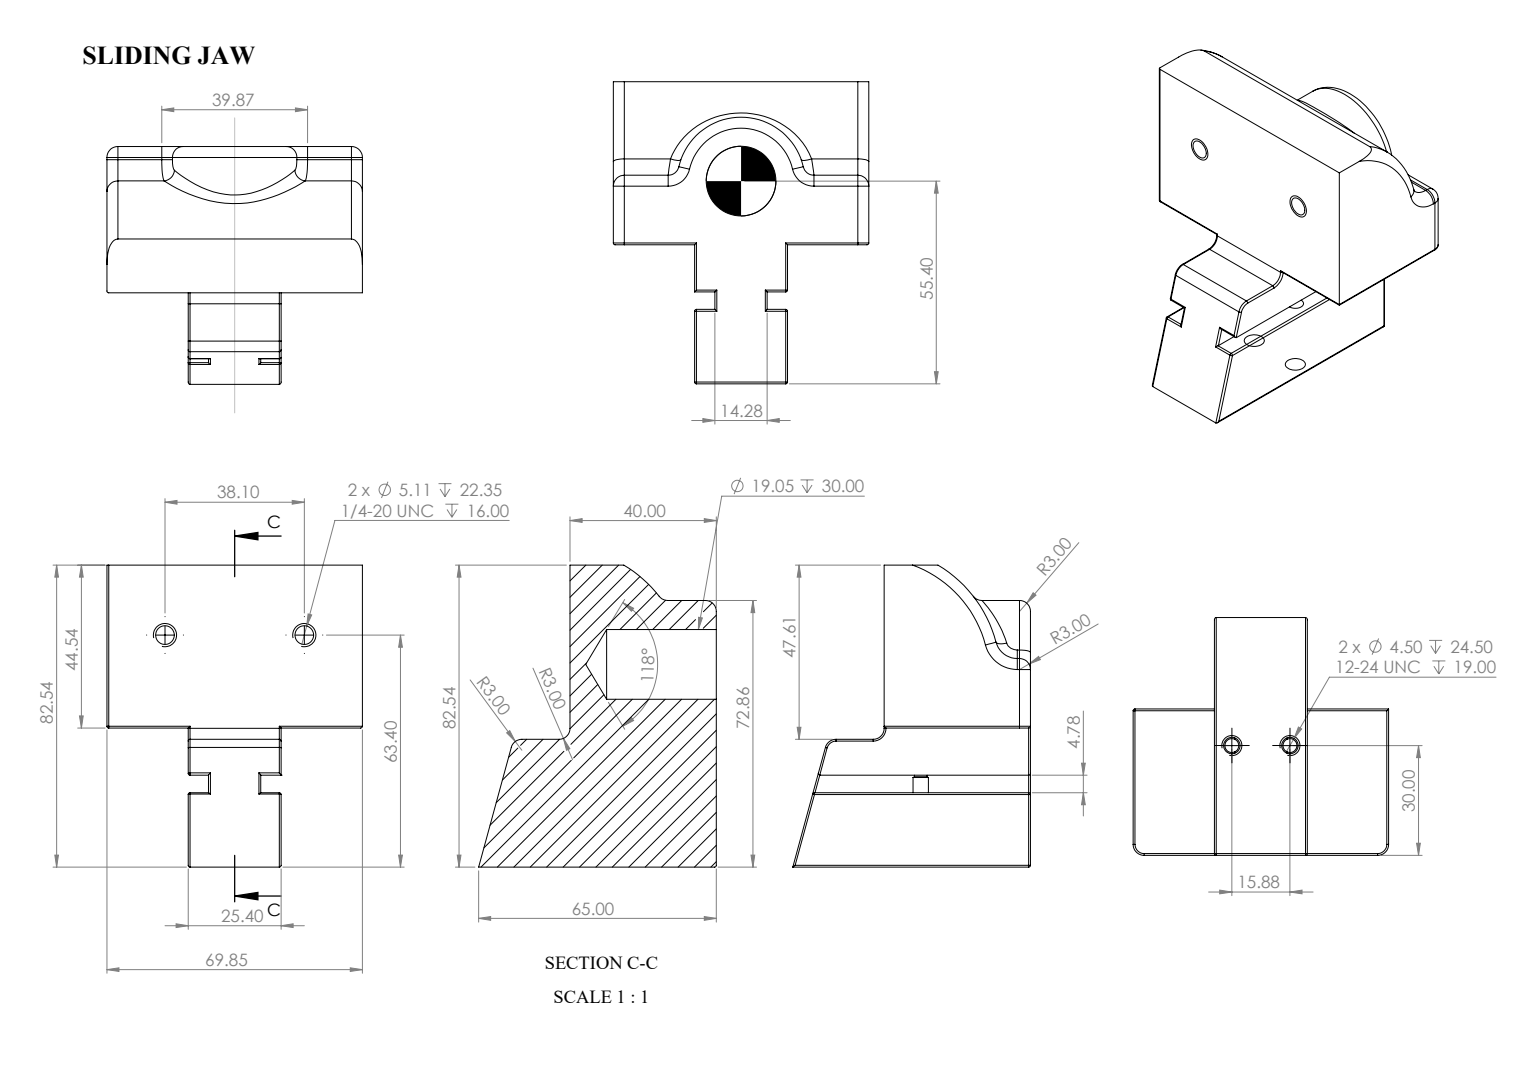
ISO-10303-21;
HEADER;
FILE_DESCRIPTION (('STEP AP214'),
    '1' );
FILE_NAME ('1.1 Sliding Jaw.step',
    '2026-10-06T08:51:13',
    ( '' ),
    ( '' ),
    'SwSTEP 2.0',
    'SolidWorks 2021',
    '' );
FILE_SCHEMA (( 'AUTOMOTIVE_DESIGN' ));
ENDSEC;

DATA;
#14=COLOUR_RGB ( '', 0.08235294, 0.09019608, 0.10196078) ;
#59=CARTESIAN_POINT ( 'NONE',  ( -12.69999999999999929, -60.26999999999998892, -39.50000000000000000 ) ) ;
#66=FILL_AREA_STYLE ('',( #56690 ) ) ;
#140=ORIENTED_EDGE ( 'NONE', *, *, #3276, .F. ) ;
#150=DIRECTION ( 'NONE',  ( 0.000000000000000000, -0.9647414015272155474, 0.2631995976047525887 ) ) ;
#175=ORIENTED_EDGE ( 'NONE', *, *, #80806, .F. ) ;
#177=EDGE_CURVE ( 'NONE', #92630, #88659, #70457, .T. ) ;
#207=ORIENTED_EDGE ( 'NONE', *, *, #61881, .T. ) ;
#237=VERTEX_POINT ( 'NONE', #52898 ) ;
#261=PRESENTATION_STYLE_ASSIGNMENT (( #47937 ) ) ;
#311=ORIENTED_EDGE ( 'NONE', *, *, #103224, .T. ) ;
#327=DIRECTION ( 'NONE',  ( -1.000000000000000000, -2.891205793294679312E-16, 0.000000000000000000 ) ) ;
#402=CARTESIAN_POINT ( 'NONE',  ( -16.92402963342697220, -0.5732982342275830812, -34.79992920313960525 ) ) ;
#422=FILL_AREA_STYLE ('',( #141288 ) ) ;
#437=EDGE_CURVE ( 'NONE', #128814, #125503, #6074, .T. ) ;
#500=EDGE_CURVE ( 'NONE', #83224, #56577, #120555, .T. ) ;
#523=CARTESIAN_POINT ( 'NONE',  ( 0.000000000000000000, -40.42999999999999261, -39.50000000000000000 ) ) ;
#561=SURFACE_STYLE_FILL_AREA ( #32509 ) ;
#640=CARTESIAN_POINT ( 'NONE',  ( 19.04500000000000881, 3.130000000000007887, -22.35000000000000142 ) ) ;
#662=ORIENTED_EDGE ( 'NONE', *, *, #138768, .T. ) ;
#675=DIRECTION ( 'NONE',  ( 1.000000000000000000, -1.248002500702738701E-15, 3.404785525682858480E-16 ) ) ;
#735=ORIENTED_EDGE ( 'NONE', *, *, #48279, .T. ) ;
#744=ORIENTED_EDGE ( 'NONE', *, *, #46623, .T. ) ;
#797=DIRECTION ( 'NONE',  ( 0.000000000000000000, 0.000000000000000000, -1.000000000000000000 ) ) ;
#818=PRESENTATION_STYLE_ASSIGNMENT (( #100864 ) ) ;
#821=ORIENTED_EDGE ( 'NONE', *, *, #120338, .F. ) ;
#853=CARTESIAN_POINT ( 'NONE',  ( 18.91358171146897860, 2.162374846302510090, -30.33482670853117114 ) ) ;
#858=STYLED_ITEM ( 'NONE', ( #106410 ), #103236 ) ;
#859=( NAMED_UNIT ( * ) SI_UNIT ( $, .STERADIAN. ) SOLID_ANGLE_UNIT ( ) );
#864=CARTESIAN_POINT ( 'NONE',  ( -19.05499999999999972, 3.130000000000007887, -23.88381690219165776 ) ) ;
#865=DIRECTION ( 'NONE',  ( 0.000000000000000000, 1.000000000000000000, 0.000000000000000000 ) ) ;
#878=VERTEX_POINT ( 'NONE', #7356 ) ;
#915=ORIENTED_EDGE ( 'NONE', *, *, #126095, .T. ) ;
#982=CARTESIAN_POINT ( 'NONE',  ( -19.05499999999999261, 3.130000000000007887, -22.35000000000000142 ) ) ;
#1021=LINE ( 'NONE', #64172, #109457 ) ;
#1027=CARTESIAN_POINT ( 'NONE',  ( 34.92500000000001847, -3.269999999999991580, -36.39086428169088094 ) ) ;
#1062=CIRCLE ( 'NONE', #24171, 9.524999999999991473 ) ;
#1094=ORIENTED_EDGE ( 'NONE', *, *, #50202, .T. ) ;
#1098=EDGE_CURVE ( 'NONE', #125503, #115328, #46246, .T. ) ;
#1116=SURFACE_STYLE_FILL_AREA ( #111312 ) ;
#1187=DIRECTION ( 'NONE',  ( 0.000000000000000000, 0.000000000000000000, -1.000000000000000000 ) ) ;
#1205=UNCERTAINTY_MEASURE_WITH_UNIT (LENGTH_MEASURE( 1.000000000000000082E-05 ), #112057, 'distance_accuracy_value', 'NONE');
#1216=CARTESIAN_POINT ( 'NONE',  ( 19.61406247417281890, -0.8217383486644460611, -31.54407713966740090 ) ) ;
#1223=EDGE_CURVE ( 'NONE', #56577, #75784, #81427, .T. ) ;
#1228=UNCERTAINTY_MEASURE_WITH_UNIT (LENGTH_MEASURE( 1.000000000000000082E-05 ), #8180, 'distance_accuracy_value', 'NONE');
#1271=ORIENTED_EDGE ( 'NONE', *, *, #28429, .T. ) ;
#1342=FACE_OUTER_BOUND ( 'NONE', #53273, .T. ) ;
#1423=CARTESIAN_POINT ( 'NONE',  ( 19.93618820137057668, -0.2700000000508058218, -40.00000000000000000 ) ) ;
#1560=FILL_AREA_STYLE_COLOUR ( '', #46155 ) ;
#1583=DIRECTION ( 'NONE',  ( 1.000000000000000000, 0.000000000000000000, 0.000000000000000000 ) ) ;
#1608=VECTOR ( 'NONE', #22294, 1000.000000000000000 ) ;
#1684=ORIENTED_EDGE ( 'NONE', *, *, #62219, .F. ) ;
#1758=CARTESIAN_POINT ( 'NONE',  ( 7.940000000000001279, -35.14999999999999858, -10.00000000000000178 ) ) ;
#1775=CARTESIAN_POINT ( 'NONE',  ( 12.19999999999999574, -25.83999999999997499, -40.00000000000000711 ) ) ;
#1800=VERTEX_POINT ( 'NONE', #105620 ) ;
#1802=CARTESIAN_POINT ( 'NONE',  ( -17.54957349249705345, -3.270000000000005347, -36.39086428169088094 ) ) ;
#1884=CARTESIAN_POINT ( 'NONE',  ( -32.59703385998916758, 22.27000000000000668, -14.57157165008255006 ) ) ;
#1899=DIRECTION ( 'NONE',  ( -1.000000000000000000, -0.000000000000000000, -0.000000000000000000 ) ) ;
#1905=( NAMED_UNIT ( * ) SI_UNIT ( $, .STERADIAN. ) SOLID_ANGLE_UNIT ( ) );
#1907=COLOUR_RGB ( '', 0.31764706, 0.68627451, 0.89019608) ;
#1970=EDGE_CURVE ( 'NONE', #119435, #81122, #129068, .T. ) ;
#1980=ORIENTED_EDGE ( 'NONE', *, *, #31379, .F. ) ;
#2139=CIRCLE ( 'NONE', #83211, 9.000000000000001776 ) ;
#2174=LINE ( 'NONE', #122554, #93845 ) ;
#2207=( NAMED_UNIT ( * ) SI_UNIT ( $, .STERADIAN. ) SOLID_ANGLE_UNIT ( ) );
#2256=CARTESIAN_POINT ( 'NONE',  ( -6.640000000000001457, -40.42999999999999261, -40.00000000000000000 ) ) ;
#2267=CARTESIAN_POINT ( 'NONE',  ( 12.56294698093633500, 9.782926692783094680, -27.04452493197952734 ) ) ;
#2273=ORIENTED_EDGE ( 'NONE', *, *, #3238, .F. ) ;
#2279=DIRECTION ( 'NONE',  ( -1.000000000000000000, 0.000000000000000000, 0.000000000000000000 ) ) ;
#2290=VECTOR ( 'NONE', #11080, 1000.000000000000000 ) ;
#2342=EDGE_LOOP ( 'NONE', ( #132806, #114622, #99029, #81008 ) ) ;
#2362=CARTESIAN_POINT ( 'NONE',  ( 33.16642969376915318, 22.27000000000001023, -14.18759795118478806 ) ) ;
#2383=ADVANCED_FACE ( 'NONE', ( #22714 ), #26494, .F. ) ;
#2395=( NAMED_UNIT ( * ) SI_UNIT ( $, .STERADIAN. ) SOLID_ANGLE_UNIT ( ) );
#2401=VERTEX_POINT ( 'NONE', #112622 ) ;
#2418=CARTESIAN_POINT ( 'NONE',  ( -7.940000000000001279, -35.14999999999999147, -11.89864999999999640 ) ) ;
#2443=LINE ( 'NONE', #24925, #33137 ) ;
#2479=ORIENTED_EDGE ( 'NONE', *, *, #17002, .F. ) ;
#2537=CARTESIAN_POINT ( 'NONE',  ( -17.15351703751440482, -1.296283446796709926, -31.89465879581624819 ) ) ;
#2598=ORIENTED_EDGE ( 'NONE', *, *, #29243, .F. ) ;
#2608=AXIS2_PLACEMENT_3D ( 'NONE', #21342, #132276, #123538 ) ;
#2651=( NAMED_UNIT ( * ) PLANE_ANGLE_UNIT ( ) SI_UNIT ( $, .RADIAN. ) );
#2664=UNCERTAINTY_MEASURE_WITH_UNIT (LENGTH_MEASURE( 1.000000000000000082E-05 ), #86950, 'distance_accuracy_value', 'NONE');
#2723=MECHANICAL_DESIGN_GEOMETRIC_PRESENTATION_REPRESENTATION('',(#65265),#107034);
#2737=ORIENTED_EDGE ( 'NONE', *, *, #52281, .F. ) ;
#2907=VERTEX_POINT ( 'NONE', #4607 ) ;
#2931=VECTOR ( 'NONE', #119304, 1000.000000000000000 ) ;
#3000=CARTESIAN_POINT ( 'NONE',  ( 12.19999999999999574, -34.51840020119763608, 17.97447928118983640 ) ) ;
#3003=CARTESIAN_POINT ( 'NONE',  ( -34.92499999999999005, -3.270000000000013340, -37.00000000000000000 ) ) ;
#3025=LINE ( 'NONE', #37086, #65102 ) ;
#3124=FILL_AREA_STYLE_COLOUR ( '', #104610 ) ;
#3150=CARTESIAN_POINT ( 'NONE',  ( 14.92996780037367799, 4.193323835446171266, -32.27671736793806900 ) ) ;
#3170=LINE ( 'NONE', #103201, #143489 ) ;
#3238=EDGE_CURVE ( 'NONE', #120537, #2401, #79273, .T. ) ;
#3248=DIRECTION ( 'NONE',  ( -1.000000000000000000, 1.451651444332056451E-15, 0.000000000000000000 ) ) ;
#3263=CARTESIAN_POINT ( 'NONE',  ( -16.45742106731621845, 0.9613713492673543470, -33.49048331797055766 ) ) ;
#3264=ORIENTED_EDGE ( 'NONE', *, *, #77395, .F. ) ;
#3276=EDGE_CURVE ( 'NONE', #6439, #25909, #5535, .T. ) ;
#3312=CARTESIAN_POINT ( 'NONE',  ( -7.940000000000001279, -33.26999999999999602, -8.101350000000008933 ) ) ;
#3341=EDGE_CURVE ( 'NONE', #71785, #109962, #90838, .T. ) ;
#3362=DIRECTION ( 'NONE',  ( 1.400468248933915008E-15, 0.9647414015272156584, -0.2631995976047526442 ) ) ;
#3417=ADVANCED_FACE ( 'NONE', ( #84929 ), #71949, .T. ) ;
#3421=DIRECTION ( 'NONE',  ( 0.000000000000000000, -0.2631995976047557528, -0.9647414015272147703 ) ) ;
#3497=ORIENTED_EDGE ( 'NONE', *, *, #39825, .F. ) ;
#3510=CARTESIAN_POINT ( 'NONE',  ( 12.69999999999999574, -34.65000000000001279, 17.49210858042622618 ) ) ;
#3521=DIRECTION ( 'NONE',  ( -1.000000000000000000, 0.000000000000000000, 0.000000000000000000 ) ) ;
#3531=VERTEX_POINT ( 'NONE', #10209 ) ;
#3602=FILL_AREA_STYLE_COLOUR ( '', #53782 ) ;
#3652=DIRECTION ( 'NONE',  ( -1.000000000000000000, 0.000000000000000000, 0.000000000000000000 ) ) ;
#3698=DIRECTION ( 'NONE',  ( -2.891205793294675861E-16, 1.000000000000000000, 0.000000000000000000 ) ) ;
#3718=CARTESIAN_POINT ( 'NONE',  ( 7.939999999999994174, -60.26999999999998892, -12.24790000000000134 ) ) ;
#3723=DIRECTION ( 'NONE',  ( 1.000000000000000000, 0.000000000000000000, 0.000000000000000000 ) ) ;
#3756=CARTESIAN_POINT ( 'NONE',  ( 12.69999999999999574, -25.83999999999998565, 13.17925390838733968 ) ) ;
#3757=CARTESIAN_POINT ( 'NONE',  ( -7.140000000000001457, 0.000000000000000000, -40.00000000000000000 ) ) ;
#3786=PRESENTATION_STYLE_ASSIGNMENT (( #58989 ) ) ;
#3795=CIRCLE ( 'NONE', #82606, 2.247899999999998677 ) ;
#3799=FACE_OUTER_BOUND ( 'NONE', #140007, .T. ) ;
#3816=VECTOR ( 'NONE', #59667, 1000.000000000000000 ) ;
#3839=DIRECTION ( 'NONE',  ( 1.000000000000000000, 0.000000000000000000, 0.000000000000000000 ) ) ;
#3861=VECTOR ( 'NONE', #102788, 1000.000000000000000 ) ;
#3883=SURFACE_SIDE_STYLE ('',( #14805 ) ) ;
#3941=SURFACE_SIDE_STYLE ('',( #68571 ) ) ;
#3983=CARTESIAN_POINT ( 'NONE',  ( -19.28515664589288647, 1.196650378695323758, -30.59010235425024860 ) ) ;
#3999=DIRECTION ( 'NONE',  ( 0.000000000000000000, 0.000000000000000000, -1.000000000000000000 ) ) ;
#4035=CARTESIAN_POINT ( 'NONE',  ( 16.85424587240084904, -0.3099398835762542936, -34.40694344753310929 ) ) ;
#4092=DIRECTION ( 'NONE',  ( -0.000000000000000000, -1.000000000000000000, -0.000000000000000000 ) ) ;
#4129=DIRECTION ( 'NONE',  ( -1.000000000000000000, 0.000000000000000000, 0.000000000000000000 ) ) ;
#4192=VERTEX_POINT ( 'NONE', #140280 ) ;
#4219=LINE ( 'NONE', #47843, #99999 ) ;
#4226=ORIENTED_EDGE ( 'NONE', *, *, #50412, .F. ) ;
#4280=EDGE_CURVE ( 'NONE', #87140, #131250, #73496, .T. ) ;
#4283=ORIENTED_EDGE ( 'NONE', *, *, #28653, .T. ) ;
#4300=ORIENTED_EDGE ( 'NONE', *, *, #110869, .F. ) ;
#4317=( NAMED_UNIT ( * ) SI_UNIT ( $, .STERADIAN. ) SOLID_ANGLE_UNIT ( ) );
#4374=CARTESIAN_POINT ( 'NONE',  ( -18.46799460936313864, 3.072550929180732471, -30.05020605058495065 ) ) ;
#4385=DIRECTION ( 'NONE',  ( 0.000000000000000000, 0.9647414015272156584, -0.2631995976047526442 ) ) ;
#4393=DIRECTION ( 'NONE',  ( 1.000000000000000000, 0.000000000000000000, 0.000000000000000000 ) ) ;
#4472=CIRCLE ( 'NONE', #64785, 2.247899999999995568 ) ;
#4482=ORIENTED_EDGE ( 'NONE', *, *, #105415, .F. ) ;
#4493=ORIENTED_EDGE ( 'NONE', *, *, #112721, .T. ) ;
#4502=ORIENTED_EDGE ( 'NONE', *, *, #56252, .F. ) ;
#4530=DIRECTION ( 'NONE',  ( 0.000000000000000000, 1.000000000000000000, 0.000000000000000000 ) ) ;
#4537=VECTOR ( 'NONE', #106112, 999.9999999999998863 ) ;
#4540=AXIS2_PLACEMENT_3D ( 'NONE', #69357, #125137, #25826 ) ;
#4607=CARTESIAN_POINT ( 'NONE',  ( -7.140000000000001457, -39.92999999999999261, 18.93259187797432475 ) ) ;
#4616=DIRECTION ( 'NONE',  ( 0.9743982503113673976, -0.2248289345038710085, 0.000000000000000000 ) ) ;
#4668=STYLED_ITEM ( 'NONE', ( #17992 ), #48749 ) ;
#4697=CARTESIAN_POINT ( 'NONE',  ( -13.89419556063288397, 5.740820235442677166, -29.07950590408880132 ) ) ;
#4708=CARTESIAN_POINT ( 'NONE',  ( -7.940000000000001279, -35.14999999999999147, -10.00000000000000178 ) ) ;
#4731=CARTESIAN_POINT ( 'NONE',  ( -34.36724870009786059, 22.27000000000001023, -12.13301201282878772 ) ) ;
#4745=CIRCLE ( 'NONE', #11710, 3.499999999999999556 ) ;
#4769=AXIS2_PLACEMENT_3D ( 'NONE', #25165, #24459, #89036 ) ;
#4819=CARTESIAN_POINT ( 'NONE',  ( -19.93618820137057668, -0.2700000000508183118, -40.00000000000000000 ) ) ;
#4829=DIRECTION ( 'NONE',  ( -1.000000000000000000, 0.000000000000000000, 0.000000000000000000 ) ) ;
#4913=DIRECTION ( 'NONE',  ( 1.000000000000000000, 0.000000000000000000, 0.000000000000000000 ) ) ;
#4964=CONICAL_SURFACE ( 'NONE', #32766, 1.898649999999993065, 1.029744258676648316 ) ;
#4984=STYLED_ITEM ( 'NONE', ( #104537 ), #141940 ) ;
#5055=CONICAL_SURFACE ( 'NONE', #67642, 2.247899999999995568, 1.029744258676650315 ) ;
#5131=CARTESIAN_POINT ( 'NONE',  ( 34.92500000000001847, 2.730000000000007976, -36.39086428169088094 ) ) ;
#5154=AXIS2_PLACEMENT_3D ( 'NONE', #122356, #67304, #78180 ) ;
#5164=CARTESIAN_POINT ( 'NONE',  ( 0.000000000000000000, -34.64999999999999147, -39.50000000000000000 ) ) ;
#5190=( NAMED_UNIT ( * ) SI_UNIT ( $, .STERADIAN. ) SOLID_ANGLE_UNIT ( ) );
#5201=FACE_OUTER_BOUND ( 'NONE', #50065, .T. ) ;
#5225=COLOUR_RGB ( '', 0.08235294, 0.09019608, 0.10196078) ;
#5267=ORIENTED_EDGE ( 'NONE', *, *, #73471, .T. ) ;
#5302=CARTESIAN_POINT ( 'NONE',  ( 34.92500000000002558, -21.76999999999999247, -37.00000000000000000 ) ) ;
#5314=B_SPLINE_CURVE_WITH_KNOTS ( 'NONE', 3,
 ( #95896, #85018, #8149, #54562, #98739, #142285, #52387, #141559, #41508, #76305 ),
 .UNSPECIFIED., .F., .F.,
 ( 4, 2, 2, 2, 4 ),
 ( 2.602085213965210642E-18, 0.001968391616361199817, 0.003936783232722403103, 0.005905174849083606389, 0.007873566465444809676 ),
 .UNSPECIFIED. ) ;
#5336=EDGE_CURVE ( 'NONE', #103352, #23962, #99221, .T. ) ;
#5383=ORIENTED_EDGE ( 'NONE', *, *, #86397, .F. ) ;
#5444=CARTESIAN_POINT ( 'NONE',  ( -11.11660040884707357, 10.72905655457496543, -26.47562522530603957 ) ) ;
#5446=DIRECTION ( 'NONE',  ( 0.000000000000000000, -1.387778780781446464E-15, 1.000000000000000000 ) ) ;
#5489=UNCERTAINTY_MEASURE_WITH_UNIT (LENGTH_MEASURE( 1.000000000000000082E-05 ), #69508, 'distance_accuracy_value', 'NONE');
#5512=ORIENTED_EDGE ( 'NONE', *, *, #26066, .T. ) ;
#5535=CIRCLE ( 'NONE', #102847, 0.5000000000000004441 ) ;
#5582=DIRECTION ( 'NONE',  ( -0.000000000000000000, -1.000000000000000000, -0.000000000000000000 ) ) ;
#5680=UNCERTAINTY_MEASURE_WITH_UNIT (LENGTH_MEASURE( 1.000000000000000082E-05 ), #58105, 'distance_accuracy_value', 'NONE');
#5683=CARTESIAN_POINT ( 'NONE',  ( 16.49230000000001439, 3.130000000000008331, -22.35000000000000142 ) ) ;
#5689=SURFACE_SIDE_STYLE ('',( #62255 ) ) ;
#5700=SURFACE_STYLE_FILL_AREA ( #105035 ) ;
#5749=SHAPE_REPRESENTATION_RELATIONSHIP ( 'NONE' , 'NONE' ,  #88538, #11968 ) ;
#5841=CARTESIAN_POINT ( 'NONE',  ( -10.91502770842411785, 10.86848332146160168, -26.39372705248169027 ) ) ;
#5955=( LENGTH_UNIT ( ) NAMED_UNIT ( * ) SI_UNIT ( .MILLI., .METRE. ) );
#6049=CARTESIAN_POINT ( 'NONE',  ( 7.139999999999991687, -35.69931938766895740, -8.025146269613541605 ) ) ;
#6069=CARTESIAN_POINT ( 'NONE',  ( -16.64463492972600633, 0.4092709014657676114, -33.72289106502642397 ) ) ;
#6074=LINE ( 'NONE', #28606, #4537 ) ;
#6099=EDGE_CURVE ( 'NONE', #40406, #27902, #137847, .T. ) ;
#6100=DIRECTION ( 'NONE',  ( 0.000000000000000000, -0.9647414015272149923, 0.2631995976047557528 ) ) ;
#6106=ORIENTED_EDGE ( 'NONE', *, *, #44004, .T. ) ;
#6127=EDGE_CURVE ( 'NONE', #17782, #4192, #2174, .T. ) ;
#6141=AXIS2_PLACEMENT_3D ( 'NONE', #137176, #68375, #93668 ) ;
#6143=CARTESIAN_POINT ( 'NONE',  ( -15.35539145651694781, 3.520240452094296923, -29.92141252516384142 ) ) ;
#6261=EDGE_CURVE ( 'NONE', #88226, #134318, #142405, .T. ) ;
#6264=VECTOR ( 'NONE', #121697, 1000.000000000000000 ) ;
#6325=FACE_OUTER_BOUND ( 'NONE', #85481, .T. ) ;
#6350=PRESENTATION_STYLE_ASSIGNMENT (( #7812 ) ) ;
#6364=LINE ( 'NONE', #48499, #141521 ) ;
#6384=SURFACE_STYLE_USAGE ( .BOTH. , #49966 ) ;
#6439=VERTEX_POINT ( 'NONE', #70256 ) ;
#6463=SURFACE_STYLE_FILL_AREA ( #65214 ) ;
#6482=SURFACE_STYLE_USAGE ( .BOTH. , #83396 ) ;
#6515=DIRECTION ( 'NONE',  ( 0.000000000000000000, -0.9647414015272155474, 0.2631995976047525887 ) ) ;
#6522=CARTESIAN_POINT ( 'NONE',  ( -7.940000000000001279, -35.14999999999999147, -10.00000000000000178 ) ) ;
#6536=VECTOR ( 'NONE', #97245, 1000.000000000000000 ) ;
#6617=FACE_OUTER_BOUND ( 'NONE', #82475, .T. ) ;
#6654=CARTESIAN_POINT ( 'NONE',  ( 31.92500000000002203, -22.26999999999999247, -39.50000000000000000 ) ) ;
#6664=ORIENTED_EDGE ( 'NONE', *, *, #95843, .T. ) ;
#6669=( GEOMETRIC_REPRESENTATION_CONTEXT ( 3 ) GLOBAL_UNCERTAINTY_ASSIGNED_CONTEXT ( ( #1228 ) ) GLOBAL_UNIT_ASSIGNED_CONTEXT ( ( #8180, #51740, #52420 ) ) REPRESENTATION_CONTEXT ( 'NONE', 'WORKASPACE' ) );
#6729=ORIENTED_EDGE ( 'NONE', *, *, #89457, .T. ) ;
#6789=ORIENTED_EDGE ( 'NONE', *, *, #51613, .T. ) ;
#6790=SURFACE_STYLE_USAGE ( .BOTH. , #41604 ) ;
#6801=SURFACE_SIDE_STYLE ('',( #72151 ) ) ;
#6828=CARTESIAN_POINT ( 'NONE',  ( 12.69999999999999574, -60.26999999999998892, -39.50000000000000000 ) ) ;
#6838=AXIS2_PLACEMENT_3D ( 'NONE', #22591, #66861, #111031 ) ;
#6852=MECHANICAL_DESIGN_GEOMETRIC_PRESENTATION_REPRESENTATION('',(#134096),#141099);
#6856=CARTESIAN_POINT ( 'NONE',  ( -16.03282571951856283, 6.618735317068870749, -28.66949109531741158 ) ) ;
#6861=CIRCLE ( 'NONE', #87938, 3.000000000000000000 ) ;
#6908=CARTESIAN_POINT ( 'NONE',  ( 17.54601624070869548, -3.246904730846185583, -35.78195362552649783 ) ) ;
#6912=ORIENTED_EDGE ( 'NONE', *, *, #121789, .T. ) ;
#6929=CARTESIAN_POINT ( 'NONE',  ( 21.59770000000000323, 3.130000000000007887, -22.35000000000000142 ) ) ;
#6940=LINE ( 'NONE', #30161, #2931 ) ;
#6948=DIRECTION ( 'NONE',  ( 0.000000000000000000, -0.000000000000000000, 1.000000000000000000 ) ) ;
#6966=EDGE_CURVE ( 'NONE', #126576, #120537, #90574, .T. ) ;
#7035=ORIENTED_EDGE ( 'NONE', *, *, #22890, .F. ) ;
#7066=CARTESIAN_POINT ( 'NONE',  ( -12.49289321881345494, -22.06289321881344634, -1.793453714559299607E-17 ) ) ;
#7073=FACE_OUTER_BOUND ( 'NONE', #99253, .T. ) ;
#7087=FACE_OUTER_BOUND ( 'NONE', #54296, .T. ) ;
#7131=ORIENTED_EDGE ( 'NONE', *, *, #67255, .T. ) ;
#7146=ORIENTED_EDGE ( 'NONE', *, *, #68056, .T. ) ;
#7236=CARTESIAN_POINT ( 'NONE',  ( 7.122370700763592133, -39.92999999999999972, 19.06900128115122328 ) ) ;
#7283=DIRECTION ( 'NONE',  ( 0.000000000000000000, -1.000000000000000000, 0.000000000000000000 ) ) ;
#7302=CONICAL_SURFACE ( 'NONE', #11972, 2.247899999999995568, 1.029744258676650315 ) ;
#7336=SURFACE_SIDE_STYLE ('',( #118970 ) ) ;
#7356=CARTESIAN_POINT ( 'NONE',  ( -7.940000000000007496, -60.26999999999998892, -12.24790000000000312 ) ) ;
#7376=CARTESIAN_POINT ( 'NONE',  ( 34.42500000000002558, -22.26999999999999247, -0.5000000000000000000 ) ) ;
#7388=ADVANCED_FACE ( 'NONE', ( #117207 ), #50553, .F. ) ;
#7451=LINE ( 'NONE', #142981, #124684 ) ;
#7456=LINE ( 'NONE', #129981, #14319 ) ;
#7478=( GEOMETRIC_REPRESENTATION_CONTEXT ( 3 ) GLOBAL_UNCERTAINTY_ASSIGNED_CONTEXT ( ( #130361 ) ) GLOBAL_UNIT_ASSIGNED_CONTEXT ( ( #90232, #54777, #33049 ) ) REPRESENTATION_CONTEXT ( 'NONE', 'WORKASPACE' ) );
#7546=ORIENTED_EDGE ( 'NONE', *, *, #63364, .F. ) ;
#7572=ADVANCED_FACE ( 'NONE', ( #130989 ), #33131, .T. ) ;
#7590=ORIENTED_EDGE ( 'NONE', *, *, #57217, .T. ) ;
#7594=CARTESIAN_POINT ( 'NONE',  ( 13.55929415207057076, 9.045080515339410709, -27.46719384617228243 ) ) ;
#7609=PRODUCT ( '1.1 Sliding Jaw', '1.1 Sliding Jaw', '', ( #61303 ) ) ;
#7648=ORIENTED_EDGE ( 'NONE', *, *, #120810, .T. ) ;
#7667=DIRECTION ( 'NONE',  ( -3.166071393695993333E-32, 1.016133275908817741E-16, -1.000000000000000000 ) ) ;
#7698=DIRECTION ( 'NONE',  ( 1.000000000000000000, 0.000000000000000000, 0.000000000000000000 ) ) ;
#7812=SURFACE_STYLE_USAGE ( .BOTH. , #139074 ) ;
#7843=EDGE_CURVE ( 'NONE', #64319, #22146, #125819, .T. ) ;
#7888=ORIENTED_EDGE ( 'NONE', *, *, #106156, .T. ) ;
#7896=( LENGTH_UNIT ( ) NAMED_UNIT ( * ) SI_UNIT ( .MILLI., .METRE. ) );
#7902=ORIENTED_EDGE ( 'NONE', *, *, #35649, .T. ) ;
#7905=( NAMED_UNIT ( * ) PLANE_ANGLE_UNIT ( ) SI_UNIT ( $, .RADIAN. ) );
#7919=CARTESIAN_POINT ( 'NONE',  ( 7.939999999999994174, -60.26999999999998892, -12.24789999999999957 ) ) ;
#7921=CARTESIAN_POINT ( 'NONE',  ( 19.61884355727922014, -0.8539424794488987835, -31.56759919030367101 ) ) ;
#7925=VERTEX_POINT ( 'NONE', #85860 ) ;
#7936=CARTESIAN_POINT ( 'NONE',  ( -9.524999999999995026, -4.870000000000014317, -40.00000000000000000 ) ) ;
#7941=STYLED_ITEM ( 'NONE', ( #13280 ), #2383 ) ;
#7960=FACE_OUTER_BOUND ( 'NONE', #132463, .T. ) ;
#7987=ORIENTED_EDGE ( 'NONE', *, *, #1098, .F. ) ;
#8028=CARTESIAN_POINT ( 'NONE',  ( -3.753437965960260136, 12.18814048229829261, -27.09591142044626011 ) ) ;
#8029=CARTESIAN_POINT ( 'NONE',  ( -6.684521246590537480, -34.56135169103111338, 17.98619725537731995 ) ) ;
#8045=( GEOMETRIC_REPRESENTATION_CONTEXT ( 3 ) GLOBAL_UNCERTAINTY_ASSIGNED_CONTEXT ( ( #105876 ) ) GLOBAL_UNIT_ASSIGNED_CONTEXT ( ( #104927, #115764, #17884 ) ) REPRESENTATION_CONTEXT ( 'NONE', 'WORKASPACE' ) );
#8051=( LENGTH_UNIT ( ) NAMED_UNIT ( * ) SI_UNIT ( .MILLI., .METRE. ) );
#8102=ORIENTED_EDGE ( 'NONE', *, *, #500, .T. ) ;
#8149=CARTESIAN_POINT ( 'NONE',  ( -19.49368896717581023, -0.02969617003380616710, -31.02254237922252500 ) ) ;
#8158=FACE_OUTER_BOUND ( 'NONE', #136308, .T. ) ;
#8162=DIRECTION ( 'NONE',  ( -0.000000000000000000, -1.000000000000000000, -0.000000000000000000 ) ) ;
#8163=CARTESIAN_POINT ( 'NONE',  ( 12.69999999999999574, -35.15000000000000568, -40.00000000000000000 ) ) ;
#8164=DIRECTION ( 'NONE',  ( -1.000000000000000000, -0.000000000000000000, -0.000000000000000000 ) ) ;
#8180=( LENGTH_UNIT ( ) NAMED_UNIT ( * ) SI_UNIT ( .MILLI., .METRE. ) );
#8257=EDGE_CURVE ( 'NONE', #63984, #124237, #110663, .T. ) ;
#8291=CARTESIAN_POINT ( 'NONE',  ( -4.595688708094440855, 11.98067335678676670, -27.27784815589622980 ) ) ;
#8402=AXIS2_PLACEMENT_3D ( 'NONE', #98352, #87474, #129520 ) ;
#8417=AXIS2_PLACEMENT_3D ( 'NONE', #44307, #141459, #63907 ) ;
#8418=EDGE_CURVE ( 'NONE', #79752, #126576, #128219, .T. ) ;
#8466=ORIENTED_EDGE ( 'NONE', *, *, #112375, .F. ) ;
#8520=DIRECTION ( 'NONE',  ( 0.000000000000000000, 0.000000000000000000, -1.000000000000000000 ) ) ;
#8534=( NAMED_UNIT ( * ) SI_UNIT ( $, .STERADIAN. ) SOLID_ANGLE_UNIT ( ) );
#8547=CARTESIAN_POINT ( 'NONE',  ( -55.65468426143998215, -25.33999999999998565, 0.000000000000000000 ) ) ;
#8557=AXIS2_PLACEMENT_3D ( 'NONE', #104149, #4092, #49116 ) ;
#8646=FACE_OUTER_BOUND ( 'NONE', #139703, .T. ) ;
#8791=SURFACE_SIDE_STYLE ('',( #63277 ) ) ;
#8833=STYLED_ITEM ( 'NONE', ( #98753 ), #57613 ) ;
#8846=DIRECTION ( 'NONE',  ( 0.000000000000000000, 1.000000000000000000, 0.000000000000000000 ) ) ;
#8891=ORIENTED_EDGE ( 'NONE', *, *, #49728, .F. ) ;
#8925=CARTESIAN_POINT ( 'NONE',  ( 0.000000000000000000, 0.000000000000000000, 0.000000000000000000 ) ) ;
#8938=EDGE_CURVE ( 'NONE', #4192, #28467, #21801, .T. ) ;
#8949=FILL_AREA_STYLE ('',( #17712 ) ) ;
#8984=CARTESIAN_POINT ( 'NONE',  ( 0.4527155423044956772, 12.59110042198609136, -25.26827755431022027 ) ) ;
#8998=ORIENTED_EDGE ( 'NONE', *, *, #117477, .T. ) ;
#9007=( LENGTH_UNIT ( ) NAMED_UNIT ( * ) SI_UNIT ( .MILLI., .METRE. ) );
#9044=AXIS2_PLACEMENT_3D ( 'NONE', #41542, #107522, #16954 ) ;
#9045=CIRCLE ( 'NONE', #129535, 2.999999999999999112 ) ;
#9071=CARTESIAN_POINT ( 'NONE',  ( -12.70000000000000462, -25.83999999999997499, -40.00000000000000711 ) ) ;
#9084=EDGE_CURVE ( 'NONE', #111777, #118671, #55247, .T. ) ;
#9102=ORIENTED_EDGE ( 'NONE', *, *, #57276, .T. ) ;
#9177=ORIENTED_EDGE ( 'NONE', *, *, #105365, .T. ) ;
#9194=EDGE_LOOP ( 'NONE', ( #48404, #130165, #120221, #122182, #13890, #72824 ) ) ;
#9225=ORIENTED_EDGE ( 'NONE', *, *, #104797, .F. ) ;
#9269=ORIENTED_EDGE ( 'NONE', *, *, #79857, .T. ) ;
#9298=ORIENTED_EDGE ( 'NONE', *, *, #77651, .T. ) ;
#9300=EDGE_CURVE ( 'NONE', #53394, #80081, #84507, .T. ) ;
#9303=MECHANICAL_DESIGN_GEOMETRIC_PRESENTATION_REPRESENTATION('',(#111157),#23539);
#9347=AXIS2_PLACEMENT_3D ( 'NONE', #68266, #35630, #11658 ) ;
#9369=( LENGTH_UNIT ( ) NAMED_UNIT ( * ) SI_UNIT ( .MILLI., .METRE. ) );
#9370=CARTESIAN_POINT ( 'NONE',  ( 7.134088674951085451, -39.93000000000000682, 19.02448003456068548 ) ) ;
#9397=DIRECTION ( 'NONE',  ( -0.000000000000000000, -0.9647414015272155474, 0.2631995976047525887 ) ) ;
#9398=ORIENTED_EDGE ( 'NONE', *, *, #6099, .F. ) ;
#9431=DIRECTION ( 'NONE',  ( 0.000000000000000000, 0.000000000000000000, 1.000000000000000000 ) ) ;
#9435=MECHANICAL_DESIGN_GEOMETRIC_PRESENTATION_REPRESENTATION('',(#53452),#44272);
#9445=CARTESIAN_POINT ( 'NONE',  ( -0.9818841892814907935, 12.58817548488941540, -26.73591915876452774 ) ) ;
#9494=CIRCLE ( 'NONE', #28058, 34.92999999999999261 ) ;
#9531=CYLINDRICAL_SURFACE ( 'NONE', #29626, 2.999999999999999112 ) ;
#9539=ORIENTED_EDGE ( 'NONE', *, *, #71326, .F. ) ;
#9561=COLOUR_RGB ( '', 0.09019608, 0.27058824, 0.51372549) ;
#9568=DIRECTION ( 'NONE',  ( -1.000000000000000000, 0.000000000000000000, 0.000000000000000000 ) ) ;
#9615=DIRECTION ( 'NONE',  ( -0.000000000000000000, 0.2631995976047526442, 0.9647414015272156584 ) ) ;
#9621=ORIENTED_EDGE ( 'NONE', *, *, #117477, .F. ) ;
#9648=AXIS2_PLACEMENT_3D ( 'NONE', #51640, #95834, #29152 ) ;
#9690=ORIENTED_EDGE ( 'NONE', *, *, #61925, .F. ) ;
#9707=VERTEX_POINT ( 'NONE', #68481 ) ;
#9727=LINE ( 'NONE', #54000, #61169 ) ;
#9741=CARTESIAN_POINT ( 'NONE',  ( -3.453448961350486623, 12.25336827149928176, -25.50699926098112513 ) ) ;
#9743=EDGE_CURVE ( 'NONE', #46696, #40966, #127095, .T. ) ;
#9786=EDGE_CURVE ( 'NONE', #106369, #103352, #59738, .T. ) ;
#9798=DIRECTION ( 'NONE',  ( 1.000000000000000000, 0.000000000000000000, 0.000000000000000000 ) ) ;
#9804=SURFACE_SIDE_STYLE ('',( #107686 ) ) ;
#9854=ORIENTED_EDGE ( 'NONE', *, *, #138768, .F. ) ;
#9868=VERTEX_POINT ( 'NONE', #118356 ) ;
#9871=CARTESIAN_POINT ( 'NONE',  ( 12.19999999999999574, -34.65000000000001279, -40.00000000000000000 ) ) ;
#9896=CIRCLE ( 'NONE', #19226, 0.5000000000000004441 ) ;
#9924=AXIS2_PLACEMENT_3D ( 'NONE', #60888, #40528, #118029 ) ;
#9949=ORIENTED_EDGE ( 'NONE', *, *, #108303, .F. ) ;
#9955=UNCERTAINTY_MEASURE_WITH_UNIT (LENGTH_MEASURE( 1.000000000000000082E-05 ), #59728, 'distance_accuracy_value', 'NONE');
#9983=UNCERTAINTY_MEASURE_WITH_UNIT (LENGTH_MEASURE( 1.000000000000000082E-05 ), #133825, 'distance_accuracy_value', 'NONE');
#10009=DIRECTION ( 'NONE',  ( -1.000000000000000000, -0.000000000000000000, -0.000000000000000000 ) ) ;
#10016=EDGE_CURVE ( 'NONE', #63984, #142234, #118080, .T. ) ;
#10072=CARTESIAN_POINT ( 'NONE',  ( 19.28515664589288647, 1.196650378695337302, -30.59010235425025215 ) ) ;
#10086=MECHANICAL_DESIGN_GEOMETRIC_PRESENTATION_REPRESENTATION('',(#858),#19400);
#10111=EDGE_CURVE ( 'NONE', #113508, #16702, #65744, .T. ) ;
#10121=VECTOR ( 'NONE', #35480, 1000.000000000000000 ) ;
#10179=CARTESIAN_POINT ( 'NONE',  ( 12.19999999999999574, -39.93000000000000682, -40.00000000000000000 ) ) ;
#10184=CARTESIAN_POINT ( 'NONE',  ( 13.41054942568818298, 6.345126847568487882, -31.22086726222595132 ) ) ;
#10197=CARTESIAN_POINT ( 'NONE',  ( -12.20000000000000284, -34.64999999999999147, -39.50000000000000000 ) ) ;
#10204=EDGE_CURVE ( 'NONE', #71183, #43110, #56533, .T. ) ;
#10209=CARTESIAN_POINT ( 'NONE',  ( -6.771599798802371950, -34.64999999999999147, 17.99210858042621908 ) ) ;
#10212=AXIS2_PLACEMENT_3D ( 'NONE', #20470, #108897, #64007 ) ;
#10229=MECHANICAL_DESIGN_GEOMETRIC_PRESENTATION_REPRESENTATION('',(#7941),#17187);
#10291=ADVANCED_FACE ( 'NONE', ( #8158 ), #42270, .T. ) ;
#10295=ORIENTED_EDGE ( 'NONE', *, *, #73754, .T. ) ;
#10322=STYLED_ITEM ( 'NONE', ( #138283 ), #7388 ) ;
#10326=( NAMED_UNIT ( * ) PLANE_ANGLE_UNIT ( ) SI_UNIT ( $, .RADIAN. ) );
#10339=SURFACE_SIDE_STYLE ('',( #111065 ) ) ;
#10340=DIRECTION ( 'NONE',  ( 0.000000000000000000, -1.000000000000000000, 0.000000000000000000 ) ) ;
#10368=CARTESIAN_POINT ( 'NONE',  ( 0.000000000000000000, -40.42999999999999261, 19.06900128115122328 ) ) ;
#10429=EDGE_CURVE ( 'NONE', #79752, #25013, #40149, .T. ) ;
#10450=CARTESIAN_POINT ( 'NONE',  ( 9.461405300130673268, 9.830979504677589631, -29.00227189367402048 ) ) ;
#10515=CARTESIAN_POINT ( 'NONE',  ( -12.20000000000000462, -21.76999999999999247, -40.00000000000000000 ) ) ;
#10516=FILL_AREA_STYLE_COLOUR ( '', #118530 ) ;
#10563=FACE_OUTER_BOUND ( 'NONE', #68307, .T. ) ;
#10598=CARTESIAN_POINT ( 'NONE',  ( -12.20000000000000284, -27.68200100598810209, 15.59110741220538188 ) ) ;
#10647=EDGE_LOOP ( 'NONE', ( #83159, #44774 ) ) ;
#10668=LINE ( 'NONE', #133223, #92463 ) ;
#10679=CARTESIAN_POINT ( 'NONE',  ( 7.940000000000001279, -33.26999999999999602, -10.00000000000000178 ) ) ;
#10712=AXIS2_PLACEMENT_3D ( 'NONE', #73543, #98146, #95272 ) ;
#10749=ORIENTED_EDGE ( 'NONE', *, *, #100523, .F. ) ;
#10753=ADVANCED_FACE ( 'NONE', ( #79021 ), #35522, .T. ) ;
#10763=EDGE_LOOP ( 'NONE', ( #9854, #5512, #58166, #127087, #132725, #106930, #115007, #23359, #46568 ) ) ;
#10768=CARTESIAN_POINT ( 'NONE',  ( 19.75393710176154016, -1.810825152012566219, -32.45514583868006753 ) ) ;
#10780=STYLED_ITEM ( 'NONE', ( #105440 ), #92115 ) ;
#10795=LINE ( 'NONE', #131177, #35628 ) ;
#10818=DIRECTION ( 'NONE',  ( -2.969899378462214681E-16, 0.9667936545734399090, 0.2555582702174445942 ) ) ;
#10820=ORIENTED_EDGE ( 'NONE', *, *, #94769, .F. ) ;
#10893=FACE_OUTER_BOUND ( 'NONE', #96011, .T. ) ;
#10902=( NAMED_UNIT ( * ) SI_UNIT ( $, .STERADIAN. ) SOLID_ANGLE_UNIT ( ) );
#10909=CARTESIAN_POINT ( 'NONE',  ( -17.01299345042646749, -0.9444868035190713274, -36.39086428169088094 ) ) ;
#10966=DIRECTION ( 'NONE',  ( -0.000000000000000000, -1.000000000000000000, -0.000000000000000000 ) ) ;
#11007=CARTESIAN_POINT ( 'NONE',  ( 17.42079396106911560, 4.797059468579773167, -29.42940194308667401 ) ) ;
#11033=DIRECTION ( 'NONE',  ( -1.000000000000000000, 0.000000000000000000, 0.000000000000000000 ) ) ;
#11075=LINE ( 'NONE', #31445, #33712 ) ;
#11080=DIRECTION ( 'NONE',  ( -1.000000000000000000, 0.000000000000000000, -0.000000000000000000 ) ) ;
#11084=MECHANICAL_DESIGN_GEOMETRIC_PRESENTATION_REPRESENTATION('',(#57508),#76009);
#11099=AXIS2_PLACEMENT_3D ( 'NONE', #101049, #56180, #55430 ) ;
#11128=ORIENTED_EDGE ( 'NONE', *, *, #79071, .F. ) ;
#11141=CARTESIAN_POINT ( 'NONE',  ( 16.93425912790457843, 5.488690751113135313, -29.15508941616193539 ) ) ;
#11152=VECTOR ( 'NONE', #46773, 1000.000000000000000 ) ;
#11155=FACE_OUTER_BOUND ( 'NONE', #117967, .T. ) ;
#11161=CARTESIAN_POINT ( 'NONE',  ( -34.92499999999997584, 0.000000000000000000, -0.5000000000000004441 ) ) ;
#11162=CARTESIAN_POINT ( 'NONE',  ( -31.92499999999997584, -21.76999999999999247, -39.50000000000000000 ) ) ;
#11181=UNCERTAINTY_MEASURE_WITH_UNIT (LENGTH_MEASURE( 1.000000000000000082E-05 ), #23420, 'distance_accuracy_value', 'NONE');
#11228=LINE ( 'NONE', #20704, #79271 ) ;
#11310=AXIS2_PLACEMENT_3D ( 'NONE', #123413, #58173, #89325 ) ;
#11343=DIRECTION ( 'NONE',  ( -1.000000000000000000, -3.115803279706882722E-16, 0.000000000000000000 ) ) ;
#11378=DIRECTION ( 'NONE',  ( 1.000000000000000000, 0.000000000000000000, 0.000000000000000000 ) ) ;
#11410=FILL_AREA_STYLE ('',( #110726 ) ) ;
#11421=ORIENTED_EDGE ( 'NONE', *, *, #45142, .F. ) ;
#11461=CARTESIAN_POINT ( 'NONE',  ( 12.69999999999999574, -22.26999999999999247, -0.2071067811865477670 ) ) ;
#11533=CARTESIAN_POINT ( 'NONE',  ( 16.93289034258302550, -0.6086847910684115570, -34.86941310074139011 ) ) ;
#11547=ORIENTED_EDGE ( 'NONE', *, *, #55115, .T. ) ;
#11613=VECTOR ( 'NONE', #675, 1000.000000000000000 ) ;
#11637=ORIENTED_EDGE ( 'NONE', *, *, #128832, .T. ) ;
#11658=DIRECTION ( 'NONE',  ( 1.000000000000000000, 0.000000000000000000, 0.000000000000000000 ) ) ;
#11669=FILL_AREA_STYLE ('',( #110992 ) ) ;
#11687=CARTESIAN_POINT ( 'NONE',  ( -7.122370700763609008, -39.92999999999999261, 19.06900128115122328 ) ) ;
#11707=AXIS2_PLACEMENT_3D ( 'NONE', #14368, #4129, #61482 ) ;
#11710=AXIS2_PLACEMENT_3D ( 'NONE', #13953, #100982, #133631 ) ;
#11716=AXIS2_PLACEMENT_3D ( 'NONE', #3510, #15107, #14422 ) ;
#11722=FACE_OUTER_BOUND ( 'NONE', #52523, .T. ) ;
#11745=EDGE_LOOP ( 'NONE', ( #142019, #9102, #29773, #311 ) ) ;
#11821=CARTESIAN_POINT ( 'NONE',  ( 33.51679449616821671, 22.27000000000000668, -13.80793696990846620 ) ) ;
#11827=VECTOR ( 'NONE', #140660, 1000.000000000000000 ) ;
#11829=AXIS2_PLACEMENT_3D ( 'NONE', #134413, #24910, #93031 ) ;
#11855=AXIS2_PLACEMENT_3D ( 'NONE', #87493, #53428, #119373 ) ;
#11875=CARTESIAN_POINT ( 'NONE',  ( 14.45122993026753377, 4.938655920609167360, -31.93222277579656776 ) ) ;
#11898=CIRCLE ( 'NONE', #60598, 1.898649999999994842 ) ;
#11968=ADVANCED_BREP_SHAPE_REPRESENTATION ( '', ( #142469, #127880 ), #35272 ) ;
#11972=AXIS2_PLACEMENT_3D ( 'NONE', #110290, #10966, #55233 ) ;
#11983=CARTESIAN_POINT ( 'NONE',  ( 0.000000000000000000, -4.870000000000014317, -10.00000000000000178 ) ) ;
#11998=LINE ( 'NONE', #112753, #116317 ) ;
#12014=PRODUCT_DEFINITION ( 'UNKNOWN', '', #132846, #61802 ) ;
#12021=DIRECTION ( 'NONE',  ( 2.496005001405478586E-15, 1.000000000000000000, -0.000000000000000000 ) ) ;
#12028=CARTESIAN_POINT ( 'NONE',  ( -12.70000000000000995, 12.19802518668052471, 4.711086268963014412 ) ) ;
#12055=FACE_OUTER_BOUND ( 'NONE', #113673, .T. ) ;
#12064=CONICAL_SURFACE ( 'NONE', #93112, 9.524999999999991473, 1.029744258676653645 ) ;
#12099=DIRECTION ( 'NONE',  ( 0.000000000000000000, -0.000000000000000000, -1.000000000000000000 ) ) ;
#12107=CARTESIAN_POINT ( 'NONE',  ( 17.52071992270299106, -3.088060075592792497, -34.88610987998131208 ) ) ;
#12161=CARTESIAN_POINT ( 'NONE',  ( -7.940000000000001279, -33.26999999999999602, -8.101350000000008933 ) ) ;
#12164=VERTEX_POINT ( 'NONE', #105726 ) ;
#12180=EDGE_CURVE ( 'NONE', #22506, #129819, #48065, .T. ) ;
#12236=DIRECTION ( 'NONE',  ( -0.000000000000000000, -0.000000000000000000, 1.000000000000000000 ) ) ;
#12247=EDGE_LOOP ( 'NONE', ( #93015, #66710, #102469, #60919 ) ) ;
#12529=ORIENTED_EDGE ( 'NONE', *, *, #57276, .F. ) ;
#12579=SURFACE_STYLE_FILL_AREA ( #99574 ) ;
#12603=CARTESIAN_POINT ( 'NONE',  ( 15.53628966088338004, 3.145490004818007446, -30.03788422909113720 ) ) ;
#12615=FACE_OUTER_BOUND ( 'NONE', #113746, .T. ) ;
#12638=( NAMED_UNIT ( * ) SI_UNIT ( $, .STERADIAN. ) SOLID_ANGLE_UNIT ( ) );
#12664=UNCERTAINTY_MEASURE_WITH_UNIT (LENGTH_MEASURE( 1.000000000000000082E-05 ), #120019, 'distance_accuracy_value', 'NONE');
#12695=ORIENTED_EDGE ( 'NONE', *, *, #120626, .T. ) ;
#12716=SURFACE_STYLE_USAGE ( .BOTH. , #25015 ) ;
#12726=CARTESIAN_POINT ( 'NONE',  ( 7.939999999999994174, -39.93000000000000682, -12.24789999999999957 ) ) ;
#12803=UNCERTAINTY_MEASURE_WITH_UNIT (LENGTH_MEASURE( 1.000000000000000082E-05 ), #9369, 'distance_accuracy_value', 'NONE');
#12855=( NAMED_UNIT ( * ) PLANE_ANGLE_UNIT ( ) SI_UNIT ( $, .RADIAN. ) );
#12877=CARTESIAN_POINT ( 'NONE',  ( -12.20000000000000284, -25.47159979880235881, 14.98806839329795260 ) ) ;
#12908=STYLED_ITEM ( 'NONE', ( #125167 ), #133441 ) ;
#12930=PRESENTATION_STYLE_ASSIGNMENT (( #71629 ) ) ;
#12978=FILL_AREA_STYLE ('',( #99264 ) ) ;
#13012=DIRECTION ( 'NONE',  ( 0.000000000000000000, 0.000000000000000000, 1.000000000000000000 ) ) ;
#13018=ORIENTED_EDGE ( 'NONE', *, *, #45142, .T. ) ;
#13112=ORIENTED_EDGE ( 'NONE', *, *, #9743, .T. ) ;
#13157=CARTESIAN_POINT ( 'NONE',  ( 15.56310719811854959, 7.173451295978907183, -28.42221963501224025 ) ) ;
#13211=AXIS2_PLACEMENT_3D ( 'NONE', #10368, #54623, #108959 ) ;
#13239=FACE_OUTER_BOUND ( 'NONE', #33860, .T. ) ;
#13262=ORIENTED_EDGE ( 'NONE', *, *, #79213, .T. ) ;
#13280=PRESENTATION_STYLE_ASSIGNMENT (( #69873 ) ) ;
#13301=CARTESIAN_POINT ( 'NONE',  ( 16.67979525387081807, 0.3337821591035673441, -30.81818940114110816 ) ) ;
#13335=EDGE_CURVE ( 'NONE', #140981, #41660, #114507, .T. ) ;
#13365=SURFACE_STYLE_FILL_AREA ( #88108 ) ;
#13368=CARTESIAN_POINT ( 'NONE',  ( 12.19999999999999574, -25.33999999999998565, 2.999999999999999112 ) ) ;
#13414=( NAMED_UNIT ( * ) SI_UNIT ( $, .STERADIAN. ) SOLID_ANGLE_UNIT ( ) );
#13442=EDGE_CURVE ( 'NONE', #121504, #878, #31797, .T. ) ;
#13467=CARTESIAN_POINT ( 'NONE',  ( 34.92500000000001847, 1.088194295437629318E-14, 0.000000000000000000 ) ) ;
#13519=CARTESIAN_POINT ( 'NONE',  ( 19.71979893569068309, -1.560063818677258851, -32.18359520017570219 ) ) ;
#13538=VERTEX_POINT ( 'NONE', #27319 ) ;
#13615=ADVANCED_FACE ( 'NONE', ( #59982 ), #22447, .F. ) ;
#13672=ORIENTED_EDGE ( 'NONE', *, *, #56935, .T. ) ;
#13698=COLOUR_RGB ( '', 0.40784314, 0.44705882, 0.49803922) ;
#13741=CIRCLE ( 'NONE', #39010, 2.247899999999996901 ) ;
#13752=PLANE ( 'NONE',  #66531 ) ;
#13758=ORIENTED_EDGE ( 'NONE', *, *, #17622, .T. ) ;
#13759=LINE ( 'NONE', #74975, #105388 ) ;
#13807=FACE_OUTER_BOUND ( 'NONE', #54293, .T. ) ;
#13819=ORIENTED_EDGE ( 'NONE', *, *, #40600, .T. ) ;
#13826=DIRECTION ( 'NONE',  ( -1.000000000000000000, 0.000000000000000000, 0.000000000000000000 ) ) ;
#13890=ORIENTED_EDGE ( 'NONE', *, *, #9300, .F. ) ;
#13917=CARTESIAN_POINT ( 'NONE',  ( -34.92499999999997584, 22.27000000000000668, -7.752744394707050901 ) ) ;
#13953=CARTESIAN_POINT ( 'NONE',  ( -12.70000000000000462, -22.33999999999998565, 3.000000000000000000 ) ) ;
#13961=CARTESIAN_POINT ( 'NONE',  ( 34.62665285692208528, 22.27000000000001023, -11.14529726906961749 ) ) ;
#13978=VERTEX_POINT ( 'NONE', #33787 ) ;
#13983=VERTEX_POINT ( 'NONE', #67864 ) ;
#13988=CIRCLE ( 'NONE', #76549, 3.000000000000002665 ) ;
#13992=CIRCLE ( 'NONE', #92758, 2.999999999999999112 ) ;
#13996=FILL_AREA_STYLE_COLOUR ( '', #26405 ) ;
#14034=SURFACE_STYLE_FILL_AREA ( #80066 ) ;
#14087=EDGE_CURVE ( 'NONE', #22506, #2401, #13992, .T. ) ;
#14161=EDGE_CURVE ( 'NONE', #131125, #82818, #18642, .T. ) ;
#14205=COLOUR_RGB ( '', 0.08235294, 0.09019608, 0.10196078) ;
#14238=CIRCLE ( 'NONE', #125406, 0.5000000000000000000 ) ;
#14253=CARTESIAN_POINT ( 'NONE',  ( 0.000000000000000000, -4.870000000000014317, -40.00000000000000000 ) ) ;
#14259=CARTESIAN_POINT ( 'NONE',  ( 16.99081895618983751, -0.8493047346644202467, -35.56339853354601388 ) ) ;
#14272=CARTESIAN_POINT ( 'NONE',  ( -21.60769999999998703, 3.130000000000008331, -22.35000000000000142 ) ) ;
#14299=ORIENTED_EDGE ( 'NONE', *, *, #60631, .T. ) ;
#14319=VECTOR ( 'NONE', #8164, 1000.000000000000000 ) ;
#14342=B_SPLINE_CURVE_WITH_KNOTS ( 'NONE', 3,
 ( #126962, #116090, #106621, #73335, #26945, #83495, #115342, #137152, #29790, #118219, #28393, #72653, #18925, #16033, #17494, #61748, #105910, #103768, #139320, #8028, #85597, #75468, #9445, #63191, #41390, #52965, #65327, #53724, #108756, #97927, #142854, #88491, #21059, #86349, #131993, #96452, #97163, #130569, #10184, #42139, #109509, #54448, #32685, #107362, #132731, #141427 ),
 .UNSPECIFIED., .F., .F.,
 ( 4, 2, 2, 2, 2, 2, 2, 2, 2, 2, 2, 2, 2, 2, 2, 2, 2, 2, 2, 2, 2, 2, 4 ),
 ( 0.000000000000000000, 0.002810485862540013525, 0.005620971725080024448, 0.007026214656350030993, 0.008431457587620039273, 0.01124194345016004543, 0.01264718638143005197, 0.01405242931270006025, 0.01686291517524007855, 0.01826815810651008856, 0.01967340103778009511, 0.02248388690032011861, 0.02388912983159013209, 0.02529437276286013864, 0.02810485862540016214, 0.02951010155667016868, 0.03091534448794018217, 0.03372583035048019873, 0.03653631621302021876, 0.03934680207556023879, 0.04075204500683024533, 0.04215728793810025188, 0.04496777380064026497 ),
 .UNSPECIFIED. ) ;
#14352=EDGE_CURVE ( 'NONE', #109349, #87614, #4745, .T. ) ;
#14368=CARTESIAN_POINT ( 'NONE',  ( 0.000000000000000000, -34.64999999999999147, 17.49210858042621908 ) ) ;
#14404=DIRECTION ( 'NONE',  ( -0.000000000000000000, -1.000000000000000000, -0.000000000000000000 ) ) ;
#14422=DIRECTION ( 'NONE',  ( 0.000000000000000000, 2.775557561562888827E-14, 1.000000000000000000 ) ) ;
#14440=DIRECTION ( 'NONE',  ( 0.000000000000000000, 0.000000000000000000, 1.000000000000000000 ) ) ;
#14562=( GEOMETRIC_REPRESENTATION_CONTEXT ( 3 ) GLOBAL_UNCERTAINTY_ASSIGNED_CONTEXT ( ( #22798 ) ) GLOBAL_UNIT_ASSIGNED_CONTEXT ( ( #9007, #132309, #88791 ) ) REPRESENTATION_CONTEXT ( 'NONE', 'WORKASPACE' ) );
#14614=CARTESIAN_POINT ( 'NONE',  ( -12.59816835436673621, 9.780221332989524896, -27.05079659061421182 ) ) ;
#14615=DIRECTION ( 'NONE',  ( -1.000000000000000000, 0.000000000000000000, 0.000000000000000000 ) ) ;
#14631=EDGE_LOOP ( 'NONE', ( #64050, #7888, #132003 ) ) ;
#14667=EDGE_LOOP ( 'NONE', ( #35487, #36498, #72551, #15198 ) ) ;
#14681=DIRECTION ( 'NONE',  ( 0.000000000000000000, 0.000000000000000000, -1.000000000000000000 ) ) ;
#14683=( NAMED_UNIT ( * ) PLANE_ANGLE_UNIT ( ) SI_UNIT ( $, .RADIAN. ) );
#14686=EDGE_LOOP ( 'NONE', ( #29095, #91055, #37837 ) ) ;
#14704=CARTESIAN_POINT ( 'NONE',  ( 34.55179764501523465, 22.26999999999999957, -11.48108961241408998 ) ) ;
#14708=FILL_AREA_STYLE ('',( #27006 ) ) ;
#14724=STYLED_ITEM ( 'NONE', ( #128682 ), #19464 ) ;
#14732=DIRECTION ( 'NONE',  ( 0.000000000000000000, 0.2631995976047524777, 0.9647414015272156584 ) ) ;
#14801=CARTESIAN_POINT ( 'NONE',  ( 12.19999999999999574, -39.93000000000001393, 19.45086547876359617 ) ) ;
#14805=SURFACE_STYLE_FILL_AREA ( #56921 ) ;
#14881=AXIS2_PLACEMENT_3D ( 'NONE', #37965, #69905, #48121 ) ;
#14893=( LENGTH_UNIT ( ) NAMED_UNIT ( * ) SI_UNIT ( .MILLI., .METRE. ) );
#14912=VERTEX_POINT ( 'NONE', #105603 ) ;
#14936=AXIS2_PLACEMENT_3D ( 'NONE', #5164, #92922, #49461 ) ;
#14958=CARTESIAN_POINT ( 'NONE',  ( 19.39435622689822480, 0.5802795747914162305, -30.75303128506508088 ) ) ;
#14989=ORIENTED_EDGE ( 'NONE', *, *, #124322, .F. ) ;
#15078=AXIS2_PLACEMENT_3D ( 'NONE', #57349, #34152, #111704 ) ;
#15079=FACE_OUTER_BOUND ( 'NONE', #133185, .T. ) ;
#15107=DIRECTION ( 'NONE',  ( 1.000000000000000000, -0.000000000000000000, -0.000000000000000000 ) ) ;
#15135=VECTOR ( 'NONE', #66225, 1000.000000000000114 ) ;
#15183=DIRECTION ( 'NONE',  ( 1.000000000000000000, 0.000000000000000000, 0.000000000000000000 ) ) ;
#15191=VERTEX_POINT ( 'NONE', #12726 ) ;
#15198=ORIENTED_EDGE ( 'NONE', *, *, #36598, .T. ) ;
#15227=AXIS2_PLACEMENT_3D ( 'NONE', #138905, #136023, #61378 ) ;
#15232=MECHANICAL_DESIGN_GEOMETRIC_PRESENTATION_REPRESENTATION('',(#98562),#57005);
#15333=CIRCLE ( 'NONE', #31624, 0.5000000000000004441 ) ;
#15381=SURFACE_STYLE_USAGE ( .BOTH. , #103141 ) ;
#15423=CIRCLE ( 'NONE', #131271, 0.5000000000000004441 ) ;
#15466=EDGE_LOOP ( 'NONE', ( #133658, #119771, #135127, #95629 ) ) ;
#15476=EDGE_LOOP ( 'NONE', ( #131384, #2479, #124770, #134830 ) ) ;
#15491=UNCERTAINTY_MEASURE_WITH_UNIT (LENGTH_MEASURE( 1.000000000000000082E-05 ), #83953, 'distance_accuracy_value', 'NONE');
#15508=LINE ( 'NONE', #82263, #97596 ) ;
#15586=CARTESIAN_POINT ( 'NONE',  ( -12.52134243846371398, 7.306103351283218750, -30.66480774954007416 ) ) ;
#15600=CARTESIAN_POINT ( 'NONE',  ( -7.940000000000001279, -60.26999999999998892, -10.00000000000000178 ) ) ;
#15625=UNCERTAINTY_MEASURE_WITH_UNIT (LENGTH_MEASURE( 1.000000000000000082E-05 ), #51391, 'distance_accuracy_value', 'NONE');
#15639=CARTESIAN_POINT ( 'NONE',  ( 17.01022479757872219, -0.9324317514308457788, -36.05569165383651153 ) ) ;
#15660=LINE ( 'NONE', #38196, #94651 ) ;
#15692=ADVANCED_FACE ( 'NONE', ( #103145 ), #116256, .T. ) ;
#15730=AXIS2_PLACEMENT_3D ( 'NONE', #84840, #29719, #95707 ) ;
#15748=FILL_AREA_STYLE ('',( #70925 ) ) ;
#15831=EDGE_CURVE ( 'NONE', #40891, #44308, #53670, .T. ) ;
#15851=AXIS2_PLACEMENT_3D ( 'NONE', #99831, #131041, #42631 ) ;
#15870=PRESENTATION_STYLE_ASSIGNMENT (( #48556 ) ) ;
#15958=MECHANICAL_DESIGN_GEOMETRIC_PRESENTATION_REPRESENTATION('',(#25208),#136349);
#16008=DIRECTION ( 'NONE',  ( -0.8571673007021110013, 1.049727191138617093E-16, 0.5150380749100563760 ) ) ;
#16020=ORIENTED_EDGE ( 'NONE', *, *, #20401, .F. ) ;
#16033=CARTESIAN_POINT ( 'NONE',  ( -8.782784137141019798, 10.22668762134568077, -28.70197684735530075 ) ) ;
#16071=AXIS2_PLACEMENT_3D ( 'NONE', #523, #11378, #33221 ) ;
#16091=( LENGTH_UNIT ( ) NAMED_UNIT ( * ) SI_UNIT ( .MILLI., .METRE. ) );
#16116=CYLINDRICAL_SURFACE ( 'NONE', #97673, 6.000000000000000000 ) ;
#16124=FILL_AREA_STYLE ('',( #95137 ) ) ;
#16169=MECHANICAL_DESIGN_GEOMETRIC_PRESENTATION_REPRESENTATION('',(#134295),#27793);
#16183=ADVANCED_FACE ( 'NONE', ( #129712 ), #84794, .T. ) ;
#16228=ORIENTED_EDGE ( 'NONE', *, *, #6261, .T. ) ;
#16240=CARTESIAN_POINT ( 'NONE',  ( 6.639999999999993463, -34.64999999999999858, -40.00000000000000000 ) ) ;
#16256=AXIS2_PLACEMENT_3D ( 'NONE', #137371, #82984, #61281 ) ;
#16265=AXIS2_PLACEMENT_3D ( 'NONE', #69082, #115374, #136448 ) ;
#16314=EDGE_LOOP ( 'NONE', ( #24492, #9539, #52690, #71646 ) ) ;
#16318=CARTESIAN_POINT ( 'NONE',  ( -10.92112245905905610, 8.781005371807186322, -29.73817149962091477 ) ) ;
#16322=DIRECTION ( 'NONE',  ( 1.000000000000000000, 3.115803279706882722E-16, -0.000000000000000000 ) ) ;
#16328=ORIENTED_EDGE ( 'NONE', *, *, #113493, .T. ) ;
#16373=CARTESIAN_POINT ( 'NONE',  ( 17.54957349249705700, -3.269999999999996909, -36.39086428169088094 ) ) ;
#16412=DIRECTION ( 'NONE',  ( 0.000000000000000000, 0.000000000000000000, 1.000000000000000000 ) ) ;
#16478=TOROIDAL_SURFACE ( 'NONE', #11829, 6.000000000000000000, 3.000000000000000000 ) ;
#16484=ORIENTED_EDGE ( 'NONE', *, *, #140396, .T. ) ;
#16501=( NAMED_UNIT ( * ) SI_UNIT ( $, .STERADIAN. ) SOLID_ANGLE_UNIT ( ) );
#16507=DIRECTION ( 'NONE',  ( 1.000000000000000000, 0.000000000000000000, 0.000000000000000000 ) ) ;
#16531=CARTESIAN_POINT ( 'NONE',  ( -31.92499999999997584, -6.270000000000012896, -36.39086428169088094 ) ) ;
#16548=ORIENTED_EDGE ( 'NONE', *, *, #27767, .F. ) ;
#16594=MECHANICAL_DESIGN_GEOMETRIC_PRESENTATION_REPRESENTATION('',(#55964),#74479);
#16608=DIRECTION ( 'NONE',  ( -3.115803279706882722E-16, 1.000000000000000000, -0.000000000000000000 ) ) ;
#16616=ORIENTED_EDGE ( 'NONE', *, *, #128025, .T. ) ;
#16702=VERTEX_POINT ( 'NONE', #66988 ) ;
#16728=FILL_AREA_STYLE_COLOUR ( '', #111173 ) ;
#16748=CARTESIAN_POINT ( 'NONE',  ( -13.39050432165378446, 9.181379155046611729, -27.39219850300061765 ) ) ;
#16793=CARTESIAN_POINT ( 'NONE',  ( 12.19999999999999574, -25.33999999999998920, 13.17925390838734323 ) ) ;
#16821=( GEOMETRIC_REPRESENTATION_CONTEXT ( 3 ) GLOBAL_UNCERTAINTY_ASSIGNED_CONTEXT ( ( #73823 ) ) GLOBAL_UNIT_ASSIGNED_CONTEXT ( ( #40008, #50148, #52269 ) ) REPRESENTATION_CONTEXT ( 'NONE', 'WORKASPACE' ) );
#16869=ORIENTED_EDGE ( 'NONE', *, *, #20291, .F. ) ;
#16954=DIRECTION ( 'NONE',  ( 0.000000000000000000, -0.000000000000000000, -1.000000000000000000 ) ) ;
#16955=CARTESIAN_POINT ( 'NONE',  ( 7.139999999999985469, -39.93000000000000682, -7.899272885403731514 ) ) ;
#16994=LINE ( 'NONE', #39476, #83395 ) ;
#17002=EDGE_CURVE ( 'NONE', #124237, #98685, #98704, .T. ) ;
#17004=ORIENTED_EDGE ( 'NONE', *, *, #177, .F. ) ;
#17050=DIRECTION ( 'NONE',  ( 0.000000000000000000, 0.000000000000000000, -1.000000000000000000 ) ) ;
#17071=CARTESIAN_POINT ( 'NONE',  ( -16.11017474120846060, 1.958518950653415303, -30.40717620614491068 ) ) ;
#17111=CYLINDRICAL_SURFACE ( 'NONE', #15227, 1.898649999999994842 ) ;
#17183=DIRECTION ( 'NONE',  ( -0.000000000000000000, 0.000000000000000000, 1.000000000000000000 ) ) ;
#17187=( GEOMETRIC_REPRESENTATION_CONTEXT ( 3 ) GLOBAL_UNCERTAINTY_ASSIGNED_CONTEXT ( ( #108726 ) ) GLOBAL_UNIT_ASSIGNED_CONTEXT ( ( #90147, #122777, #2395 ) ) REPRESENTATION_CONTEXT ( 'NONE', 'WORKASPACE' ) );
#17193=CARTESIAN_POINT ( 'NONE',  ( 12.19999999999999574, -59.76999999999998892, -39.50000000000000000 ) ) ;
#17225=CARTESIAN_POINT ( 'NONE',  ( 12.19999999999999574, -40.43000000000000682, -40.00000000000000000 ) ) ;
#17255=EDGE_CURVE ( 'NONE', #91102, #73050, #93556, .T. ) ;
#17277=CARTESIAN_POINT ( 'NONE',  ( 7.939999999999994174, -60.26999999999998892, -10.00000000000000178 ) ) ;
#17316=CARTESIAN_POINT ( 'NONE',  ( -12.20000000000000284, -35.14999999999999147, -39.50000000000000000 ) ) ;
#17392=ORIENTED_EDGE ( 'NONE', *, *, #26645, .F. ) ;
#17397=CARTESIAN_POINT ( 'NONE',  ( 6.639999999999984581, -40.42999999999999972, -40.00000000000000000 ) ) ;
#17405=CARTESIAN_POINT ( 'NONE',  ( -34.42499999999997584, -22.26999999999999247, -40.00000000000000000 ) ) ;
#17444=AXIS2_PLACEMENT_3D ( 'NONE', #123235, #112341, #134835 ) ;
#17470=LINE ( 'NONE', #105885, #118398 ) ;
#17494=CARTESIAN_POINT ( 'NONE',  ( -8.396172048266301147, 10.44511258719185953, -28.53519072974560800 ) ) ;
#17507=EDGE_LOOP ( 'NONE', ( #29832, #13112, #140233, #40422 ) ) ;
#17518=DIRECTION ( 'NONE',  ( 0.000000000000000000, 1.000000000000000000, 0.000000000000000000 ) ) ;
#17539=CARTESIAN_POINT ( 'NONE',  ( -19.28515664589289003, 1.196650378695325090, -30.59010235425025215 ) ) ;
#17547=( NAMED_UNIT ( * ) PLANE_ANGLE_UNIT ( ) SI_UNIT ( $, .RADIAN. ) );
#17556=COLOUR_RGB ( '', 0.72549020, 0.75294118, 0.79215686) ;
#17617=LINE ( 'NONE', #127102, #83003 ) ;
#17622=EDGE_CURVE ( 'NONE', #81439, #80081, #143465, .T. ) ;
#17650=CIRCLE ( 'NONE', #110264, 9.524999999999998579 ) ;
#17677=CARTESIAN_POINT ( 'NONE',  ( -16.45742106731621845, 0.9613713492673547911, -33.49048331797055766 ) ) ;
#17712=FILL_AREA_STYLE_COLOUR ( '', #23152 ) ;
#17748=CARTESIAN_POINT ( 'NONE',  ( -18.92851995498817530, 2.123550300856637207, -30.34508942967045186 ) ) ;
#17755=LINE ( 'NONE', #103342, #77629 ) ;
#17782=VERTEX_POINT ( 'NONE', #103484 ) ;
#17785=EDGE_LOOP ( 'NONE', ( #32631, #62652, #73622, #36329 ) ) ;
#17884=( NAMED_UNIT ( * ) SI_UNIT ( $, .STERADIAN. ) SOLID_ANGLE_UNIT ( ) );
#17992=PRESENTATION_STYLE_ASSIGNMENT (( #41944 ) ) ;
#18059=ORIENTED_EDGE ( 'NONE', *, *, #47667, .F. ) ;
#18081=ADVANCED_FACE ( 'NONE', ( #112093 ), #48797, .T. ) ;
#18110=SURFACE_SIDE_STYLE ('',( #59043 ) ) ;
#18199=FILL_AREA_STYLE ('',( #29116 ) ) ;
#18206=CYLINDRICAL_SURFACE ( 'NONE', #8417, 2.552699999999994418 ) ;
#18226=EDGE_CURVE ( 'NONE', #118457, #38058, #113651, .T. ) ;
#18268=DIRECTION ( 'NONE',  ( 2.496005001405478586E-15, 1.000000000000000000, -0.000000000000000000 ) ) ;
#18320=CARTESIAN_POINT ( 'NONE',  ( 12.19999999999999574, -40.43000000000000682, -39.50000000000000000 ) ) ;
#18335=AXIS2_PLACEMENT_3D ( 'NONE', #65721, #86724, #43221 ) ;
#18426=EDGE_CURVE ( 'NONE', #38919, #104775, #65400, .T. ) ;
#18453=CARTESIAN_POINT ( 'NONE',  ( 12.77438429321126812, 9.652835684742514744, -27.12452711299875574 ) ) ;
#18479=DIRECTION ( 'NONE',  ( -1.000000000000000000, 2.496005001405478586E-15, -6.809571051365719919E-16 ) ) ;
#18480=CARTESIAN_POINT ( 'NONE',  ( -7.122370700763609008, -39.92999999999999261, 19.06900128115122328 ) ) ;
#18550=DIRECTION ( 'NONE',  ( 0.000000000000000000, -1.000000000000000000, 0.000000000000000000 ) ) ;
#18555=FACE_OUTER_BOUND ( 'NONE', #135254, .T. ) ;
#18564=ORIENTED_EDGE ( 'NONE', *, *, #128832, .F. ) ;
#18600=ORIENTED_EDGE ( 'NONE', *, *, #97500, .F. ) ;
#18608=ORIENTED_EDGE ( 'NONE', *, *, #17002, .T. ) ;
#18642=CIRCLE ( 'NONE', #16256, 2.552699999999997971 ) ;
#18695=DIRECTION ( 'NONE',  ( 3.115803279706882722E-16, -1.000000000000000000, 0.000000000000000000 ) ) ;
#18698=ORIENTED_EDGE ( 'NONE', *, *, #80182, .F. ) ;
#18717=EDGE_CURVE ( 'NONE', #122313, #61905, #62362, .T. ) ;
#18720=EDGE_CURVE ( 'NONE', #86478, #6439, #130764, .T. ) ;
#18750=LINE ( 'NONE', #62297, #138026 ) ;
#18789=CARTESIAN_POINT ( 'NONE',  ( -8.773457579940252170E-14, -35.14999999999997726, -40.00000000000000000 ) ) ;
#18790=CARTESIAN_POINT ( 'NONE',  ( 12.69999999999999574, -40.43000000000000682, -40.00000000000000000 ) ) ;
#18805=CARTESIAN_POINT ( 'NONE',  ( 19.83042955554208220, -2.395858916147067585, -33.25513085038058136 ) ) ;
#18816=CARTESIAN_POINT ( 'NONE',  ( -31.92499999999997584, -21.76999999999999247, -40.00000000000000000 ) ) ;
#18833=VERTEX_POINT ( 'NONE', #33329 ) ;
#18888=ORIENTED_EDGE ( 'NONE', *, *, #29080, .F. ) ;
#18891=( NAMED_UNIT ( * ) PLANE_ANGLE_UNIT ( ) SI_UNIT ( $, .RADIAN. ) );
#18925=CARTESIAN_POINT ( 'NONE',  ( -9.535978227293808729, 9.762579867702294578, -29.04603976045208569 ) ) ;
#18926=SURFACE_SIDE_STYLE ('',( #94345 ) ) ;
#18973=DIRECTION ( 'NONE',  ( 1.000000000000000000, 0.000000000000000000, 0.000000000000000000 ) ) ;
#19005=CARTESIAN_POINT ( 'NONE',  ( -6.932893218813454439, -34.94289321881344534, -40.00000000000000000 ) ) ;
#19205=AXIS2_PLACEMENT_3D ( 'NONE', #95373, #65662, #62775 ) ;
#19207=CARTESIAN_POINT ( 'NONE',  ( 15.02190751083870524, 7.730481892681857481, -28.15093226488858491 ) ) ;
#19226=AXIS2_PLACEMENT_3D ( 'NONE', #11162, #43139, #55439 ) ;
#19400=( GEOMETRIC_REPRESENTATION_CONTEXT ( 3 ) GLOBAL_UNCERTAINTY_ASSIGNED_CONTEXT ( ( #57641 ) ) GLOBAL_UNIT_ASSIGNED_CONTEXT ( ( #49956, #73831, #29593 ) ) REPRESENTATION_CONTEXT ( 'NONE', 'WORKASPACE' ) );
#19433=DIRECTION ( 'NONE',  ( -1.000000000000000000, -3.115803279706882722E-16, 0.000000000000000000 ) ) ;
#19438=AXIS2_PLACEMENT_3D ( 'NONE', #131163, #33327, #31855 ) ;
#19439=CARTESIAN_POINT ( 'NONE',  ( -12.70000000000000462, -22.26999999999999247, -39.79289321881346098 ) ) ;
#19463=ORIENTED_EDGE ( 'NONE', *, *, #60595, .T. ) ;
#19464=ADVANCED_FACE ( 'NONE', ( #12055 ), #103475, .F. ) ;
#19482=VERTEX_POINT ( 'NONE', #2418 ) ;
#19504=CARTESIAN_POINT ( 'NONE',  ( 7.139999999999994351, -35.14999999999999147, -39.79289321881344677 ) ) ;
#19574=( NAMED_UNIT ( * ) PLANE_ANGLE_UNIT ( ) SI_UNIT ( $, .RADIAN. ) );
#19578=EDGE_LOOP ( 'NONE', ( #82400, #124647, #132086, #88529 ) ) ;
#19602=CIRCLE ( 'NONE', #38149, 1.898649999999994842 ) ;
#19668=( NAMED_UNIT ( * ) PLANE_ANGLE_UNIT ( ) SI_UNIT ( $, .RADIAN. ) );
#19743=EDGE_CURVE ( 'NONE', #133539, #100573, #77548, .T. ) ;
#19795=DIRECTION ( 'NONE',  ( 1.000000000000000000, 0.000000000000000000, 0.000000000000000000 ) ) ;
#19900=CARTESIAN_POINT ( 'NONE',  ( -5.900168161225546548, 12.95172380562260805, -24.96972421923774377 ) ) ;
#19955=CARTESIAN_POINT ( 'NONE',  ( -12.20000000000000284, -34.64999999999999147, -40.00000000000000000 ) ) ;
#19961=FILL_AREA_STYLE ('',( #52597 ) ) ;
#19986=ADVANCED_FACE ( 'NONE', ( #6325 ), #37093, .T. ) ;
#20074=VECTOR ( 'NONE', #15183, 1000.000000000000000 ) ;
#20082=VERTEX_POINT ( 'NONE', #72401 ) ;
#20108=CARTESIAN_POINT ( 'NONE',  ( -12.20000000000000462, -21.76999999999999247, 0.000000000000000000 ) ) ;
#20113=( NAMED_UNIT ( * ) PLANE_ANGLE_UNIT ( ) SI_UNIT ( $, .RADIAN. ) );
#20149=EDGE_LOOP ( 'NONE', ( #85106, #37189, #137791, #83566 ) ) ;
#20195=CARTESIAN_POINT ( 'NONE',  ( 12.19999999999999574, -21.76999999999999247, -40.00000000000000000 ) ) ;
#20221=CARTESIAN_POINT ( 'NONE',  ( 19.65643278553995543, -1.111889603260001858, -31.77067279039590986 ) ) ;
#20290=DIRECTION ( 'NONE',  ( 0.000000000000000000, -1.000000000000000000, 0.000000000000000000 ) ) ;
#20291=EDGE_CURVE ( 'NONE', #7925, #132295, #34726, .T. ) ;
#20301=CARTESIAN_POINT ( 'NONE',  ( 7.139999999999956160, -60.26999999999998892, -11.72188031596273206 ) ) ;
#20343=CARTESIAN_POINT ( 'NONE',  ( 7.139999999999989910, -35.05528132343074788, 17.90627459364450402 ) ) ;
#20361=( BOUNDED_CURVE ( )  B_SPLINE_CURVE ( 3, ( #134388, #123529, #24192, #69871 ),
 .UNSPECIFIED., .F., .T. ) 
 B_SPLINE_CURVE_WITH_KNOTS ( ( 4, 4 ),
 ( 0.2663372438543372689, 1.570796326794905440 ),
 .UNSPECIFIED. ) 
 CURVE ( )  GEOMETRIC_REPRESENTATION_ITEM ( )  RATIONAL_B_SPLINE_CURVE ( ( 1.000000000000000000, 0.8631550219135034618, 0.8631550219135034618, 1.000000000000000000 ) ) 
 REPRESENTATION_ITEM ( '' )  );
#20401=EDGE_CURVE ( 'NONE', #131359, #2907, #78530, .T. ) ;
#20454=CARTESIAN_POINT ( 'NONE',  ( -6.640000000000001457, -35.14999999999999147, -40.00000000000000000 ) ) ;
#20470=CARTESIAN_POINT ( 'NONE',  ( -5.045674110341171311E-14, -40.42999999999999261, -39.50000000000000000 ) ) ;
#20491=CARTESIAN_POINT ( 'NONE',  ( -55.65468426143998215, -25.33999999999998920, 15.47043909406156281 ) ) ;
#20503=DIRECTION ( 'NONE',  ( 0.000000000000000000, 1.000000000000000000, 0.000000000000000000 ) ) ;
#20600=CARTESIAN_POINT ( 'NONE',  ( -19.93618820137057668, -0.2700000000508183118, -36.99999999997771738 ) ) ;
#20615=CARTESIAN_POINT ( 'NONE',  ( 8.706187397278121409, 10.29068361123369080, -28.65696959968947866 ) ) ;
#20620=PRESENTATION_STYLE_ASSIGNMENT (( #54014 ) ) ;
#20670=DIRECTION ( 'NONE',  ( 0.000000000000000000, 0.000000000000000000, 1.000000000000000000 ) ) ;
#20679=VECTOR ( 'NONE', #21405, 1000.000000000000000 ) ;
#20704=CARTESIAN_POINT ( 'NONE',  ( -0.000000000000000000, 22.27000000000000668, 0.000000000000000000 ) ) ;
#20733=DIRECTION ( 'NONE',  ( -1.000000000000000000, 0.000000000000000000, 0.000000000000000000 ) ) ;
#20823=ORIENTED_EDGE ( 'NONE', *, *, #56935, .F. ) ;
#20838=VECTOR ( 'NONE', #133510, 1000.000000000000000 ) ;
#20947=CARTESIAN_POINT ( 'NONE',  ( 19.86926087748564740, -2.706703797573569936, -33.83166409453657764 ) ) ;
#21014=ORIENTED_EDGE ( 'NONE', *, *, #135866, .T. ) ;
#21027=DIRECTION ( 'NONE',  ( -1.000000000000000000, 1.248002500702738701E-15, 0.000000000000000000 ) ) ;
#21050=AXIS2_PLACEMENT_3D ( 'NONE', #45340, #101821, #133747 ) ;
#21055=LINE ( 'NONE', #10179, #41818 ) ;
#21058=ORIENTED_EDGE ( 'NONE', *, *, #437, .F. ) ;
#21059=CARTESIAN_POINT ( 'NONE',  ( 7.578844083866184356, 10.86561545741349377, -28.20638205426730138 ) ) ;
#21068=VERTEX_POINT ( 'NONE', #129971 ) ;
#21073=MECHANICAL_DESIGN_GEOMETRIC_PRESENTATION_REPRESENTATION('',(#83723),#41998);
#21084=AXIS2_PLACEMENT_3D ( 'NONE', #101714, #82840, #80700 ) ;
#21119=VECTOR ( 'NONE', #87355, 1000.000000000000000 ) ;
#21121=CARTESIAN_POINT ( 'NONE',  ( 1.953608656376216022E-15, -6.270000000000002238, -40.00000000000000000 ) ) ;
#21139=CARTESIAN_POINT ( 'NONE',  ( 12.19999999999999574, -59.76999999999998892, -39.50000000000000000 ) ) ;
#21150=( LENGTH_UNIT ( ) NAMED_UNIT ( * ) SI_UNIT ( .MILLI., .METRE. ) );
#21151=LINE ( 'NONE', #66112, #6536 ) ;
#21155=STYLED_ITEM ( 'NONE', ( #28915 ), #129368 ) ;
#21162=ORIENTED_EDGE ( 'NONE', *, *, #127854, .T. ) ;
#21215=DIRECTION ( 'NONE',  ( -1.000000000000000000, -3.115803279706882722E-16, -0.000000000000000000 ) ) ;
#21217=( LENGTH_UNIT ( ) NAMED_UNIT ( * ) SI_UNIT ( .MILLI., .METRE. ) );
#21239=ADVANCED_FACE ( 'NONE', ( #11722 ), #86223, .T. ) ;
#21245=FACE_OUTER_BOUND ( 'NONE', #16314, .T. ) ;
#21302=MECHANICAL_DESIGN_GEOMETRIC_PRESENTATION_REPRESENTATION('',(#51425),#58399);
#21304=ORIENTED_EDGE ( 'NONE', *, *, #57517, .T. ) ;
#21315=EDGE_LOOP ( 'NONE', ( #121607, #8102, #124009, #109492, #56336, #13819, #34981, #37441, #114223, #79966, #7146, #84160, #52749, #44165, #61796, #143284, #91928, #140214, #88445, #47978 ) ) ;
#21342=CARTESIAN_POINT ( 'NONE',  ( 12.69999999999999574, -22.33999999999998565, 3.000000000000000000 ) ) ;
#21351=CARTESIAN_POINT ( 'NONE',  ( 10.20209588485037777, 11.26426916695988467, -26.13888605657682973 ) ) ;
#21405=DIRECTION ( 'NONE',  ( 1.369518533665900312E-16, -1.000000000000000000, 0.000000000000000000 ) ) ;
#21413=FACE_OUTER_BOUND ( 'NONE', #62760, .T. ) ;
#21467=FILL_AREA_STYLE_COLOUR ( '', #77905 ) ;
#21481=STYLED_ITEM ( 'NONE', ( #29791 ), #66477 ) ;
#21564=AXIS2_PLACEMENT_3D ( 'NONE', #102882, #3521, #14440 ) ;
#21575=DIRECTION ( 'NONE',  ( -1.000000000000000000, 0.000000000000000000, 0.000000000000000000 ) ) ;
#21578=LINE ( 'NONE', #110681, #22124 ) ;
#21607=ORIENTED_EDGE ( 'NONE', *, *, #1098, .T. ) ;
#21611=FACE_OUTER_BOUND ( 'NONE', #65732, .T. ) ;
#21626=LINE ( 'NONE', #33258, #1608 ) ;
#21718=DIRECTION ( 'NONE',  ( 0.000000000000000000, 1.000000000000000000, 0.000000000000000000 ) ) ;
#21801=( BOUNDED_CURVE ( )  B_SPLINE_CURVE ( 3, ( #73265, #106551, #9370, #7236 ),
 .UNSPECIFIED., .F., .T. ) 
 B_SPLINE_CURVE_WITH_KNOTS ( ( 4, 4 ),
 ( 1.570796326794895892, 1.837133570649240211 ),
 .UNSPECIFIED. ) 
 CURVE ( )  GEOMETRIC_REPRESENTATION_ITEM ( )  RATIONAL_B_SPLINE_CURVE ( ( 1.000000000000000000, 0.9940974367313470950, 0.9940974367313470950, 1.000000000000000000 ) ) 
 REPRESENTATION_ITEM ( '' )  );
#21858=SPHERICAL_SURFACE ( 'NONE', #30645, 0.5000000000000000000 ) ;
#21929=ORIENTED_EDGE ( 'NONE', *, *, #26645, .T. ) ;
#21994=ORIENTED_EDGE ( 'NONE', *, *, #54527, .F. ) ;
#22001=CARTESIAN_POINT ( 'NONE',  ( -7.140000000000001457, -35.76999999999998892, -7.899272885403731514 ) ) ;
#22064=DIRECTION ( 'NONE',  ( 0.000000000000000000, 0.000000000000000000, 1.000000000000000000 ) ) ;
#22073=VERTEX_POINT ( 'NONE', #131435 ) ;
#22077=CARTESIAN_POINT ( 'NONE',  ( -34.92499999999997584, 2.729999999999987104, -36.39086428169088094 ) ) ;
#22113=EDGE_CURVE ( 'NONE', #3531, #36808, #66186, .T. ) ;
#22124=VECTOR ( 'NONE', #131052, 1000.000000000000000 ) ;
#22146=VERTEX_POINT ( 'NONE', #124119 ) ;
#22152=CARTESIAN_POINT ( 'NONE',  ( -31.92499999999997584, 2.729999999999987104, -36.39086428169088094 ) ) ;
#22178=COLOUR_RGB ( '', 0.09019608, 0.27058824, 0.51372549) ;
#22184=DIRECTION ( 'NONE',  ( 3.071323233543530392E-32, -2.242629915582283412E-16, 1.000000000000000000 ) ) ;
#22233=CARTESIAN_POINT ( 'NONE',  ( -34.92499999999999005, 1.196650378695320427, -30.59010235425025215 ) ) ;
#22293=PLANE ( 'NONE',  #104847 ) ;
#22294=DIRECTION ( 'NONE',  ( 0.000000000000000000, 0.000000000000000000, 1.000000000000000000 ) ) ;
#22367=DIRECTION ( 'NONE',  ( -1.000000000000000000, -1.369518533665900312E-16, 0.000000000000000000 ) ) ;
#22395=EDGE_LOOP ( 'NONE', ( #28654, #31700, #49735, #105031 ) ) ;
#22415=CARTESIAN_POINT ( 'NONE',  ( 16.78952603566995805, -0.07140279771002741582, -34.10863443292984698 ) ) ;
#22436=DIRECTION ( 'NONE',  ( 0.000000000000000000, 0.000000000000000000, -1.000000000000000000 ) ) ;
#22447=CONICAL_SURFACE ( 'NONE', #8557, 1.898649999999993065, 1.029744258676648316 ) ;
#22483=DIRECTION ( 'NONE',  ( 0.000000000000000000, 0.2631995976047524777, 0.9647414015272156584 ) ) ;
#22505=EDGE_CURVE ( 'NONE', #7925, #13538, #21055, .T. ) ;
#22506=VERTEX_POINT ( 'NONE', #98617 ) ;
#22518=EDGE_CURVE ( 'NONE', #14912, #36342, #24667, .T. ) ;
#22528=DIRECTION ( 'NONE',  ( -0.000000000000000000, -1.000000000000000000, -0.000000000000000000 ) ) ;
#22591=CARTESIAN_POINT ( 'NONE',  ( -19.05499999999999261, 3.130000000000007887, -2.396719511207313368E-16 ) ) ;
#22603=ORIENTED_EDGE ( 'NONE', *, *, #128025, .F. ) ;
#22620=FILL_AREA_STYLE ('',( #43003 ) ) ;
#22656=FILL_AREA_STYLE_COLOUR ( '', #141646 ) ;
#22681=CARTESIAN_POINT ( 'NONE',  ( 33.97743759385590323, 22.27000000000000668, -13.09127955744558847 ) ) ;
#22705=DIRECTION ( 'NONE',  ( 0.000000000000000000, -1.000000000000000000, 0.000000000000000000 ) ) ;
#22714=FACE_OUTER_BOUND ( 'NONE', #60543, .T. ) ;
#22719=CARTESIAN_POINT ( 'NONE',  ( 0.000000000000000000, -22.26999999999999247, -40.00000000000000000 ) ) ;
#22753=DIRECTION ( 'NONE',  ( 1.000000000000000000, 0.000000000000000000, -0.000000000000000000 ) ) ;
#22798=UNCERTAINTY_MEASURE_WITH_UNIT (LENGTH_MEASURE( 1.000000000000000082E-05 ), #9007, 'distance_accuracy_value', 'NONE');
#22816=DIRECTION ( 'NONE',  ( 1.000000000000000000, 0.000000000000000000, 0.000000000000000000 ) ) ;
#22822=AXIS2_PLACEMENT_3D ( 'NONE', #57443, #37085, #2279 ) ;
#22854=DIRECTION ( 'NONE',  ( 0.000000000000000000, 1.000000000000000000, -0.000000000000000000 ) ) ;
#22855=CARTESIAN_POINT ( 'NONE',  ( -17.54957349083946383, -3.269999989306286547, -35.77884719040818595 ) ) ;
#22883=CARTESIAN_POINT ( 'NONE',  ( -1.256362331258242971E-13, -34.64999999999997726, 17.49210858042621908 ) ) ;
#22890=EDGE_CURVE ( 'NONE', #97358, #50924, #9494, .T. ) ;
#22905=DIRECTION ( 'NONE',  ( 0.000000000000000000, 0.000000000000000000, 1.000000000000000000 ) ) ;
#22925=CIRCLE ( 'NONE', #76269, 2.999999999999999556 ) ;
#22933=AXIS2_PLACEMENT_3D ( 'NONE', #4708, #62034, #27222 ) ;
#22957=CARTESIAN_POINT ( 'NONE',  ( 19.80437226529636163, -2.191939191560713152, -32.94353395994160394 ) ) ;
#23002=SURFACE_STYLE_FILL_AREA ( #11410 ) ;
#23055=EDGE_CURVE ( 'NONE', #75784, #20082, #104404, .T. ) ;
#23082=DIRECTION ( 'NONE',  ( 1.000000000000000000, 0.000000000000000000, 0.000000000000000000 ) ) ;
#23089=ORIENTED_EDGE ( 'NONE', *, *, #79689, .F. ) ;
#23095=AXIS2_PLACEMENT_3D ( 'NONE', #27592, #116024, #72599 ) ;
#23103=DIRECTION ( 'NONE',  ( 1.000000000000000000, 0.000000000000000000, 0.000000000000000000 ) ) ;
#23146=UNCERTAINTY_MEASURE_WITH_UNIT (LENGTH_MEASURE( 1.000000000000000082E-05 ), #105479, 'distance_accuracy_value', 'NONE');
#23152=COLOUR_RGB ( '', 0.66274510, 0.83137255, 0.94901961) ;
#23252=CARTESIAN_POINT ( 'NONE',  ( -7.140000000000001457, -60.26999999999998892, -12.10072711459627293 ) ) ;
#23325=CARTESIAN_POINT ( 'NONE',  ( 2.602316007518551189, 13.59879521490819165, -24.48217750605332910 ) ) ;
#23359=ORIENTED_EDGE ( 'NONE', *, *, #79504, .T. ) ;
#23395=DIRECTION ( 'NONE',  ( -1.000000000000000000, -0.000000000000000000, -0.000000000000000000 ) ) ;
#23397=FILL_AREA_STYLE ('',( #22656 ) ) ;
#23406=CARTESIAN_POINT ( 'NONE',  ( -16.50229999999999819, 3.130000000000007887, 0.000000000000000000 ) ) ;
#23420=( LENGTH_UNIT ( ) NAMED_UNIT ( * ) SI_UNIT ( .MILLI., .METRE. ) );
#23423=VECTOR ( 'NONE', #106904, 1000.000000000000000 ) ;
#23483=CARTESIAN_POINT ( 'NONE',  ( 19.28515664589288292, 1.196650378695338635, -30.59010235425024860 ) ) ;
#23497=SURFACE_SIDE_STYLE ('',( #14034 ) ) ;
#23538=ORIENTED_EDGE ( 'NONE', *, *, #102250, .F. ) ;
#23539=( GEOMETRIC_REPRESENTATION_CONTEXT ( 3 ) GLOBAL_UNCERTAINTY_ASSIGNED_CONTEXT ( ( #25863 ) ) GLOBAL_UNIT_ASSIGNED_CONTEXT ( ( #97692, #20113, #86115 ) ) REPRESENTATION_CONTEXT ( 'NONE', 'WORKASPACE' ) );
#23560=DIRECTION ( 'NONE',  ( 2.496005001405478586E-15, 1.000000000000000000, -0.000000000000000000 ) ) ;
#23604=CARTESIAN_POINT ( 'NONE',  ( -19.93618820135884562, -3.270000000000008900, -36.39086428169088094 ) ) ;
#23711=CARTESIAN_POINT ( 'NONE',  ( 16.73810023419144954, 0.1001526995030668499, -33.96747071225524905 ) ) ;
#23736=VECTOR ( 'NONE', #104276, 1000.000000000000000 ) ;
#23738=AXIS2_PLACEMENT_3D ( 'NONE', #143487, #121021, #21718 ) ;
#23786=CIRCLE ( 'NONE', #46914, 2.999999999999999112 ) ;
#23832=COLOUR_RGB ( '', 0.31764706, 0.68627451, 0.89019608) ;
#23834=CARTESIAN_POINT ( 'NONE',  ( 6.639999999999984581, -40.29840020119762301, 19.55137198191483350 ) ) ;
#23883=ORIENTED_EDGE ( 'NONE', *, *, #122040, .F. ) ;
#23962=VERTEX_POINT ( 'NONE', #105753 ) ;
#23982=DIRECTION ( 'NONE',  ( 0.000000000000000000, 0.9647414015272168797, -0.2631995976047484254 ) ) ;
#23998=VERTEX_POINT ( 'NONE', #141257 ) ;
#24068=CARTESIAN_POINT ( 'NONE',  ( 17.69516080050994589, 4.375290223488867980, -29.58855600362791449 ) ) ;
#24131=DIRECTION ( 'NONE',  ( 0.000000000000000000, 0.000000000000000000, 1.000000000000000000 ) ) ;
#24133=( LENGTH_UNIT ( ) NAMED_UNIT ( * ) SI_UNIT ( .MILLI., .METRE. ) );
#24155=CARTESIAN_POINT ( 'NONE',  ( 34.89822658805448441, 22.27000000000000668, -9.118343482381657594 ) ) ;
#24171=AXIS2_PLACEMENT_3D ( 'NONE', #137960, #113320, #92280 ) ;
#24192=CARTESIAN_POINT ( 'NONE',  ( 6.874395825605885690, -40.07226884389044130, 19.48967909493512352 ) ) ;
#24227=( NAMED_UNIT ( * ) PLANE_ANGLE_UNIT ( ) SI_UNIT ( $, .RADIAN. ) );
#24261=ORIENTED_EDGE ( 'NONE', *, *, #99136, .F. ) ;
#24263=DIRECTION ( 'NONE',  ( 0.000000000000000000, 0.000000000000000000, 1.000000000000000000 ) ) ;
#24310=CIRCLE ( 'NONE', #126239, 0.5000000000000004441 ) ;
#24322=CARTESIAN_POINT ( 'NONE',  ( -16.77039577548053728, -0.01029060706347190504, -34.06785180161139692 ) ) ;
#24337=ORIENTED_EDGE ( 'NONE', *, *, #88831, .T. ) ;
#24363=ORIENTED_EDGE ( 'NONE', *, *, #101901, .T. ) ;
#24427=EDGE_CURVE ( 'NONE', #87614, #51304, #83959, .T. ) ;
#24459=DIRECTION ( 'NONE',  ( 0.000000000000000000, -1.000000000000000000, 0.000000000000000000 ) ) ;
#24465=DIRECTION ( 'NONE',  ( -1.000000000000000000, 0.000000000000000000, 0.000000000000000000 ) ) ;
#24492=ORIENTED_EDGE ( 'NONE', *, *, #60227, .T. ) ;
#24546=FACE_OUTER_BOUND ( 'NONE', #62524, .T. ) ;
#24611=CARTESIAN_POINT ( 'NONE',  ( -8.648657329869978142E-14, -34.64999999999997726, -39.50000000000000000 ) ) ;
#24635=EDGE_CURVE ( 'NONE', #61603, #135652, #11998, .T. ) ;
#24650=SURFACE_STYLE_FILL_AREA ( #34841 ) ;
#24667=B_SPLINE_CURVE_WITH_KNOTS ( 'NONE', 3,
 ( #48532, #81178, #134128, #113056 ),
 .UNSPECIFIED., .F., .F.,
 ( 4, 4 ),
 ( 0.001163520961193752548, 0.001596196080316615801 ),
 .UNSPECIFIED. ) ;
#24711=FILL_AREA_STYLE_COLOUR ( '', #95401 ) ;
#24715=DIRECTION ( 'NONE',  ( 1.000000000000000000, 3.115803279706882722E-16, 0.000000000000000000 ) ) ;
#24727=FACE_OUTER_BOUND ( 'NONE', #15466, .T. ) ;
#24769=CARTESIAN_POINT ( 'NONE',  ( 7.166003870700648370, 12.55858695562843330, -25.25459431962041634 ) ) ;
#24836=CARTESIAN_POINT ( 'NONE',  ( 21.59770000000000678, 3.130000000000007887, -2.396719511207313368E-16 ) ) ;
#24869=CARTESIAN_POINT ( 'NONE',  ( 34.42500000000002558, -22.26999999999999247, -37.00000000000000000 ) ) ;
#24908=ORIENTED_EDGE ( 'NONE', *, *, #113493, .F. ) ;
#24910=DIRECTION ( 'NONE',  ( -0.000000000000000000, 0.000000000000000000, 1.000000000000000000 ) ) ;
#24925=CARTESIAN_POINT ( 'NONE',  ( 34.92500000000002558, -21.76999999999999247, -37.00000000000000000 ) ) ;
#24973=ADVANCED_FACE ( 'NONE', ( #45229 ), #132947, .T. ) ;
#24986=AXIS2_PLACEMENT_3D ( 'NONE', #59197, #103351, #3999 ) ;
#25013=VERTEX_POINT ( 'NONE', #17539 ) ;
#25015=SURFACE_SIDE_STYLE ('',( #1116 ) ) ;
#25036=ORIENTED_EDGE ( 'NONE', *, *, #61925, .T. ) ;
#25054=VERTEX_POINT ( 'NONE', #105273 ) ;
#25119=CARTESIAN_POINT ( 'NONE',  ( 16.95443293193746115, -0.6982307342378247794, -35.09649380009672370 ) ) ;
#25122=( GEOMETRIC_REPRESENTATION_CONTEXT ( 3 ) GLOBAL_UNCERTAINTY_ASSIGNED_CONTEXT ( ( #48891 ) ) GLOBAL_UNIT_ASSIGNED_CONTEXT ( ( #35470, #99978, #66641 ) ) REPRESENTATION_CONTEXT ( 'NONE', 'WORKASPACE' ) );
#25165=CARTESIAN_POINT ( 'NONE',  ( -7.940000000000001279, -35.14999999999999147, -10.00000000000000178 ) ) ;
#25167=ADVANCED_FACE ( 'NONE', ( #68591 ), #65551, .T. ) ;
#25208=STYLED_ITEM ( 'NONE', ( #111796 ), #139027 ) ;
#25219=CONICAL_SURFACE ( 'NONE', #36812, 9.524999999999991473, 1.029744258676653645 ) ;
#25220=CIRCLE ( 'NONE', #48311, 1.898649999999994842 ) ;
#25251=DIRECTION ( 'NONE',  ( 0.000000000000000000, 0.000000000000000000, -1.000000000000000000 ) ) ;
#25253=PRESENTATION_STYLE_ASSIGNMENT (( #100159 ) ) ;
#25306=DIRECTION ( 'NONE',  ( -0.000000000000000000, -1.000000000000000000, -0.000000000000000000 ) ) ;
#25366=EDGE_LOOP ( 'NONE', ( #30790, #108634, #93827, #1980 ) ) ;
#25413=DIRECTION ( 'NONE',  ( 0.000000000000000000, -0.000000000000000000, -1.000000000000000000 ) ) ;
#25453=CARTESIAN_POINT ( 'NONE',  ( -12.20000000000000284, -27.55040120718572894, 16.07347811296898854 ) ) ;
#25468=CARTESIAN_POINT ( 'NONE',  ( 2.075939324931954655, 13.65470463357565123, -24.43886132094158725 ) ) ;
#25481=LINE ( 'NONE', #124101, #58694 ) ;
#25569=EDGE_LOOP ( 'NONE', ( #46349, #47449, #33898, #103692, #24337, #45344, #109041, #129441 ) ) ;
#25591=AXIS2_PLACEMENT_3D ( 'NONE', #78213, #134015, #91246 ) ;
#25601=CIRCLE ( 'NONE', #11716, 0.5000000000000004441 ) ;
#25605=CARTESIAN_POINT ( 'NONE',  ( 7.940000000000001279, -33.26999999999999602, -10.00000000000000178 ) ) ;
#25665=CARTESIAN_POINT ( 'NONE',  ( -7.940000000000007496, -60.26999999999998892, -7.752100000000004876 ) ) ;
#25706=FACE_OUTER_BOUND ( 'NONE', #67787, .T. ) ;
#25715=( GEOMETRIC_REPRESENTATION_CONTEXT ( 3 ) GLOBAL_UNCERTAINTY_ASSIGNED_CONTEXT ( ( #38863 ) ) GLOBAL_UNIT_ASSIGNED_CONTEXT ( ( #142435, #77195, #80058 ) ) REPRESENTATION_CONTEXT ( 'NONE', 'WORKASPACE' ) );
#25744=FILL_AREA_STYLE_COLOUR ( '', #111523 ) ;
#25771=( NAMED_UNIT ( * ) PLANE_ANGLE_UNIT ( ) SI_UNIT ( $, .RADIAN. ) );
#25778=CARTESIAN_POINT ( 'NONE',  ( -12.70000000000000284, -34.64999999999999147, -39.50000000000000000 ) ) ;
#25816=ADVANCED_FACE ( 'NONE', ( #3799 ), #16116, .F. ) ;
#25826=DIRECTION ( 'NONE',  ( 0.000000000000000000, 0.000000000000000000, 1.000000000000000000 ) ) ;
#25863=UNCERTAINTY_MEASURE_WITH_UNIT (LENGTH_MEASURE( 1.000000000000000082E-05 ), #97692, 'distance_accuracy_value', 'NONE');
#25883=ORIENTED_EDGE ( 'NONE', *, *, #9743, .F. ) ;
#25909=VERTEX_POINT ( 'NONE', #6654 ) ;
#25919=AXIS2_PLACEMENT_3D ( 'NONE', #129041, #38480, #52197 ) ;
#25933=MECHANICAL_DESIGN_GEOMETRIC_PRESENTATION_REPRESENTATION('',(#83915),#100031);
#25972=( GEOMETRIC_REPRESENTATION_CONTEXT ( 3 ) GLOBAL_UNCERTAINTY_ASSIGNED_CONTEXT ( ( #5680 ) ) GLOBAL_UNIT_ASSIGNED_CONTEXT ( ( #58105, #27548, #2207 ) ) REPRESENTATION_CONTEXT ( 'NONE', 'WORKASPACE' ) );
#26031=AXIS2_PLACEMENT_3D ( 'NONE', #28412, #51598, #38567 ) ;
#26034=CYLINDRICAL_SURFACE ( 'NONE', #21564, 0.5000000000000004441 ) ;
#26066=EDGE_CURVE ( 'NONE', #113921, #118671, #89956, .T. ) ;
#26079=ADVANCED_FACE ( 'NONE', ( #109581 ), #21858, .T. ) ;
#26107=DIRECTION ( 'NONE',  ( -0.000000000000000000, -0.000000000000000000, 1.000000000000000000 ) ) ;
#26119=ORIENTED_EDGE ( 'NONE', *, *, #48279, .F. ) ;
#26149=ADVANCED_FACE ( 'NONE', ( #13807 ), #47935, .F. ) ;
#26158=( NAMED_UNIT ( * ) SI_UNIT ( $, .STERADIAN. ) SOLID_ANGLE_UNIT ( ) );
#26159=SURFACE_STYLE_FILL_AREA ( #116726 ) ;
#26167=ORIENTED_EDGE ( 'NONE', *, *, #120535, .F. ) ;
#26177=LINE ( 'NONE', #58127, #118165 ) ;
#26221=LINE ( 'NONE', #93619, #79099 ) ;
#26259=CARTESIAN_POINT ( 'NONE',  ( 16.49230000000001439, 3.130000000000008331, 0.000000000000000000 ) ) ;
#26269=VECTOR ( 'NONE', #113513, 1000.000000000000000 ) ;
#26280=CARTESIAN_POINT ( 'NONE',  ( 19.04500000000000881, 3.130000000000007887, 0.000000000000000000 ) ) ;
#26352=CIRCLE ( 'NONE', #63433, 2.247899999999998677 ) ;
#26405=COLOUR_RGB ( '', 0.09019608, 0.27058824, 0.51372549) ;
#26443=ADVANCED_FACE ( 'NONE', ( #131890 ), #44928, .T. ) ;
#26494=CONICAL_SURFACE ( 'NONE', #63479, 2.552699999999994418, 1.029744258676651869 ) ;
#26502=LINE ( 'NONE', #37382, #43847 ) ;
#26504=ORIENTED_EDGE ( 'NONE', *, *, #38426, .T. ) ;
#26510=ADVANCED_FACE ( 'NONE', ( #15079 ), #137606, .F. ) ;
#26517=CARTESIAN_POINT ( 'NONE',  ( -14.95063623912963635, 4.191486776496043731, -32.28758159997615707 ) ) ;
#26573=DIRECTION ( 'NONE',  ( 0.000000000000000000, 0.2631995976047524777, 0.9647414015272156584 ) ) ;
#26645=EDGE_CURVE ( 'NONE', #61603, #70779, #129249, .T. ) ;
#26661=CIRCLE ( 'NONE', #40550, 1.898649999999994842 ) ;
#26681=CYLINDRICAL_SURFACE ( 'NONE', #134536, 3.000000000000000000 ) ;
#26692=PLANE ( 'NONE',  #88026 ) ;
#26710=EDGE_LOOP ( 'NONE', ( #136361, #88038, #67651, #139676 ) ) ;
#26852=SURFACE_STYLE_FILL_AREA ( #38456 ) ;
#26912=CARTESIAN_POINT ( 'NONE',  ( 0.4878811198072842137, 13.74641354151631134, -24.36756908848417780 ) ) ;
#26913=CARTESIAN_POINT ( 'NONE',  ( 0.000000000000000000, -4.870000000000014317, -10.00000000000000178 ) ) ;
#26927=( NAMED_UNIT ( * ) SI_UNIT ( $, .STERADIAN. ) SOLID_ANGLE_UNIT ( ) );
#26945=CARTESIAN_POINT ( 'NONE',  ( -14.48042995505719510, 4.924559884198918880, -31.94719639125090538 ) ) ;
#27006=FILL_AREA_STYLE_COLOUR ( '', #109026 ) ;
#27041=DIRECTION ( 'NONE',  ( 1.000000000000000000, 0.000000000000000000, 0.000000000000000000 ) ) ;
#27046=ORIENTED_EDGE ( 'NONE', *, *, #74309, .T. ) ;
#27146=CARTESIAN_POINT ( 'NONE',  ( -16.78948154309660268, -0.07126238382044708386, -34.10854881514017478 ) ) ;
#27156=DIRECTION ( 'NONE',  ( 1.000000000000000000, 0.000000000000000000, 0.000000000000000000 ) ) ;
#27212=CARTESIAN_POINT ( 'NONE',  ( -13.03876099366718400, 6.774379884391048101, -28.62998901354190195 ) ) ;
#27222=DIRECTION ( 'NONE',  ( 0.000000000000000000, 0.000000000000000000, -1.000000000000000000 ) ) ;
#27229=ORIENTED_EDGE ( 'NONE', *, *, #83980, .T. ) ;
#27250=UNCERTAINTY_MEASURE_WITH_UNIT (LENGTH_MEASURE( 1.000000000000000082E-05 ), #109529, 'distance_accuracy_value', 'NONE');
#27259=CARTESIAN_POINT ( 'NONE',  ( -12.20000000000000284, -28.33999999999998565, 13.17925390838734323 ) ) ;
#27263=CARTESIAN_POINT ( 'NONE',  ( 19.93618820135884917, -3.269999999999996909, -36.39086428169088094 ) ) ;
#27267=CARTESIAN_POINT ( 'NONE',  ( 7.940000000000001279, -35.14999999999999858, -11.89864999999999640 ) ) ;
#27310=CARTESIAN_POINT ( 'NONE',  ( 0.000000000000000000, -21.76999999999999247, 0.000000000000000000 ) ) ;
#27319=CARTESIAN_POINT ( 'NONE',  ( 12.19999999999999574, -39.93000000000000682, -39.50000000000000000 ) ) ;
#27339=EDGE_CURVE ( 'NONE', #71183, #116824, #26177, .T. ) ;
#27370=SURFACE_SIDE_STYLE ('',( #126687 ) ) ;
#27431=ORIENTED_EDGE ( 'NONE', *, *, #102563, .F. ) ;
#27488=ORIENTED_EDGE ( 'NONE', *, *, #36918, .T. ) ;
#27507=CARTESIAN_POINT ( 'NONE',  ( 1.953608656376216022E-15, -6.270000000000002238, -40.00000000000000000 ) ) ;
#27548=( NAMED_UNIT ( * ) PLANE_ANGLE_UNIT ( ) SI_UNIT ( $, .RADIAN. ) );
#27551=PLANE ( 'NONE',  #50603 ) ;
#27592=CARTESIAN_POINT ( 'NONE',  ( 7.140000000000044089, -1.036479131253094653E-14, -40.00000000000000000 ) ) ;
#27615=CARTESIAN_POINT ( 'NONE',  ( -15.56688804974254126, 7.140284830960222706, -28.42913291040909840 ) ) ;
#27679=CARTESIAN_POINT ( 'NONE',  ( -12.20000000000000284, -34.64999999999999147, -39.50000000000000000 ) ) ;
#27732=CARTESIAN_POINT ( 'NONE',  ( -6.997731156109542106, -34.88439582560590679, 17.99210858042622974 ) ) ;
#27767=EDGE_CURVE ( 'NONE', #50410, #89049, #88095, .T. ) ;
#27793=( GEOMETRIC_REPRESENTATION_CONTEXT ( 3 ) GLOBAL_UNCERTAINTY_ASSIGNED_CONTEXT ( ( #101253 ) ) GLOBAL_UNIT_ASSIGNED_CONTEXT ( ( #49543, #40785, #137240 ) ) REPRESENTATION_CONTEXT ( 'NONE', 'WORKASPACE' ) );
#27798=DIRECTION ( 'NONE',  ( 0.000000000000000000, -1.000000000000000000, -6.938893903907222067E-15 ) ) ;
#27840=STYLED_ITEM ( 'NONE', ( #52503 ), #41862 ) ;
#27878=ORIENTED_EDGE ( 'NONE', *, *, #44194, .F. ) ;
#27880=( NAMED_UNIT ( * ) PLANE_ANGLE_UNIT ( ) SI_UNIT ( $, .RADIAN. ) );
#27902=VERTEX_POINT ( 'NONE', #86094 ) ;
#27939=CARTESIAN_POINT ( 'NONE',  ( -13.40214831053034850, 6.329416083240667845, -31.22042670906152040 ) ) ;
#27967=CARTESIAN_POINT ( 'NONE',  ( -7.140000000000001457, -39.92999999999999261, 18.97874025153853239 ) ) ;
#27985=CARTESIAN_POINT ( 'NONE',  ( -7.140000000000001457, -35.14999999999999147, -39.50000000000000000 ) ) ;
#28004=COLOUR_RGB ( '', 0.72549020, 0.75294118, 0.79215686) ;
#28019=DIRECTION ( 'NONE',  ( 0.000000000000000000, 1.000000000000000000, 0.000000000000000000 ) ) ;
#28035=COLOUR_RGB ( '', 0.09019608, 0.27058824, 0.51372549) ;
#28048=CARTESIAN_POINT ( 'NONE',  ( -12.20000000000000284, -34.64999999999999147, 17.49210858042622263 ) ) ;
#28058=AXIS2_PLACEMENT_3D ( 'NONE', #52785, #133252, #132557 ) ;
#28071=ORIENTED_EDGE ( 'NONE', *, *, #121803, .F. ) ;
#28085=CIRCLE ( 'NONE', #116027, 3.000000000000000444 ) ;
#28132=( GEOMETRIC_REPRESENTATION_CONTEXT ( 3 ) GLOBAL_UNCERTAINTY_ASSIGNED_CONTEXT ( ( #134475 ) ) GLOBAL_UNIT_ASSIGNED_CONTEXT ( ( #45802, #99411, #89282 ) ) REPRESENTATION_CONTEXT ( 'NONE', 'WORKASPACE' ) );
#28208=CIRCLE ( 'NONE', #86160, 2.999999999999999112 ) ;
#28209=COLOUR_RGB ( '', 0.08235294, 0.09019608, 0.10196078) ;
#28251=DIRECTION ( 'NONE',  ( -1.000000000000000000, 0.000000000000000000, 0.000000000000000000 ) ) ;
#28255=( GEOMETRIC_REPRESENTATION_CONTEXT ( 3 ) GLOBAL_UNCERTAINTY_ASSIGNED_CONTEXT ( ( #133388 ) ) GLOBAL_UNIT_ASSIGNED_CONTEXT ( ( #5955, #94417, #82860 ) ) REPRESENTATION_CONTEXT ( 'NONE', 'WORKASPACE' ) );
#28297=VECTOR ( 'NONE', #112676, 1000.000000000000000 ) ;
#28319=CARTESIAN_POINT ( 'NONE',  ( -55.65468426143998215, -27.55040120718572894, 16.07347811296898854 ) ) ;
#28366=DIRECTION ( 'NONE',  ( 0.000000000000000000, 0.2631995976047524777, 0.9647414015272156584 ) ) ;
#28393=CARTESIAN_POINT ( 'NONE',  ( -10.95743729084448859, 8.751477814956837520, -29.75791556614341360 ) ) ;
#28412=CARTESIAN_POINT ( 'NONE',  ( -31.92499999999997584, -22.26999999999999247, -37.00000000000000000 ) ) ;
#28429=EDGE_CURVE ( 'NONE', #43110, #22506, #142458, .T. ) ;
#28467=VERTEX_POINT ( 'NONE', #71870 ) ;
#28487=DIRECTION ( 'NONE',  ( -0.000000000000000000, 0.000000000000000000, 1.000000000000000000 ) ) ;
#28501=CARTESIAN_POINT ( 'NONE',  ( 12.19999999999999574, -60.26999999999998892, 25.00000000000000000 ) ) ;
#28606=CARTESIAN_POINT ( 'NONE',  ( -7.940000000000001279, -33.26999999999999602, -11.89864999999999462 ) ) ;
#28613=ADVANCED_FACE ( 'NONE', ( #84181 ), #51534, .T. ) ;
#28642=SURFACE_STYLE_USAGE ( .BOTH. , #107597 ) ;
#28644=ORIENTED_EDGE ( 'NONE', *, *, #100005, .T. ) ;
#28653=EDGE_CURVE ( 'NONE', #19482, #85621, #11898, .T. ) ;
#28654=ORIENTED_EDGE ( 'NONE', *, *, #33903, .F. ) ;
#28677=CARTESIAN_POINT ( 'NONE',  ( -12.12207849854756248, 7.746936202595393617, -28.17582321246111832 ) ) ;
#28712=CARTESIAN_POINT ( 'NONE',  ( -33.98013387480477832, 22.27000000000000313, -13.08571143629930944 ) ) ;
#28730=ORIENTED_EDGE ( 'NONE', *, *, #111668, .F. ) ;
#28731=CARTESIAN_POINT ( 'NONE',  ( -6.640000000000001457, -40.29840020119761590, 19.55137198191482995 ) ) ;
#28751=CARTESIAN_POINT ( 'NONE',  ( 12.19999999999999574, -34.65000000000001279, -40.00000000000000000 ) ) ;
#28827=DIRECTION ( 'NONE',  ( -1.000000000000000000, 0.000000000000000000, 0.000000000000000000 ) ) ;
#28857=DIRECTION ( 'NONE',  ( -1.000000000000000000, 0.000000000000000000, 0.000000000000000000 ) ) ;
#28898=CARTESIAN_POINT ( 'NONE',  ( -12.70000000000000462, -22.26999999999999247, -39.50000000000000000 ) ) ;
#28902=DIRECTION ( 'NONE',  ( 1.248002500702738701E-15, 1.000000000000000000, -0.000000000000000000 ) ) ;
#28915=PRESENTATION_STYLE_ASSIGNMENT (( #6384 ) ) ;
#28991=DIRECTION ( 'NONE',  ( 1.000000000000000000, 0.000000000000000000, 0.000000000000000000 ) ) ;
#29001=DIRECTION ( 'NONE',  ( 0.000000000000000000, -1.000000000000000000, 0.000000000000000000 ) ) ;
#29076=( GEOMETRIC_REPRESENTATION_CONTEXT ( 3 ) GLOBAL_UNCERTAINTY_ASSIGNED_CONTEXT ( ( #134627 ) ) GLOBAL_UNIT_ASSIGNED_CONTEXT ( ( #53307, #131601, #26927 ) ) REPRESENTATION_CONTEXT ( 'NONE', 'WORKASPACE' ) );
#29080=EDGE_CURVE ( 'NONE', #25013, #109867, #5314, .T. ) ;
#29095=ORIENTED_EDGE ( 'NONE', *, *, #44765, .T. ) ;
#29097=FILL_AREA_STYLE ('',( #129114 ) ) ;
#29116=FILL_AREA_STYLE_COLOUR ( '', #32561 ) ;
#29132=DIRECTION ( 'NONE',  ( -0.000000000000000000, -0.000000000000000000, -1.000000000000000000 ) ) ;
#29141=CARTESIAN_POINT ( 'NONE',  ( 7.940000000000001279, -60.26999999999998892, -10.00000000000000178 ) ) ;
#29152=DIRECTION ( 'NONE',  ( 0.000000000000000000, 0.000000000000000000, -1.000000000000000000 ) ) ;
#29243=EDGE_CURVE ( 'NONE', #88659, #1800, #131452, .T. ) ;
#29281=LINE ( 'NONE', #51053, #59321 ) ;
#29320=DIRECTION ( 'NONE',  ( 0.000000000000000000, -0.000000000000000000, -1.000000000000000000 ) ) ;
#29351=CARTESIAN_POINT ( 'NONE',  ( 6.205262656257519716, 11.46168650470408146, -26.04351286206016525 ) ) ;
#29372=DIRECTION ( 'NONE',  ( 0.000000000000000000, 1.000000000000000000, 0.000000000000000000 ) ) ;
#29393=SURFACE_STYLE_FILL_AREA ( #54055 ) ;
#29431=CARTESIAN_POINT ( 'NONE',  ( 12.69999999999999574, -35.15000000000000568, -39.79289321881344677 ) ) ;
#29461=( GEOMETRIC_REPRESENTATION_CONTEXT ( 3 ) GLOBAL_UNCERTAINTY_ASSIGNED_CONTEXT ( ( #35895 ) ) GLOBAL_UNIT_ASSIGNED_CONTEXT ( ( #35580, #112392, #79810 ) ) REPRESENTATION_CONTEXT ( 'NONE', 'WORKASPACE' ) );
#29539=LINE ( 'NONE', #111202, #73299 ) ;
#29543=ORIENTED_EDGE ( 'NONE', *, *, #101901, .F. ) ;
#29545=ORIENTED_EDGE ( 'NONE', *, *, #70339, .T. ) ;
#29593=( NAMED_UNIT ( * ) SI_UNIT ( $, .STERADIAN. ) SOLID_ANGLE_UNIT ( ) );
#29607=FACE_OUTER_BOUND ( 'NONE', #44374, .T. ) ;
#29626=AXIS2_PLACEMENT_3D ( 'NONE', #42218, #65406, #109586 ) ;
#29670=( BOUNDED_CURVE ( )  B_SPLINE_CURVE ( 3, ( #62515, #106683, #128478, #7376 ),
 .UNSPECIFIED., .F., .T. ) 
 B_SPLINE_CURVE_WITH_KNOTS ( ( 4, 4 ),
 ( 3.141592653589793116, 4.712388980384689674 ),
 .UNSPECIFIED. ) 
 CURVE ( )  GEOMETRIC_REPRESENTATION_ITEM ( )  RATIONAL_B_SPLINE_CURVE ( ( 1.000000000000000000, 0.8047378541243649375, 0.8047378541243649375, 1.000000000000000000 ) ) 
 REPRESENTATION_ITEM ( '' )  );
#29691=DIRECTION ( 'NONE',  ( 0.000000000000000000, 0.000000000000000000, -1.000000000000000000 ) ) ;
#29696=DIRECTION ( 'NONE',  ( -0.000000000000000000, -0.000000000000000000, -1.000000000000000000 ) ) ;
#29719=DIRECTION ( 'NONE',  ( -0.000000000000000000, -0.000000000000000000, 1.000000000000000000 ) ) ;
#29735=DIRECTION ( 'NONE',  ( -0.000000000000000000, -0.000000000000000000, 1.000000000000000000 ) ) ;
#29773=ORIENTED_EDGE ( 'NONE', *, *, #92959, .T. ) ;
#29790=CARTESIAN_POINT ( 'NONE',  ( -12.54203964395424009, 7.284662239043824705, -30.67748158611714970 ) ) ;
#29791=PRESENTATION_STYLE_ASSIGNMENT (( #61749 ) ) ;
#29794=AXIS2_PLACEMENT_3D ( 'NONE', #24611, #47151, #57281 ) ;
#29801=DIRECTION ( 'NONE',  ( 6.938893903907221278E-15, -0.000000000000000000, -1.000000000000000000 ) ) ;
#29807=DIRECTION ( 'NONE',  ( -0.000000000000000000, 1.000000000000000000, -0.000000000000000000 ) ) ;
#29832=ORIENTED_EDGE ( 'NONE', *, *, #30345, .T. ) ;
#29992=CIRCLE ( 'NONE', #122607, 9.000000000000001776 ) ;
#30024=( LENGTH_UNIT ( ) NAMED_UNIT ( * ) SI_UNIT ( .MILLI., .METRE. ) );
#30067=CARTESIAN_POINT ( 'NONE',  ( 10.90130741741065101, 8.797424235802401071, -29.72726348083716630 ) ) ;
#30161=CARTESIAN_POINT ( 'NONE',  ( -34.92499999999997584, -6.270000000000012896, -37.00000000000000000 ) ) ;
#30189=PRESENTATION_STYLE_ASSIGNMENT (( #99008 ) ) ;
#30192=AXIS2_PLACEMENT_3D ( 'NONE', #21139, #57371, #797 ) ;
#30260=ORIENTED_EDGE ( 'NONE', *, *, #30376, .F. ) ;
#30279=( NAMED_UNIT ( * ) PLANE_ANGLE_UNIT ( ) SI_UNIT ( $, .RADIAN. ) );
#30338=CYLINDRICAL_SURFACE ( 'NONE', #34869, 17.46000000000000085 ) ;
#30341=VERTEX_POINT ( 'NONE', #864 ) ;
#30345=EDGE_CURVE ( 'NONE', #88659, #46696, #90779, .T. ) ;
#30372=DIRECTION ( 'NONE',  ( -0.000000000000000000, -1.000000000000000000, -0.000000000000000000 ) ) ;
#30374=AXIS2_PLACEMENT_3D ( 'NONE', #90654, #48560, #134151 ) ;
#30376=EDGE_CURVE ( 'NONE', #129025, #135430, #104623, .T. ) ;
#30426=ORIENTED_EDGE ( 'NONE', *, *, #106156, .F. ) ;
#30430=SURFACE_STYLE_USAGE ( .BOTH. , #129722 ) ;
#30445=ORIENTED_EDGE ( 'NONE', *, *, #116835, .T. ) ;
#30487=VECTOR ( 'NONE', #130177, 1000.000000000000000 ) ;
#30490=AXIS2_PLACEMENT_3D ( 'NONE', #45395, #101874, #56982 ) ;
#30515=PRESENTATION_STYLE_ASSIGNMENT (( #129090 ) ) ;
#30529=LINE ( 'NONE', #141414, #127244 ) ;
#30550=CARTESIAN_POINT ( 'NONE',  ( -34.42499999999997584, 22.27000000000000668, -0.5000000000000000000 ) ) ;
#30585=ORIENTED_EDGE ( 'NONE', *, *, #136983, .F. ) ;
#30599=AXIS2_PLACEMENT_3D ( 'NONE', #109727, #95986, #119855 ) ;
#30645=AXIS2_PLACEMENT_3D ( 'NONE', #77690, #88571, #132807 ) ;
#30661=LINE ( 'NONE', #20454, #137514 ) ;
#30713=ORIENTED_EDGE ( 'NONE', *, *, #6966, .F. ) ;
#30790=ORIENTED_EDGE ( 'NONE', *, *, #96919, .F. ) ;
#30811=ORIENTED_EDGE ( 'NONE', *, *, #55753, .T. ) ;
#30823=CARTESIAN_POINT ( 'NONE',  ( -1.027788732625423807, 12.58765678330771287, -25.27074045886576670 ) ) ;
#30875=CARTESIAN_POINT ( 'NONE',  ( -31.92499999999997584, -21.76999999999999247, -37.00000000000000000 ) ) ;
#30893=ORIENTED_EDGE ( 'NONE', *, *, #36598, .F. ) ;
#30974=DIRECTION ( 'NONE',  ( -1.000000000000000000, 0.000000000000000000, 0.000000000000000000 ) ) ;
#31038=EDGE_LOOP ( 'NONE', ( #75847, #70624, #141419, #108708 ) ) ;
#31061=DIRECTION ( 'NONE',  ( -0.000000000000000000, -1.000000000000000000, -0.000000000000000000 ) ) ;
#31078=EDGE_CURVE ( 'NONE', #15191, #97431, #56136, .T. ) ;
#31130=SURFACE_STYLE_FILL_AREA ( #422 ) ;
#31147=( NAMED_UNIT ( * ) SI_UNIT ( $, .STERADIAN. ) SOLID_ANGLE_UNIT ( ) );
#31199=CARTESIAN_POINT ( 'NONE',  ( 34.92500000000001847, 0.4299755680430066840, -27.68972139052992532 ) ) ;
#31295=DIRECTION ( 'NONE',  ( 0.000000000000000000, 0.000000000000000000, -1.000000000000000000 ) ) ;
#31365=VERTEX_POINT ( 'NONE', #60694 ) ;
#31379=EDGE_CURVE ( 'NONE', #88226, #878, #136768, .T. ) ;
#31445=CARTESIAN_POINT ( 'NONE',  ( -12.20000000000000284, -39.92999999999999261, 19.45086547876359617 ) ) ;
#31465=MECHANICAL_DESIGN_GEOMETRIC_PRESENTATION_REPRESENTATION('',(#12908),#123987);
#31471=DIRECTION ( 'NONE',  ( 1.000000000000000000, 0.000000000000000000, 0.000000000000000000 ) ) ;
#31494=CARTESIAN_POINT ( 'NONE',  ( -8.749659869322266218E-15, -4.870000000000014317, -4.276802603762487998 ) ) ;
#31517=CARTESIAN_POINT ( 'NONE',  ( 1.043401249077450688, 13.72784592288353345, -24.38207966554766060 ) ) ;
#31522=SURFACE_SIDE_STYLE ('',( #87333 ) ) ;
#31624=AXIS2_PLACEMENT_3D ( 'NONE', #40259, #17050, #84470 ) ;
#31673=CARTESIAN_POINT ( 'NONE',  ( -12.70000000000000462, -25.83999999999998920, 13.17925390838734323 ) ) ;
#31700=ORIENTED_EDGE ( 'NONE', *, *, #96700, .T. ) ;
#31739=EDGE_LOOP ( 'NONE', ( #63390, #137905, #21162, #122832, #137588, #32569, #94330, #7131 ) ) ;
#31744=ORIENTED_EDGE ( 'NONE', *, *, #35215, .T. ) ;
#31745=SURFACE_STYLE_FILL_AREA ( #95561 ) ;
#31759=DIRECTION ( 'NONE',  ( 0.000000000000000000, -0.2555582702174447052, 0.9667936545734397980 ) ) ;
#31797=CIRCLE ( 'NONE', #52583, 2.247900000000000453 ) ;
#31825=ORIENTED_EDGE ( 'NONE', *, *, #106755, .T. ) ;
#31855=DIRECTION ( 'NONE',  ( 0.9425785261922230429, 0.3339846133601018230, 0.000000000000000000 ) ) ;
#31859=CARTESIAN_POINT ( 'NONE',  ( 12.19999999999999574, 0.000000000000000000, -0.5000000000000004441 ) ) ;
#31919=UNCERTAINTY_MEASURE_WITH_UNIT (LENGTH_MEASURE( 1.000000000000000082E-05 ), #61810, 'distance_accuracy_value', 'NONE');
#31923=EDGE_CURVE ( 'NONE', #50924, #103756, #77138, .T. ) ;
#31935=ORIENTED_EDGE ( 'NONE', *, *, #38426, .F. ) ;
#31971=FACE_OUTER_BOUND ( 'NONE', #105404, .T. ) ;
#31976=AXIS2_PLACEMENT_3D ( 'NONE', #132859, #121925, #142985 ) ;
#31986=( BOUNDED_CURVE ( )  B_SPLINE_CURVE ( 3, ( #85753, #63341, #142310, #61901 ),
 .UNSPECIFIED., .F., .T. ) 
 B_SPLINE_CURVE_WITH_KNOTS ( ( 4, 4 ),
 ( 1.570796326794896558, 3.141592653589793116 ),
 .UNSPECIFIED. ) 
 CURVE ( )  GEOMETRIC_REPRESENTATION_ITEM ( )  RATIONAL_B_SPLINE_CURVE ( ( 1.000000000000000000, 0.8047378541243649375, 0.8047378541243649375, 1.000000000000000000 ) ) 
 REPRESENTATION_ITEM ( '' )  );
#32022=ORIENTED_EDGE ( 'NONE', *, *, #130561, .F. ) ;
#32031=FILL_AREA_STYLE ('',( #140102 ) ) ;
#32067=DIRECTION ( 'NONE',  ( -0.000000000000000000, -0.000000000000000000, -1.000000000000000000 ) ) ;
#32230=CARTESIAN_POINT ( 'NONE',  ( -5.385325943209082311, 13.08800193907929277, -24.86884355624839316 ) ) ;
#32287=CARTESIAN_POINT ( 'NONE',  ( -34.42499999999997584, -22.26999999999999247, -37.00000000000000000 ) ) ;
#32290=VERTEX_POINT ( 'NONE', #71736 ) ;
#32298=EDGE_CURVE ( 'NONE', #113508, #36808, #53953, .T. ) ;
#32346=FILL_AREA_STYLE ('',( #21467 ) ) ;
#32391=FACE_OUTER_BOUND ( 'NONE', #82290, .T. ) ;
#32407=CYLINDRICAL_SURFACE ( 'NONE', #53488, 0.5000000000000004441 ) ;
#32461=AXIS2_PLACEMENT_3D ( 'NONE', #127801, #28487, #132812 ) ;
#32495=CYLINDRICAL_SURFACE ( 'NONE', #51608, 2.552699999999994418 ) ;
#32509=FILL_AREA_STYLE ('',( #44101 ) ) ;
#32540=ADVANCED_FACE ( 'NONE', ( #77458 ), #101314, .F. ) ;
#32561=COLOUR_RGB ( '', 0.08235294, 0.09019608, 0.10196078) ;
#32569=ORIENTED_EDGE ( 'NONE', *, *, #100950, .F. ) ;
#32574=ORIENTED_EDGE ( 'NONE', *, *, #72661, .F. ) ;
#32591=PRESENTATION_STYLE_ASSIGNMENT (( #76826 ) ) ;
#32631=ORIENTED_EDGE ( 'NONE', *, *, #122212, .F. ) ;
#32633=PRESENTATION_STYLE_ASSIGNMENT (( #143510 ) ) ;
#32685=CARTESIAN_POINT ( 'NONE',  ( 15.15628408943919858, 3.809557873852078114, -32.44464145375744835 ) ) ;
#32691=CARTESIAN_POINT ( 'NONE',  ( -12.20000000000000284, -35.14999999999999147, -40.00000000000000000 ) ) ;
#32764=STYLED_ITEM ( 'NONE', ( #62767 ), #74598 ) ;
#32766=AXIS2_PLACEMENT_3D ( 'NONE', #25605, #91591, #115434 ) ;
#32774=( GEOMETRIC_REPRESENTATION_CONTEXT ( 3 ) GLOBAL_UNCERTAINTY_ASSIGNED_CONTEXT ( ( #47664 ) ) GLOBAL_UNIT_ASSIGNED_CONTEXT ( ( #127656, #41331, #74722 ) ) REPRESENTATION_CONTEXT ( 'NONE', 'WORKASPACE' ) );
#32865=DIRECTION ( 'NONE',  ( 0.000000000000000000, 0.000000000000000000, 1.000000000000000000 ) ) ;
#32904=LINE ( 'NONE', #55352, #98688 ) ;
#32905=LINE ( 'NONE', #142362, #49420 ) ;
#32908=EDGE_LOOP ( 'NONE', ( #136686, #75537, #74017, #24261 ) ) ;
#32950=AXIS2_PLACEMENT_3D ( 'NONE', #42658, #28902, #106409 ) ;
#32986=ORIENTED_EDGE ( 'NONE', *, *, #50570, .F. ) ;
#33010=CARTESIAN_POINT ( 'NONE',  ( -12.20000000000000107, -34.64999999999999147, 17.49210858042622263 ) ) ;
#33049=( NAMED_UNIT ( * ) SI_UNIT ( $, .STERADIAN. ) SOLID_ANGLE_UNIT ( ) );
#33050=UNCERTAINTY_MEASURE_WITH_UNIT (LENGTH_MEASURE( 1.000000000000000082E-05 ), #33490, 'distance_accuracy_value', 'NONE');
#33069=CARTESIAN_POINT ( 'NONE',  ( 19.93618820137057668, -6.269999999999995133, -40.00000000000000000 ) ) ;
#33094=DIRECTION ( 'NONE',  ( -0.000000000000000000, -1.016133275908817741E-16, 1.000000000000000000 ) ) ;
#33131=CYLINDRICAL_SURFACE ( 'NONE', #125841, 0.5000000000000004441 ) ;
#33137=VECTOR ( 'NONE', #35131, 1000.000000000000000 ) ;
#33183=LINE ( 'NONE', #22233, #140882 ) ;
#33190=UNCERTAINTY_MEASURE_WITH_UNIT (LENGTH_MEASURE( 1.000000000000000082E-05 ), #75858, 'distance_accuracy_value', 'NONE');
#33221=DIRECTION ( 'NONE',  ( 0.000000000000000000, 0.000000000000000000, -1.000000000000000000 ) ) ;
#33258=CARTESIAN_POINT ( 'NONE',  ( -7.140000000000001457, -35.14999999999999147, -40.00000000000000000 ) ) ;
#33306=EDGE_CURVE ( 'NONE', #42501, #134318, #55485, .T. ) ;
#33313=CARTESIAN_POINT ( 'NONE',  ( 19.72391290958995569, -1.589875490879015141, -32.21414776232133192 ) ) ;
#33327=DIRECTION ( 'NONE',  ( 0.3240768213499733985, -0.9146165434626267743, -0.2417659866237898969 ) ) ;
#33329=CARTESIAN_POINT ( 'NONE',  ( 7.139999999999991687, -35.76999999999998892, -7.899272885403729738 ) ) ;
#33343=AXIS2_PLACEMENT_3D ( 'NONE', #127852, #137293, #27798 ) ;
#33368=CARTESIAN_POINT ( 'NONE',  ( 16.55917894070448426, 0.6741881004290185553, -33.57943960405233241 ) ) ;
#33390=( LENGTH_UNIT ( ) NAMED_UNIT ( * ) SI_UNIT ( .MILLI., .METRE. ) );
#33490=( LENGTH_UNIT ( ) NAMED_UNIT ( * ) SI_UNIT ( .MILLI., .METRE. ) );
#33525=DIRECTION ( 'NONE',  ( 0.000000000000000000, 0.000000000000000000, 1.000000000000000000 ) ) ;
#33583=CARTESIAN_POINT ( 'NONE',  ( -6.640000000000001457, 0.000000000000000000, -39.50000000000000000 ) ) ;
#33591=CARTESIAN_POINT ( 'NONE',  ( -12.20000000000000284, -22.33999999999998565, 0.000000000000000000 ) ) ;
#33626=CARTESIAN_POINT ( 'NONE',  ( -12.20000000000000817, -1.670812611072399357E-15, -39.50000000000000000 ) ) ;
#33679=CARTESIAN_POINT ( 'NONE',  ( 14.19664412335589887, 5.303595669547504166, -31.75409969297703938 ) ) ;
#33705=ORIENTED_EDGE ( 'NONE', *, *, #67696, .F. ) ;
#33712=VECTOR ( 'NONE', #97375, 1000.000000000000000 ) ;
#33717=CARTESIAN_POINT ( 'NONE',  ( -34.92499999999999005, -7.730000000000016414, 3.180000000000000160 ) ) ;
#33775=CARTESIAN_POINT ( 'NONE',  ( -12.19999999999999574, -60.26999999999998892, 25.00000000000000000 ) ) ;
#33787=CARTESIAN_POINT ( 'NONE',  ( -7.140000000000001457, -35.56014942880461405, -8.278119684037248405 ) ) ;
#33794=CARTESIAN_POINT ( 'NONE',  ( -16.95726112187796986, -0.7092031756307797252, -35.09041480028862736 ) ) ;
#33820=DIRECTION ( 'NONE',  ( 1.000000000000000000, -2.496005001405478586E-15, 6.809571051365719919E-16 ) ) ;
#33860=EDGE_LOOP ( 'NONE', ( #25036, #138873, #29543, #27878 ) ) ;
#33890=CARTESIAN_POINT ( 'NONE',  ( 17.33001774602888645, -2.066807786662312463, -32.74895997315899621 ) ) ;
#33898=ORIENTED_EDGE ( 'NONE', *, *, #43480, .F. ) ;
#33899=DIRECTION ( 'NONE',  ( -1.000000000000000000, 2.496005001405478586E-15, -0.000000000000000000 ) ) ;
#33903=EDGE_CURVE ( 'NONE', #89049, #50410, #70970, .T. ) ;
#33919=ORIENTED_EDGE ( 'NONE', *, *, #39825, .T. ) ;
#33974=CARTESIAN_POINT ( 'NONE',  ( 12.19999999999999574, -59.76999999999998892, -39.50000000000000000 ) ) ;
#33977=CARTESIAN_POINT ( 'NONE',  ( 12.19999999999999574, -21.76999999999999247, 0.000000000000000000 ) ) ;
#34003=EDGE_CURVE ( 'NONE', #16702, #81122, #58464, .T. ) ;
#34030=ORIENTED_EDGE ( 'NONE', *, *, #95843, .F. ) ;
#34038=CARTESIAN_POINT ( 'NONE',  ( 19.04500000000000881, 3.130000000000007887, -22.35000000000000142 ) ) ;
#34121=ORIENTED_EDGE ( 'NONE', *, *, #104680, .F. ) ;
#34152=DIRECTION ( 'NONE',  ( -0.000000000000000000, -0.000000000000000000, 1.000000000000000000 ) ) ;
#34154=ORIENTED_EDGE ( 'NONE', *, *, #32298, .F. ) ;
#34178=VERTEX_POINT ( 'NONE', #34946 ) ;
#34222=ADVANCED_FACE ( 'NONE', ( #47290 ), #50802, .T. ) ;
#34232=CARTESIAN_POINT ( 'NONE',  ( 19.28515664589288647, 1.196650378695337302, -30.59010235425025215 ) ) ;
#34267=CARTESIAN_POINT ( 'NONE',  ( 31.92500000000001492, -3.269999999999992468, -36.39086428169088094 ) ) ;
#34276=ORIENTED_EDGE ( 'NONE', *, *, #86207, .T. ) ;
#34349=FACE_OUTER_BOUND ( 'NONE', #92097, .T. ) ;
#34372=CARTESIAN_POINT ( 'NONE',  ( 15.15510207594467218, 3.811689137368155844, -32.44374734479579558 ) ) ;
#34379=VERTEX_POINT ( 'NONE', #31199 ) ;
#34433=SURFACE_SIDE_STYLE ('',( #13365 ) ) ;
#34434=UNCERTAINTY_MEASURE_WITH_UNIT (LENGTH_MEASURE( 1.000000000000000082E-05 ), #86886, 'distance_accuracy_value', 'NONE');
#34488=CARTESIAN_POINT ( 'NONE',  ( -17.01299344913721612, -0.9444867979315253459, -36.05398659021086871 ) ) ;
#34538=( BOUNDED_CURVE ( )  B_SPLINE_CURVE ( 3, ( #28751, #137505, #29431, #95409 ),
 .UNSPECIFIED., .F., .T. ) 
 B_SPLINE_CURVE_WITH_KNOTS ( ( 4, 4 ),
 ( 4.712388980384696779, 6.283185307179586232 ),
 .UNSPECIFIED. ) 
 CURVE ( )  GEOMETRIC_REPRESENTATION_ITEM ( )  RATIONAL_B_SPLINE_CURVE ( ( 1.000000000000000000, 0.8047378541243667138, 0.8047378541243667138, 1.000000000000000000 ) ) 
 REPRESENTATION_ITEM ( '' )  );
#34567=CARTESIAN_POINT ( 'NONE',  ( 12.69999999999999574, -22.26999999999999247, -39.50000000000000000 ) ) ;
#34595=CARTESIAN_POINT ( 'NONE',  ( 19.92001344501310456, -3.130733134304450438, -35.06310854429385415 ) ) ;
#34641=( LENGTH_UNIT ( ) NAMED_UNIT ( * ) SI_UNIT ( .MILLI., .METRE. ) );
#34662=FACE_OUTER_BOUND ( 'NONE', #120867, .T. ) ;
#34705=CARTESIAN_POINT ( 'NONE',  ( 34.92500000000001847, -6.269999999999991580, -36.39086428169088094 ) ) ;
#34726=CIRCLE ( 'NONE', #134280, 0.5000000000000004441 ) ;
#34787=UNCERTAINTY_MEASURE_WITH_UNIT (LENGTH_MEASURE( 1.000000000000000082E-05 ), #94824, 'distance_accuracy_value', 'NONE');
#34841=FILL_AREA_STYLE ('',( #68905 ) ) ;
#34842=COLOUR_RGB ( '', 0.09019608, 0.27058824, 0.51372549) ;
#34857=ORIENTED_EDGE ( 'NONE', *, *, #48379, .T. ) ;
#34869=AXIS2_PLACEMENT_3D ( 'NONE', #52092, #75294, #118767 ) ;
#34946=CARTESIAN_POINT ( 'NONE',  ( -12.20000000000000284, -25.33999999999998920, 13.17925390838734323 ) ) ;
#34981=ORIENTED_EDGE ( 'NONE', *, *, #59442, .T. ) ;
#34982=ORIENTED_EDGE ( 'NONE', *, *, #123443, .F. ) ;
#35031=( NAMED_UNIT ( * ) PLANE_ANGLE_UNIT ( ) SI_UNIT ( $, .RADIAN. ) );
#35053=AXIS2_PLACEMENT_3D ( 'NONE', #106557, #71132, #94976 ) ;
#35088=SURFACE_SIDE_STYLE ('',( #12579 ) ) ;
#35090=AXIS2_PLACEMENT_3D ( 'NONE', #101207, #126355, #27041 ) ;
#35129=AXIS2_PLACEMENT_3D ( 'NONE', #52909, #76127, #131218 ) ;
#35131=DIRECTION ( 'NONE',  ( -0.000000000000000000, -0.000000000000000000, -1.000000000000000000 ) ) ;
#35215=EDGE_CURVE ( 'NONE', #20082, #63324, #50602, .T. ) ;
#35229=CARTESIAN_POINT ( 'NONE',  ( -19.71993606672559096, -1.561048305595850838, -32.18456460708710409 ) ) ;
#35240=EDGE_CURVE ( 'NONE', #21068, #48074, #3795, .T. ) ;
#35255=MECHANICAL_DESIGN_GEOMETRIC_PRESENTATION_REPRESENTATION('',(#32764),#72325);
#35272=( GEOMETRIC_REPRESENTATION_CONTEXT ( 3 ) GLOBAL_UNCERTAINTY_ASSIGNED_CONTEXT ( ( #11181 ) ) GLOBAL_UNIT_ASSIGNED_CONTEXT ( ( #23420, #71063, #44514 ) ) REPRESENTATION_CONTEXT ( 'NONE', 'WORKASPACE' ) );
#35298=ADVANCED_FACE ( 'NONE', ( #117248 ), #122086, .T. ) ;
#35317=CARTESIAN_POINT ( 'NONE',  ( -33.18123773989405834, 22.27000000000001378, -14.20145869268583638 ) ) ;
#35327=EDGE_CURVE ( 'NONE', #89438, #117423, #29539, .T. ) ;
#35336=FILL_AREA_STYLE ('',( #135357 ) ) ;
#35368=STYLED_ITEM ( 'NONE', ( #118843 ), #16183 ) ;
#35413=COLOUR_RGB ( '', 0.31764706, 0.68627451, 0.89019608) ;
#35421=LINE ( 'NONE', #112238, #39911 ) ;
#35456=ORIENTED_EDGE ( 'NONE', *, *, #29243, .T. ) ;
#35470=( LENGTH_UNIT ( ) NAMED_UNIT ( * ) SI_UNIT ( .MILLI., .METRE. ) );
#35480=DIRECTION ( 'NONE',  ( -0.000000000000000000, -0.000000000000000000, -1.000000000000000000 ) ) ;
#35487=ORIENTED_EDGE ( 'NONE', *, *, #44194, .T. ) ;
#35512=FACE_OUTER_BOUND ( 'NONE', #87613, .T. ) ;
#35522=CYLINDRICAL_SURFACE ( 'NONE', #116412, 0.5000000000000000000 ) ;
#35549=EDGE_LOOP ( 'NONE', ( #744, #68169, #1271, #98429 ) ) ;
#35566=CIRCLE ( 'NONE', #40213, 9.524999999999991473 ) ;
#35580=( LENGTH_UNIT ( ) NAMED_UNIT ( * ) SI_UNIT ( .MILLI., .METRE. ) );
#35628=VECTOR ( 'NONE', #55063, 1000.000000000000000 ) ;
#35630=DIRECTION ( 'NONE',  ( -0.000000000000000000, -0.000000000000000000, 1.000000000000000000 ) ) ;
#35637=( NAMED_UNIT ( * ) SI_UNIT ( $, .STERADIAN. ) SOLID_ANGLE_UNIT ( ) );
#35649=EDGE_CURVE ( 'NONE', #66948, #59938, #122917, .T. ) ;
#35703=( NAMED_UNIT ( * ) PLANE_ANGLE_UNIT ( ) SI_UNIT ( $, .RADIAN. ) );
#35725=SPHERICAL_SURFACE ( 'NONE', #69342, 0.5000000000000000000 ) ;
#35779=ORIENTED_EDGE ( 'NONE', *, *, #34003, .F. ) ;
#35796=ORIENTED_EDGE ( 'NONE', *, *, #111668, .T. ) ;
#35878=AXIS2_PLACEMENT_3D ( 'NONE', #104402, #82677, #29691 ) ;
#35895=UNCERTAINTY_MEASURE_WITH_UNIT (LENGTH_MEASURE( 1.000000000000000082E-05 ), #35580, 'distance_accuracy_value', 'NONE');
#35901=CIRCLE ( 'NONE', #47509, 9.524999999999998579 ) ;
#35942=CARTESIAN_POINT ( 'NONE',  ( -16.98224699891571277, -0.6362351928176004368, -31.34040500397710005 ) ) ;
#35946=FACE_OUTER_BOUND ( 'NONE', #93582, .T. ) ;
#36042=CARTESIAN_POINT ( 'NONE',  ( 16.98219951865394606, -0.6360915077794555561, -31.34035742411751713 ) ) ;
#36054=LINE ( 'NONE', #14272, #40649 ) ;
#36089=DIRECTION ( 'NONE',  ( -0.000000000000000000, -1.000000000000000000, -0.000000000000000000 ) ) ;
#36099=DIRECTION ( 'NONE',  ( 0.000000000000000000, 0.000000000000000000, -1.000000000000000000 ) ) ;
#36173=EDGE_CURVE ( 'NONE', #131559, #91102, #119458, .T. ) ;
#36204=CIRCLE ( 'NONE', #68928, 6.000000000000000000 ) ;
#36241=DIRECTION ( 'NONE',  ( 1.000000000000000000, 0.000000000000000000, 0.000000000000000000 ) ) ;
#36281=MECHANICAL_DESIGN_GEOMETRIC_PRESENTATION_REPRESENTATION('',(#10780),#103410);
#36329=ORIENTED_EDGE ( 'NONE', *, *, #127291, .T. ) ;
#36342=VERTEX_POINT ( 'NONE', #130019 ) ;
#36436=SURFACE_SIDE_STYLE ('',( #91537 ) ) ;
#36467=PRESENTATION_STYLE_ASSIGNMENT (( #15381 ) ) ;
#36488=CYLINDRICAL_SURFACE ( 'NONE', #64414, 9.524999999999995026 ) ;
#36498=ORIENTED_EDGE ( 'NONE', *, *, #18426, .T. ) ;
#36579=AXIS2_PLACEMENT_3D ( 'NONE', #33583, #20503, #32865 ) ;
#36580=SPHERICAL_SURFACE ( 'NONE', #83778, 0.5000000000000000000 ) ;
#36589=CARTESIAN_POINT ( 'NONE',  ( -12.69999999999999929, -59.76999999999998892, 24.34531699603381938 ) ) ;
#36595=DIRECTION ( 'NONE',  ( 0.000000000000000000, 0.000000000000000000, 1.000000000000000000 ) ) ;
#36598=EDGE_CURVE ( 'NONE', #70234, #113156, #87939, .T. ) ;
#36613=FACE_OUTER_BOUND ( 'NONE', #95961, .T. ) ;
#36616=( NAMED_UNIT ( * ) PLANE_ANGLE_UNIT ( ) SI_UNIT ( $, .RADIAN. ) );
#36663=FILL_AREA_STYLE_COLOUR ( '', #74984 ) ;
#36702=LINE ( 'NONE', #80249, #71838 ) ;
#36720=CARTESIAN_POINT ( 'NONE',  ( 17.39690951308662648, -2.395832017967521654, -33.23817995126653813 ) ) ;
#36778=EDGE_CURVE ( 'NONE', #64204, #135652, #110490, .T. ) ;
#36808=VERTEX_POINT ( 'NONE', #111966 ) ;
#36812=AXIS2_PLACEMENT_3D ( 'NONE', #26913, #137837, #14615 ) ;
#36886=FACE_OUTER_BOUND ( 'NONE', #108547, .T. ) ;
#36918=EDGE_CURVE ( 'NONE', #77610, #40891, #3170, .T. ) ;
#36962=LINE ( 'NONE', #23406, #98137 ) ;
#36993=ORIENTED_EDGE ( 'NONE', *, *, #116962, .T. ) ;
#37015=DIRECTION ( 'NONE',  ( -1.000000000000000000, 0.000000000000000000, 0.000000000000000000 ) ) ;
#37031=VECTOR ( 'NONE', #133415, 1000.000000000000114 ) ;
#37075=DIRECTION ( 'NONE',  ( 0.000000000000000000, 0.000000000000000000, 1.000000000000000000 ) ) ;
#37082=DIRECTION ( 'NONE',  ( 0.000000000000000000, 0.000000000000000000, 1.000000000000000000 ) ) ;
#37085=DIRECTION ( 'NONE',  ( 0.000000000000000000, -0.000000000000000000, -1.000000000000000000 ) ) ;
#37086=CARTESIAN_POINT ( 'NONE',  ( -34.92499999999999005, 1.196650378695320427, -30.59010235425025215 ) ) ;
#37093=TOROIDAL_SURFACE ( 'NONE', #127328, 2.500000000000000000, 0.5000000000000000000 ) ;
#37111=CYLINDRICAL_SURFACE ( 'NONE', #14936, 0.5000000000000004441 ) ;
#37142=DIRECTION ( 'NONE',  ( -0.000000000000000000, 0.9647414015272155474, -0.2631995976047525887 ) ) ;
#37146=( LENGTH_UNIT ( ) NAMED_UNIT ( * ) SI_UNIT ( .MILLI., .METRE. ) );
#37189=ORIENTED_EDGE ( 'NONE', *, *, #65628, .F. ) ;
#37193=DIRECTION ( 'NONE',  ( 0.000000000000000000, 1.000000000000000000, 0.000000000000000000 ) ) ;
#37378=DIRECTION ( 'NONE',  ( 3.115803279706882722E-16, -1.000000000000000000, -1.016133275908817741E-16 ) ) ;
#37382=CARTESIAN_POINT ( 'NONE',  ( -12.20000000000000284, -25.33999999999998209, 15.47043909406156104 ) ) ;
#37395=CARTESIAN_POINT ( 'NONE',  ( -16.67979525387081807, 0.3337821591035541879, -30.81818940114110816 ) ) ;
#37418=( GEOMETRIC_REPRESENTATION_CONTEXT ( 3 ) GLOBAL_UNCERTAINTY_ASSIGNED_CONTEXT ( ( #15625 ) ) GLOBAL_UNIT_ASSIGNED_CONTEXT ( ( #51391, #140512, #94853 ) ) REPRESENTATION_CONTEXT ( 'NONE', 'WORKASPACE' ) );
#37441=ORIENTED_EDGE ( 'NONE', *, *, #98917, .T. ) ;
#37459=ORIENTED_EDGE ( 'NONE', *, *, #102660, .F. ) ;
#37480=DIRECTION ( 'NONE',  ( 0.000000000000000000, 0.000000000000000000, -1.000000000000000000 ) ) ;
#37515=FILL_AREA_STYLE ('',( #49109 ) ) ;
#37553=SURFACE_STYLE_FILL_AREA ( #83188 ) ;
#37658=CYLINDRICAL_SURFACE ( 'NONE', #29794, 0.5000000000000004441 ) ;
#37672=EDGE_CURVE ( 'NONE', #18833, #36342, #129305, .T. ) ;
#37761=DIRECTION ( 'NONE',  ( 0.000000000000000000, -1.000000000000000000, 0.000000000000000000 ) ) ;
#37762=CARTESIAN_POINT ( 'NONE',  ( 12.69999999999999574, 0.000000000000000000, -40.00000000000000000 ) ) ;
#37837=ORIENTED_EDGE ( 'NONE', *, *, #95890, .F. ) ;
#37869=ORIENTED_EDGE ( 'NONE', *, *, #19743, .T. ) ;
#37886=DIRECTION ( 'NONE',  ( -0.000000000000000000, -0.000000000000000000, 1.000000000000000000 ) ) ;
#37965=CARTESIAN_POINT ( 'NONE',  ( 34.42500000000002558, -21.76999999999999247, -37.00000000000000000 ) ) ;
#37966=DIRECTION ( 'NONE',  ( 1.000000000000000000, 0.000000000000000000, -0.000000000000000000 ) ) ;
#38036=ORIENTED_EDGE ( 'NONE', *, *, #79772, .T. ) ;
#38058=VERTEX_POINT ( 'NONE', #101806 ) ;
#38078=EDGE_CURVE ( 'NONE', #97698, #121504, #48871, .T. ) ;
#38120=( NAMED_UNIT ( * ) PLANE_ANGLE_UNIT ( ) SI_UNIT ( $, .RADIAN. ) );
#38126=DIRECTION ( 'NONE',  ( 1.000000000000000000, 0.000000000000000000, -0.000000000000000000 ) ) ;
#38149=AXIS2_PLACEMENT_3D ( 'NONE', #129191, #18268, #62546 ) ;
#38171=VECTOR ( 'NONE', #118551, 1000.000000000000000 ) ;
#38176=CARTESIAN_POINT ( 'NONE',  ( 17.01299344985120499, -0.9444868010259039881, -36.22218118524219932 ) ) ;
#38181=VERTEX_POINT ( 'NONE', #60479 ) ;
#38196=CARTESIAN_POINT ( 'NONE',  ( 7.940000000000001279, -33.26999999999999602, -8.101350000000008933 ) ) ;
#38287=DIRECTION ( 'NONE',  ( 0.000000000000000000, 0.000000000000000000, 1.000000000000000000 ) ) ;
#38322=DIRECTION ( 'NONE',  ( 1.369518533665900312E-16, -1.000000000000000000, 0.000000000000000000 ) ) ;
#38349=ADVANCED_FACE ( 'NONE', ( #42992 ), #98761, .F. ) ;
#38394=CIRCLE ( 'NONE', #84648, 3.000000000000002665 ) ;
#38411=LINE ( 'NONE', #27507, #58463 ) ;
#38420=ORIENTED_EDGE ( 'NONE', *, *, #119890, .F. ) ;
#38426=EDGE_CURVE ( 'NONE', #117264, #120537, #122391, .T. ) ;
#38456=FILL_AREA_STYLE ('',( #24711 ) ) ;
#38470=EDGE_LOOP ( 'NONE', ( #9225, #28071 ) ) ;
#38480=DIRECTION ( 'NONE',  ( -1.000000000000000000, 0.000000000000000000, 0.000000000000000000 ) ) ;
#38487=VECTOR ( 'NONE', #42855, 1000.000000000000000 ) ;
#38519=DIRECTION ( 'NONE',  ( -1.000000000000000000, -3.115803279706882722E-16, 0.000000000000000000 ) ) ;
#38567=DIRECTION ( 'NONE',  ( 0.000000000000000000, 0.000000000000000000, -1.000000000000000000 ) ) ;
#38575=DIRECTION ( 'NONE',  ( 1.000000000000000000, 0.000000000000000000, 0.000000000000000000 ) ) ;
#38608=( NAMED_UNIT ( * ) PLANE_ANGLE_UNIT ( ) SI_UNIT ( $, .RADIAN. ) );
#38648=DIRECTION ( 'NONE',  ( 0.000000000000000000, 0.000000000000000000, -1.000000000000000000 ) ) ;
#38652=AXIS2_PLACEMENT_3D ( 'NONE', #66804, #24715, #68968 ) ;
#38692=DIRECTION ( 'NONE',  ( 0.000000000000000000, 0.000000000000000000, 1.000000000000000000 ) ) ;
#38745=CARTESIAN_POINT ( 'NONE',  ( 7.139999999999985469, -39.93000000000000682, -12.10072711459627293 ) ) ;
#38782=FILL_AREA_STYLE ('',( #138094 ) ) ;
#38825=CARTESIAN_POINT ( 'NONE',  ( -16.96380654081093553, 5.480407308985125070, -29.16618357164760766 ) ) ;
#38850=ORIENTED_EDGE ( 'NONE', *, *, #124322, .T. ) ;
#38855=TOROIDAL_SURFACE ( 'NONE', #57400, 3.500000000000000000, 0.5000000000000000000 ) ;
#38856=CARTESIAN_POINT ( 'NONE',  ( -34.75757056450616744, 22.27000000000000668, -10.47732366696226869 ) ) ;
#38863=UNCERTAINTY_MEASURE_WITH_UNIT (LENGTH_MEASURE( 1.000000000000000082E-05 ), #142435, 'distance_accuracy_value', 'NONE');
#38919=VERTEX_POINT ( 'NONE', #50652 ) ;
#38958=COLOUR_RGB ( '', 0.08235294, 0.09019608, 0.10196078) ;
#39004=CARTESIAN_POINT ( 'NONE',  ( -7.940000000000007496, -39.92999999999999261, -10.00000000000000178 ) ) ;
#39010=AXIS2_PLACEMENT_3D ( 'NONE', #109089, #110502, #43860 ) ;
#39183=MECHANICAL_DESIGN_GEOMETRIC_PRESENTATION_REPRESENTATION('',(#67022),#78611);
#39185=CIRCLE ( 'NONE', #55437, 0.5000000000000004441 ) ;
#39203=ORIENTED_EDGE ( 'NONE', *, *, #76752, .F. ) ;
#39214=CARTESIAN_POINT ( 'NONE',  ( 6.640000000000043201, -9.638965590364918103E-15, -39.50000000000000000 ) ) ;
#39230=VERTEX_POINT ( 'NONE', #13368 ) ;
#39231=CARTESIAN_POINT ( 'NONE',  ( -2.132336019816571060, 13.66774714948344283, -24.42935889323532805 ) ) ;
#39254=FILL_AREA_STYLE_COLOUR ( '', #87127 ) ;
#39362=FACE_OUTER_BOUND ( 'NONE', #76789, .T. ) ;
#39405=MECHANICAL_DESIGN_GEOMETRIC_PRESENTATION_REPRESENTATION('',(#90396),#76455);
#39442=ADVANCED_FACE ( 'NONE', ( #21245 ), #132172, .T. ) ;
#39476=CARTESIAN_POINT ( 'NONE',  ( 34.92500000000001137, 22.27000000000000668, -40.00000000000000000 ) ) ;
#39478=CARTESIAN_POINT ( 'NONE',  ( -17.01299345042646749, -0.9444868035190714384, -36.07450300634584295 ) ) ;
#39497=SURFACE_STYLE_USAGE ( .BOTH. , #6801 ) ;
#39545=ORIENTED_EDGE ( 'NONE', *, *, #112721, .F. ) ;
#39555=CARTESIAN_POINT ( 'NONE',  ( -17.51947408101518633, 4.682391862010510053, -29.48234182121950653 ) ) ;
#39578=CARTESIAN_POINT ( 'NONE',  ( -7.140000000000001457, -39.92999999999999261, 18.93259187797432475 ) ) ;
#39693=ORIENTED_EDGE ( 'NONE', *, *, #17255, .T. ) ;
#39825=EDGE_CURVE ( 'NONE', #113508, #48675, #109514, .T. ) ;
#39852=CIRCLE ( 'NONE', #55997, 2.552699999999994418 ) ;
#39911=VECTOR ( 'NONE', #99172, 1000.000000000000000 ) ;
#39972=CARTESIAN_POINT ( 'NONE',  ( -5.731388644227705775, 12.99752701236087660, -24.93595787201127578 ) ) ;
#39979=CARTESIAN_POINT ( 'NONE',  ( 12.19999999999999574, 12.19802518668052649, 4.711086268963014412 ) ) ;
#40008=( LENGTH_UNIT ( ) NAMED_UNIT ( * ) SI_UNIT ( .MILLI., .METRE. ) );
#40040=FILL_AREA_STYLE ('',( #95080 ) ) ;
#40061=ORIENTED_EDGE ( 'NONE', *, *, #77316, .T. ) ;
#40097=ORIENTED_EDGE ( 'NONE', *, *, #46901, .F. ) ;
#40134=VECTOR ( 'NONE', #40732, 1000.000000000000000 ) ;
#40149=B_SPLINE_CURVE_WITH_KNOTS ( 'NONE', 3,
 ( #34232, #853, #45144, #24068, #11007, #57428, #68325, #13157, #88626, #55275, #44422, #2267, #89320, #122649, #101613, #99452, #47301, #24769, #78456, #113193, #91472, #23325, #25468, #138542, #26912, #71157, #39231, #116773, #124801, #82736, #39972, #69746, #49421, #113923, #5841, #14614, #16748, #60284, #115301, #27615, #92879, #61028, #127671, #4374, #47985, #136383 ),
 .UNSPECIFIED., .F., .F.,
 ( 4, 2, 2, 2, 2, 2, 2, 2, 2, 2, 2, 2, 2, 2, 2, 2, 2, 2, 2, 2, 2, 2, 4 ),
 ( 1.301042606982605321E-18, 0.003160655639991156486, 0.004740983459986731693, 0.006321311279982309503, 0.009481966919973470326, 0.01106229473996905160, 0.01264262255996463115, 0.01580327819995578503, 0.01738360601995135937, 0.01896393383994693718, 0.02212458947993808239, 0.02370491729993365326, 0.02528524511992922413, 0.02844590075992036934, 0.03002622857991594021, 0.03160655639991151455, 0.03476721203990266323, 0.03792786767989381191, 0.04108852331988496059, 0.04266885113988053840, 0.04424917895987611621, 0.04740983459986727183, 0.05057049023985842745 ),
 .UNSPECIFIED. ) ;
#40191=CARTESIAN_POINT ( 'NONE',  ( 31.92500000000001492, 1.196650378695341299, -30.59010235425025215 ) ) ;
#40213=AXIS2_PLACEMENT_3D ( 'NONE', #11983, #47536, #111294 ) ;
#40247=ORIENTED_EDGE ( 'NONE', *, *, #81922, .F. ) ;
#40258=EDGE_CURVE ( 'NONE', #12164, #126832, #21626, .T. ) ;
#40259=CARTESIAN_POINT ( 'NONE',  ( 12.19999999999999574, -40.43000000000000682, -39.50000000000000000 ) ) ;
#40280=CARTESIAN_POINT ( 'NONE',  ( -16.45742106731621490, 0.9613713492673534589, -33.49048331797056477 ) ) ;
#40332=DIRECTION ( 'NONE',  ( -1.369518533665900312E-16, 1.000000000000000000, -0.000000000000000000 ) ) ;
#40406=VERTEX_POINT ( 'NONE', #56446 ) ;
#40420=DIRECTION ( 'NONE',  ( 1.000000000000000000, 0.000000000000000000, 0.000000000000000000 ) ) ;
#40422=ORIENTED_EDGE ( 'NONE', *, *, #177, .T. ) ;
#40427=B_SPLINE_CURVE_WITH_KNOTS ( 'NONE', 3,
 ( #101247, #99823, #122266, #1884, #134620, #35317, #79557, #68649, #28712, #62060, #4731, #71490, #38856, #117109, #103367, #59220 ),
 .UNSPECIFIED., .F., .F.,
 ( 4, 2, 2, 2, 2, 2, 2, 4 ),
 ( 0.000000000000000000, 0.0005146009271697703615, 0.001029201854339540723, 0.002058403708679101395, 0.003087605563018661851, 0.004116807417358222740, 0.006175211126037349722, 0.008233614834716476705 ),
 .UNSPECIFIED. ) ;
#40430=EDGE_CURVE ( 'NONE', #128814, #115328, #124501, .T. ) ;
#40469=AXIS2_PLACEMENT_3D ( 'NONE', #33974, #134735, #45585 ) ;
#40480=CARTESIAN_POINT ( 'NONE',  ( -7.940000000000001279, -33.26999999999999602, -10.00000000000000178 ) ) ;
#40498=( NAMED_UNIT ( * ) SI_UNIT ( $, .STERADIAN. ) SOLID_ANGLE_UNIT ( ) );
#40528=DIRECTION ( 'NONE',  ( -1.000000000000000000, 0.000000000000000000, 3.596245529072721644E-15 ) ) ;
#40550=AXIS2_PLACEMENT_3D ( 'NONE', #55836, #25306, #22436 ) ;
#40552=AXIS2_PLACEMENT_3D ( 'NONE', #27679, #17518, #38575 ) ;
#40556=DIRECTION ( 'NONE',  ( 0.000000000000000000, 0.000000000000000000, -1.000000000000000000 ) ) ;
#40600=EDGE_CURVE ( 'NONE', #56871, #25054, #132896, .T. ) ;
#40615=ADVANCED_FACE ( 'NONE', ( #121574 ), #121260, .T. ) ;
#40649=VECTOR ( 'NONE', #104108, 1000.000000000000000 ) ;
#40678=FILL_AREA_STYLE ('',( #39254 ) ) ;
#40732=DIRECTION ( 'NONE',  ( 0.000000000000000000, -1.000000000000000000, 0.000000000000000000 ) ) ;
#40785=( NAMED_UNIT ( * ) PLANE_ANGLE_UNIT ( ) SI_UNIT ( $, .RADIAN. ) );
#40855=EDGE_CURVE ( 'NONE', #131359, #133539, #115785, .T. ) ;
#40864=CIRCLE ( 'NONE', #45555, 2.999999999999999112 ) ;
#40891=VERTEX_POINT ( 'NONE', #85210 ) ;
#40901=ORIENTED_EDGE ( 'NONE', *, *, #79213, .F. ) ;
#40965=CARTESIAN_POINT ( 'NONE',  ( -3.933891695358868734, 12.14980826004766712, -25.57915494108756249 ) ) ;
#40966=VERTEX_POINT ( 'NONE', #78640 ) ;
#40976=CARTESIAN_POINT ( 'NONE',  ( 12.69999999999999574, -22.26999999999999247, -39.50000000000000000 ) ) ;
#41075=SURFACE_SIDE_STYLE ('',( #140385 ) ) ;
#41080=DIRECTION ( 'NONE',  ( 0.000000000000000000, 0.000000000000000000, 1.000000000000000000 ) ) ;
#41144=CARTESIAN_POINT ( 'NONE',  ( -12.20000000000000284, -39.92999999999999261, -39.50000000000000000 ) ) ;
#41161=DIRECTION ( 'NONE',  ( -0.000000000000000000, -1.000000000000000000, -0.000000000000000000 ) ) ;
#41183=CARTESIAN_POINT ( 'NONE',  ( -12.49289321881345494, -22.06289321881344634, -40.00000000000000000 ) ) ;
#41199=CYLINDRICAL_SURFACE ( 'NONE', #65174, 3.000000000000000000 ) ;
#41227=COLOUR_RGB ( '', 0.40784314, 0.44705882, 0.49803922) ;
#41271=AXIS2_PLACEMENT_3D ( 'NONE', #68110, #112291, #132642 ) ;
#41283=ORIENTED_EDGE ( 'NONE', *, *, #102660, .T. ) ;
#41317=FILL_AREA_STYLE_COLOUR ( '', #131604 ) ;
#41331=( NAMED_UNIT ( * ) PLANE_ANGLE_UNIT ( ) SI_UNIT ( $, .RADIAN. ) );
#41340=CARTESIAN_POINT ( 'NONE',  ( 12.69999999999999574, -22.33999999999998565, 0.000000000000000000 ) ) ;
#41365=SURFACE_SIDE_STYLE ('',( #83467 ) ) ;
#41390=CARTESIAN_POINT ( 'NONE',  ( 0.9194859777227279984, 12.57226318162868672, -26.75049658419982634 ) ) ;
#41395=( GEOMETRIC_REPRESENTATION_CONTEXT ( 3 ) GLOBAL_UNCERTAINTY_ASSIGNED_CONTEXT ( ( #2664 ) ) GLOBAL_UNIT_ASSIGNED_CONTEXT ( ( #86950, #99966, #68791 ) ) REPRESENTATION_CONTEXT ( 'NONE', 'WORKASPACE' ) );
#41467=( NAMED_UNIT ( * ) PLANE_ANGLE_UNIT ( ) SI_UNIT ( $, .RADIAN. ) );
#41473=AXIS2_PLACEMENT_3D ( 'NONE', #28048, #73017, #116478 ) ;
#41489=VECTOR ( 'NONE', #42242, 1000.000000000000000 ) ;
#41490=CARTESIAN_POINT ( 'NONE',  ( -21.60769999999999058, 3.130000000000008331, -2.396719511207313368E-16 ) ) ;
#41508=CARTESIAN_POINT ( 'NONE',  ( -19.93618820135885983, -3.270000000000009788, -35.72555304890778416 ) ) ;
#41542=CARTESIAN_POINT ( 'NONE',  ( 0.000000000000000000, -39.92999999999999261, -40.00000000000000000 ) ) ;
#41554=AXIS2_PLACEMENT_3D ( 'NONE', #142824, #97895, #142133 ) ;
#41604=SURFACE_SIDE_STYLE ('',( #73540 ) ) ;
#41660=VERTEX_POINT ( 'NONE', #133127 ) ;
#41671=CARTESIAN_POINT ( 'NONE',  ( 5.327707837555167636, 13.12214320084893870, -24.84562023559181654 ) ) ;
#41730=ORIENTED_EDGE ( 'NONE', *, *, #65059, .T. ) ;
#41788=ORIENTED_EDGE ( 'NONE', *, *, #74973, .T. ) ;
#41818=VECTOR ( 'NONE', #54443, 1000.000000000000000 ) ;
#41862=ADVANCED_FACE ( 'NONE', ( #109013 ), #85136, .F. ) ;
#41916=AXIS2_PLACEMENT_3D ( 'NONE', #18320, #8846, #66168 ) ;
#41944=SURFACE_STYLE_USAGE ( .BOTH. , #52782 ) ;
#41970=( BOUNDED_SURFACE ( )  B_SPLINE_SURFACE ( 3, 2, ( 
 ( #91813, #113561, #47651 ),
 ( #78824, #136036, #14958 ),
 ( #133214, #36042, #79578 ),
 ( #23711, #112850, #1216 ),
 ( #70125, #123763, #57799 ),
 ( #103388, #59239, #13519 ),
 ( #4035, #33890, #88989 ),
 ( #122284, #36720, #22957 ),
 ( #123035, #101989, #124449 ),
 ( #25119, #67226, #133904 ),
 ( #69378, #89677, #111422 ),
 ( #14259, #12107, #56391 ),
 ( #45500, #100572, #34595 ),
 ( #15639, #6908, #82393 ),
 ( #38176, #126572, #62076 ),
 ( #81697, #16373, #27263 ) ),
 .UNSPECIFIED., .F., .F., .F. ) 
 B_SPLINE_SURFACE_WITH_KNOTS ( ( 4, 2, 2, 2, 2, 2, 2, 4 ),
 ( 3, 3 ),
 ( -4.336808689942017736E-19, 0.0009973376669657767115, 0.001496006500448665393, 0.001994675333931553857, 0.002493344167414442321, 0.002992013000897330785, 0.003490681834380219249, 0.003989350667863107713 ),
 ( 0.000000000000000000, 1.000000000000000000 ),
 .UNSPECIFIED. ) 
 GEOMETRIC_REPRESENTATION_ITEM ( )  RATIONAL_B_SPLINE_SURFACE ( (
 ( 1.000000000000000000, 0.7366656399173067138, 1.000000000000000000),
 ( 1.000000000000000000, 0.7469946078304352532, 1.000000000000000000),
 ( 1.000000000000000000, 0.7550065080344044999, 1.000000000000000000),
 ( 1.000000000000000000, 0.7644701404565185099, 1.000000000000000000),
 ( 1.000000000000000000, 0.7671379903610555662, 1.000000000000000000),
 ( 1.000000000000000000, 0.7716469694716783234, 1.000000000000000000),
 ( 1.000000000000000000, 0.7735028669872892060, 1.000000000000000000),
 ( 1.000000000000000000, 0.7766014048701626038, 1.000000000000000000),
 ( 1.000000000000000000, 0.7778260050860584807, 1.000000000000000000),
 ( 1.000000000000000000, 0.7797609306255449679, 1.000000000000000000),
 ( 1.000000000000000000, 0.7804845266836839546, 1.000000000000000000),
 ( 1.000000000000000000, 0.7815908473005801493, 1.000000000000000000),
 ( 1.000000000000000000, 0.7819678579954093545, 1.000000000000000000),
 ( 1.000000000000000000, 0.7824545089705922107, 1.000000000000000000),
 ( 1.000000000000000000, 0.7825677149574248315, 1.000000000000000000),
 ( 1.000000000000000000, 0.7825691453495833283, 1.000000000000000000) ) ) 
 REPRESENTATION_ITEM ( '' )  SURFACE ( )  );
#41998=( GEOMETRIC_REPRESENTATION_CONTEXT ( 3 ) GLOBAL_UNCERTAINTY_ASSIGNED_CONTEXT ( ( #9983 ) ) GLOBAL_UNIT_ASSIGNED_CONTEXT ( ( #133825, #7905, #122206 ) ) REPRESENTATION_CONTEXT ( 'NONE', 'WORKASPACE' ) );
#42021=SURFACE_SIDE_STYLE ('',( #6463 ) ) ;
#42043=EDGE_CURVE ( 'NONE', #61841, #3531, #65909, .T. ) ;
#42065=CYLINDRICAL_SURFACE ( 'NONE', #23738, 6.000000000000000000 ) ;
#42101=AXIS2_PLACEMENT_3D ( 'NONE', #3757, #113996, #61100 ) ;
#42139=CARTESIAN_POINT ( 'NONE',  ( 14.20335188619867672, 5.294102111022186641, -31.75876904902751718 ) ) ;
#42142=CARTESIAN_POINT ( 'NONE',  ( -7.140000000000001457, -60.26999999999998892, -7.899272885403729738 ) ) ;
#42218=CARTESIAN_POINT ( 'NONE',  ( -19.93618820137057668, -0.2700000000508183118, 500000.0000000000582 ) ) ;
#42225=VECTOR ( 'NONE', #130398, 1000.000000000000000 ) ;
#42238=MECHANICAL_DESIGN_GEOMETRIC_PRESENTATION_REPRESENTATION('',(#74625),#25972);
#42242=DIRECTION ( 'NONE',  ( -1.451651444332056451E-15, -1.000000000000000000, 0.000000000000000000 ) ) ;
#42270=CYLINDRICAL_SURFACE ( 'NONE', #10212, 0.5000000000000004441 ) ;
#42274=SURFACE_STYLE_FILL_AREA ( #44426 ) ;
#42287=VECTOR ( 'NONE', #37966, 1000.000000000000000 ) ;
#42330=ORIENTED_EDGE ( 'NONE', *, *, #10111, .T. ) ;
#42418=CARTESIAN_POINT ( 'NONE',  ( -3.802034438261828964, 13.42402838347469007, -24.61607834315348953 ) ) ;
#42426=ORIENTED_EDGE ( 'NONE', *, *, #5336, .F. ) ;
#42441=PRESENTATION_STYLE_ASSIGNMENT (( #99625 ) ) ;
#42450=ORIENTED_EDGE ( 'NONE', *, *, #87905, .T. ) ;
#42501=VERTEX_POINT ( 'NONE', #125997 ) ;
#42589=CARTESIAN_POINT ( 'NONE',  ( -34.42499999999997584, -21.76999999999999247, -40.00000000000000000 ) ) ;
#42631=DIRECTION ( 'NONE',  ( 0.000000000000000000, 0.000000000000000000, -1.000000000000000000 ) ) ;
#42658=CARTESIAN_POINT ( 'NONE',  ( 7.939999999999994174, -39.93000000000000682, -10.00000000000000178 ) ) ;
#42661=DIRECTION ( 'NONE',  ( 1.412012880465675998E-16, 0.9667936545734397980, 0.2555582702174447052 ) ) ;
#42761=DIRECTION ( 'NONE',  ( 0.000000000000000000, 0.000000000000000000, 1.000000000000000000 ) ) ;
#42855=DIRECTION ( 'NONE',  ( -0.000000000000000000, -0.000000000000000000, -1.000000000000000000 ) ) ;
#42866=ORIENTED_EDGE ( 'NONE', *, *, #8938, .T. ) ;
#42868=DIRECTION ( 'NONE',  ( 0.000000000000000000, 0.000000000000000000, -1.000000000000000000 ) ) ;
#42875=FILL_AREA_STYLE ('',( #110922 ) ) ;
#42949=VECTOR ( 'NONE', #16608, 1000.000000000000000 ) ;
#42985=SURFACE_STYLE_USAGE ( .BOTH. , #77750 ) ;
#42992=FACE_OUTER_BOUND ( 'NONE', #25366, .T. ) ;
#43003=FILL_AREA_STYLE_COLOUR ( '', #85552 ) ;
#43017=EDGE_CURVE ( 'NONE', #78237, #81439, #9727, .T. ) ;
#43080=CARTESIAN_POINT ( 'NONE',  ( 34.42500000000002558, -21.76999999999999247, -40.00000000000000000 ) ) ;
#43110=VERTEX_POINT ( 'NONE', #77181 ) ;
#43118=CARTESIAN_POINT ( 'NONE',  ( 4.838719539454570118, 11.93618569029472276, -25.72792102991144958 ) ) ;
#43139=DIRECTION ( 'NONE',  ( 1.000000000000000000, 0.000000000000000000, 0.000000000000000000 ) ) ;
#43143=AXIS2_PLACEMENT_3D ( 'NONE', #12877, #102051, #3421 ) ;
#43150=DIRECTION ( 'NONE',  ( 0.000000000000000000, 0.000000000000000000, 1.000000000000000000 ) ) ;
#43161=AXIS2_PLACEMENT_3D ( 'NONE', #74380, #48000, #4393 ) ;
#43221=DIRECTION ( 'NONE',  ( 0.000000000000000000, 0.000000000000000000, 1.000000000000000000 ) ) ;
#43312=PRESENTATION_STYLE_ASSIGNMENT (( #52733 ) ) ;
#43324=EDGE_CURVE ( 'NONE', #13983, #122313, #1062, .T. ) ;
#43330=CARTESIAN_POINT ( 'NONE',  ( -12.20000000000000462, -25.83999999999998565, 2.999999999999999112 ) ) ;
#43354=CARTESIAN_POINT ( 'NONE',  ( -31.92499999999997584, 0.4299755680429847016, -27.68972139052992176 ) ) ;
#43416=EDGE_LOOP ( 'NONE', ( #134284, #34276, #96263, #85856, #39693 ) ) ;
#43433=CARTESIAN_POINT ( 'NONE',  ( 19.92044161110034750, -3.134395820719624748, -35.08047115841593921 ) ) ;
#43449=DIRECTION ( 'NONE',  ( 0.000000000000000000, 1.000000000000000000, 0.000000000000000000 ) ) ;
#43480=EDGE_CURVE ( 'NONE', #81439, #112461, #19602, .T. ) ;
#43505=ORIENTED_EDGE ( 'NONE', *, *, #133372, .F. ) ;
#43517=DIRECTION ( 'NONE',  ( 0.000000000000000000, 0.000000000000000000, -1.000000000000000000 ) ) ;
#43521=ORIENTED_EDGE ( 'NONE', *, *, #122457, .F. ) ;
#43560=( NAMED_UNIT ( * ) PLANE_ANGLE_UNIT ( ) SI_UNIT ( $, .RADIAN. ) );
#43620=EDGE_LOOP ( 'NONE', ( #134121, #821, #10295, #7035 ) ) ;
#43628=DIRECTION ( 'NONE',  ( 0.000000000000000000, 0.000000000000000000, 1.000000000000000000 ) ) ;
#43669=VECTOR ( 'NONE', #16507, 1000.000000000000000 ) ;
#43741=B_SPLINE_CURVE_WITH_KNOTS ( 'NONE', 3,
 ( #89177, #76158, #77603, #120322 ),
 .UNSPECIFIED., .F., .F.,
 ( 4, 4 ),
 ( 0.001163520961193508819, 0.001596196080316354942 ),
 .UNSPECIFIED. ) ;
#43754=DIRECTION ( 'NONE',  ( 0.000000000000000000, 0.000000000000000000, -1.000000000000000000 ) ) ;
#43778=FACE_OUTER_BOUND ( 'NONE', #121669, .T. ) ;
#43819=CARTESIAN_POINT ( 'NONE',  ( -1.130389105715452036, 13.74331369484366761, -24.36998560215478804 ) ) ;
#43847=VECTOR ( 'NONE', #81621, 1000.000000000000114 ) ;
#43860=DIRECTION ( 'NONE',  ( -1.000000000000000000, 0.000000000000000000, 0.000000000000000000 ) ) ;
#43870=MECHANICAL_DESIGN_GEOMETRIC_PRESENTATION_REPRESENTATION('',(#138769),#80912);
#43912=ORIENTED_EDGE ( 'NONE', *, *, #96919, .T. ) ;
#44004=EDGE_CURVE ( 'NONE', #115328, #81524, #10795, .T. ) ;
#44063=EDGE_CURVE ( 'NONE', #38058, #85621, #60063, .T. ) ;
#44072=MECHANICAL_DESIGN_GEOMETRIC_PRESENTATION_REPRESENTATION('',(#4668),#69545);
#44101=FILL_AREA_STYLE_COLOUR ( '', #23832 ) ;
#44110=CARTESIAN_POINT ( 'NONE',  ( -7.940000000000007496, -60.26999999999998892, -10.00000000000000178 ) ) ;
#44159=CARTESIAN_POINT ( 'NONE',  ( 19.93618820137057668, -3.269999999999996465, -36.39086428169088094 ) ) ;
#44165=ORIENTED_EDGE ( 'NONE', *, *, #10016, .T. ) ;
#44179=VECTOR ( 'NONE', #103385, 1000.000000000000000 ) ;
#44194=EDGE_CURVE ( 'NONE', #113156, #38919, #57222, .T. ) ;
#44246=SURFACE_STYLE_USAGE ( .BOTH. , #98593 ) ;
#44271=CIRCLE ( 'NONE', #120582, 0.5000000000000004441 ) ;
#44272=( GEOMETRIC_REPRESENTATION_CONTEXT ( 3 ) GLOBAL_UNCERTAINTY_ASSIGNED_CONTEXT ( ( #27250 ) ) GLOBAL_UNIT_ASSIGNED_CONTEXT ( ( #109529, #43560, #132011 ) ) REPRESENTATION_CONTEXT ( 'NONE', 'WORKASPACE' ) );
#44307=CARTESIAN_POINT ( 'NONE',  ( -19.05499999999999261, 3.130000000000007887, 0.000000000000000000 ) ) ;
#44308=VERTEX_POINT ( 'NONE', #142440 ) ;
#44366=PRESENTATION_STYLE_ASSIGNMENT (( #79868 ) ) ;
#44374=EDGE_LOOP ( 'NONE', ( #111715, #105692, #121706, #139605, #27229, #64519 ) ) ;
#44422=CARTESIAN_POINT ( 'NONE',  ( 13.36114865838684374, 9.181040837666923693, -27.38535958397034520 ) ) ;
#44426=FILL_AREA_STYLE ('',( #52400 ) ) ;
#44489=SURFACE_STYLE_FILL_AREA ( #23397 ) ;
#44505=CARTESIAN_POINT ( 'NONE',  ( -34.42499999999997584, -22.26999999999999247, -0.5000000000000000000 ) ) ;
#44514=( NAMED_UNIT ( * ) SI_UNIT ( $, .STERADIAN. ) SOLID_ANGLE_UNIT ( ) );
#44544=EDGE_CURVE ( 'NONE', #86478, #92341, #116717, .T. ) ;
#44589=AXIS2_PLACEMENT_3D ( 'NONE', #97048, #28991, #108646 ) ;
#44600=CARTESIAN_POINT ( 'NONE',  ( -31.92499999999997584, -6.270000000000012008, -37.00000000000000000 ) ) ;
#44682=EDGE_CURVE ( 'NONE', #73050, #63324, #98315, .T. ) ;
#44703=VECTOR ( 'NONE', #72760, 1000.000000000000000 ) ;
#44726=VECTOR ( 'NONE', #113698, 1000.000000000000000 ) ;
#44727=DIRECTION ( 'NONE',  ( -1.321231229586337907E-16, 0.9647414015272155474, -0.2631995976047525887 ) ) ;
#44765=EDGE_CURVE ( 'NONE', #72919, #48675, #91388, .T. ) ;
#44774=ORIENTED_EDGE ( 'NONE', *, *, #14161, .F. ) ;
#44780=( NAMED_UNIT ( * ) SI_UNIT ( $, .STERADIAN. ) SOLID_ANGLE_UNIT ( ) );
#44781=CARTESIAN_POINT ( 'NONE',  ( 34.92500000000001137, 22.27000000000000668, 0.000000000000000000 ) ) ;
#44793=VECTOR ( 'NONE', #119035, 1000.000000000000000 ) ;
#44928=CYLINDRICAL_SURFACE ( 'NONE', #64485, 0.5000000000000000000 ) ;
#44943=VECTOR ( 'NONE', #50989, 1000.000000000000000 ) ;
#44964=EDGE_LOOP ( 'NONE', ( #116382, #25883, #119043, #40097 ) ) ;
#44980=EDGE_CURVE ( 'NONE', #106369, #22146, #102963, .T. ) ;
#44985=CARTESIAN_POINT ( 'NONE',  ( 0.000000000000000000, -21.76999999999999247, -0.5000000000000000000 ) ) ;
#45026=CONICAL_SURFACE ( 'NONE', #135243, 1.898649999999993065, 1.029744258676648316 ) ;
#45122=LINE ( 'NONE', #98726, #137524 ) ;
#45142=EDGE_CURVE ( 'NONE', #59938, #109867, #17755, .T. ) ;
#45144=CARTESIAN_POINT ( 'NONE',  ( 18.46695620621371248, 3.075185539296316328, -30.04948271178109920 ) ) ;
#45150=SURFACE_STYLE_USAGE ( .BOTH. , #102367 ) ;
#45155=DIRECTION ( 'NONE',  ( -1.000000000000000000, 0.000000000000000000, 0.000000000000000000 ) ) ;
#45168=EDGE_CURVE ( 'NONE', #118671, #25909, #49732, .T. ) ;
#45206=PLANE ( 'NONE',  #42101 ) ;
#45228=ORIENTED_EDGE ( 'NONE', *, *, #22518, .T. ) ;
#45229=FACE_OUTER_BOUND ( 'NONE', #71596, .T. ) ;
#45248=EDGE_CURVE ( 'NONE', #142234, #13538, #24310, .T. ) ;
#45266=DIRECTION ( 'NONE',  ( 1.000000000000000000, 0.000000000000000000, 0.000000000000000000 ) ) ;
#45302=DIRECTION ( 'NONE',  ( 0.000000000000000000, 1.000000000000000000, -0.000000000000000000 ) ) ;
#45321=EDGE_LOOP ( 'NONE', ( #5267, #8891, #2598, #17004 ) ) ;
#45340=CARTESIAN_POINT ( 'NONE',  ( -12.20000000000000284, -40.42999999999999261, -39.50000000000000000 ) ) ;
#45344=ORIENTED_EDGE ( 'NONE', *, *, #65059, .F. ) ;
#45395=CARTESIAN_POINT ( 'NONE',  ( -31.92499999999997584, 0.000000000000000000, -37.00000000000000000 ) ) ;
#45418=PRESENTATION_STYLE_ASSIGNMENT (( #51454 ) ) ;
#45447=SURFACE_SIDE_STYLE ('',( #56343 ) ) ;
#45500=CARTESIAN_POINT ( 'NONE',  ( 16.99919035942976109, -0.8850635513006737121, -35.72698641301105482 ) ) ;
#45547=DIRECTION ( 'NONE',  ( 0.000000000000000000, -1.000000000000000000, -1.734723475976807686E-15 ) ) ;
#45555=AXIS2_PLACEMENT_3D ( 'NONE', #137918, #70553, #135088 ) ;
#45585=DIRECTION ( 'NONE',  ( 0.000000000000000000, 0.000000000000000000, -1.000000000000000000 ) ) ;
#45615=STYLED_ITEM ( 'NONE', ( #44366 ), #106840 ) ;
#45748=EDGE_CURVE ( 'NONE', #140981, #64204, #132888, .T. ) ;
#45770=EDGE_CURVE ( 'NONE', #95348, #2907, #45122, .T. ) ;
#45788=DIRECTION ( 'NONE',  ( 1.369518533665900312E-16, -1.000000000000000000, 0.000000000000000000 ) ) ;
#45802=( LENGTH_UNIT ( ) NAMED_UNIT ( * ) SI_UNIT ( .MILLI., .METRE. ) );
#45899=ORIENTED_EDGE ( 'NONE', *, *, #109914, .F. ) ;
#45926=CARTESIAN_POINT ( 'NONE',  ( 34.92500000000001137, 22.27000000000000668, -7.752744394707098863 ) ) ;
#45931=STYLED_ITEM ( 'NONE', ( #126375 ), #125643 ) ;
#45994=COLOUR_RGB ( '', 0.72549020, 0.75294118, 0.79215686) ;
#46086=CARTESIAN_POINT ( 'NONE',  ( 7.139999999999985469, -39.92999999999999972, -40.00000000000000000 ) ) ;
#46089=COLOUR_RGB ( '', 0.66274510, 0.83137255, 0.94901961) ;
#46102=CARTESIAN_POINT ( 'NONE',  ( -16.85442536677114589, -0.3105974261732821762, -34.40776350357948132 ) ) ;
#46155=COLOUR_RGB ( '', 0.72549020, 0.75294118, 0.79215686) ;
#46166=COLOUR_RGB ( '', 0.31764706, 0.68627451, 0.89019608) ;
#46224=UNCERTAINTY_MEASURE_WITH_UNIT (LENGTH_MEASURE( 1.000000000000000082E-05 ), #48368, 'distance_accuracy_value', 'NONE');
#46246=CIRCLE ( 'NONE', #115594, 1.898649999999993065 ) ;
#46260=SURFACE_STYLE_USAGE ( .BOTH. , #55689 ) ;
#46349=ORIENTED_EDGE ( 'NONE', *, *, #79772, .F. ) ;
#46356=CARTESIAN_POINT ( 'NONE',  ( -12.70000000000000284, -40.42999999999999261, -40.00000000000000000 ) ) ;
#46391=SURFACE_SIDE_STYLE ('',( #57255 ) ) ;
#46403=DIRECTION ( 'NONE',  ( 1.000000000000000000, 0.000000000000000000, 0.000000000000000000 ) ) ;
#46455=EDGE_LOOP ( 'NONE', ( #93738, #136765, #82072 ) ) ;
#46465=EDGE_CURVE ( 'NONE', #118785, #16702, #81892, .T. ) ;
#46529=SURFACE_STYLE_FILL_AREA ( #66 ) ;
#46568=ORIENTED_EDGE ( 'NONE', *, *, #64101, .T. ) ;
#46623=EDGE_CURVE ( 'NONE', #117264, #103756, #56198, .T. ) ;
#46674=CIRCLE ( 'NONE', #35053, 0.5000000000000004441 ) ;
#46696=VERTEX_POINT ( 'NONE', #137294 ) ;
#46712=CARTESIAN_POINT ( 'NONE',  ( 0.000000000000000000, -4.870000000000014317, -40.00000000000000000 ) ) ;
#46732=CARTESIAN_POINT ( 'NONE',  ( 14.88812247636860064, 4.294539510182263875, -29.64274772238085021 ) ) ;
#46746=CYLINDRICAL_SURFACE ( 'NONE', #11099, 2.247899999999996901 ) ;
#46768=( NAMED_UNIT ( * ) PLANE_ANGLE_UNIT ( ) SI_UNIT ( $, .RADIAN. ) );
#46773=DIRECTION ( 'NONE',  ( -0.000000000000000000, -1.000000000000000000, -0.000000000000000000 ) ) ;
#46786=MECHANICAL_DESIGN_GEOMETRIC_PRESENTATION_REPRESENTATION('',(#60638),#106832);
#46846=CARTESIAN_POINT ( 'NONE',  ( -19.61417773406576259, -0.8225097182635713322, -31.54462512304873911 ) ) ;
#46874=AXIS2_PLACEMENT_3D ( 'NONE', #33717, #57611, #122111 ) ;
#46901=EDGE_CURVE ( 'NONE', #142234, #106369, #7451, .T. ) ;
#46914=AXIS2_PLACEMENT_3D ( 'NONE', #20600, #54694, #76449 ) ;
#46944=CARTESIAN_POINT ( 'NONE',  ( 34.92500000000001137, 22.27000000000000668, -7.752744394707098863 ) ) ;
#46949=FACE_OUTER_BOUND ( 'NONE', #62168, .T. ) ;
#47031=( GEOMETRIC_REPRESENTATION_CONTEXT ( 3 ) GLOBAL_UNCERTAINTY_ASSIGNED_CONTEXT ( ( #46224 ) ) GLOBAL_UNIT_ASSIGNED_CONTEXT ( ( #48368, #103441, #91195 ) ) REPRESENTATION_CONTEXT ( 'NONE', 'WORKASPACE' ) );
#47071=ORIENTED_EDGE ( 'NONE', *, *, #87905, .F. ) ;
#47075=ADVANCED_FACE ( 'NONE', ( #104464 ), #25219, .F. ) ;
#47091=ORIENTED_EDGE ( 'NONE', *, *, #45770, .F. ) ;
#47151=DIRECTION ( 'NONE',  ( -1.000000000000000000, 2.496005001405478586E-15, 0.000000000000000000 ) ) ;
#47208=TOROIDAL_SURFACE ( 'NONE', #128188, 31.92999999999999261, 3.000000000000000000 ) ;
#47250=( NAMED_UNIT ( * ) PLANE_ANGLE_UNIT ( ) SI_UNIT ( $, .RADIAN. ) );
#47252=CYLINDRICAL_SURFACE ( 'NONE', #38652, 3.000000000000000000 ) ;
#47290=FACE_OUTER_BOUND ( 'NONE', #15476, .T. ) ;
#47301=CARTESIAN_POINT ( 'NONE',  ( 8.131392392196376662, 12.20025264268591059, -25.50689499364121815 ) ) ;
#47318=DIRECTION ( 'NONE',  ( -1.000000000000000000, -3.115803279706882722E-16, 0.000000000000000000 ) ) ;
#47351=LINE ( 'NONE', #26259, #138774 ) ;
#47387=DIRECTION ( 'NONE',  ( -1.369518533665900312E-16, 1.000000000000000000, -0.000000000000000000 ) ) ;
#47414=SURFACE_STYLE_FILL_AREA ( #59684 ) ;
#47440=CIRCLE ( 'NONE', #123781, 1.898649999999993065 ) ;
#47449=ORIENTED_EDGE ( 'NONE', *, *, #77395, .T. ) ;
#47493=LINE ( 'NONE', #113392, #60028 ) ;
#47509=AXIS2_PLACEMENT_3D ( 'NONE', #70170, #79626, #24465 ) ;
#47523=ADVANCED_FACE ( 'NONE', ( #7087 ), #75963, .F. ) ;
#47528=DIRECTION ( 'NONE',  ( 0.000000000000000000, 1.000000000000000000, 0.000000000000000000 ) ) ;
#47536=DIRECTION ( 'NONE',  ( -0.000000000000000000, -0.000000000000000000, -1.000000000000000000 ) ) ;
#47555=CARTESIAN_POINT ( 'NONE',  ( -16.67979525387082518, 0.3337821591035555757, -30.81818940114110461 ) ) ;
#47591=ORIENTED_EDGE ( 'NONE', *, *, #62674, .F. ) ;
#47614=ORIENTED_EDGE ( 'NONE', *, *, #74973, .F. ) ;
#47651=CARTESIAN_POINT ( 'NONE',  ( 19.28515664589288292, 1.196650378695334416, -30.59010235425024149 ) ) ;
#47664=UNCERTAINTY_MEASURE_WITH_UNIT (LENGTH_MEASURE( 1.000000000000000082E-05 ), #127656, 'distance_accuracy_value', 'NONE');
#47667=EDGE_CURVE ( 'NONE', #122541, #79346, #10668, .T. ) ;
#47701=( BOUNDED_CURVE ( )  B_SPLINE_CURVE ( 3, ( #52974, #20343, #75475, #74777 ),
 .UNSPECIFIED., .F., .T. ) 
 B_SPLINE_CURVE_WITH_KNOTS ( ( 4, 4 ),
 ( 3.141592653589795336, 4.712388980384686121 ),
 .UNSPECIFIED. ) 
 CURVE ( )  GEOMETRIC_REPRESENTATION_ITEM ( )  RATIONAL_B_SPLINE_CURVE ( ( 1.000000000000000000, 0.8047378541243663808, 0.8047378541243663808, 1.000000000000000000 ) ) 
 REPRESENTATION_ITEM ( '' )  );
#47785=CARTESIAN_POINT ( 'NONE',  ( -34.92499999999997584, -22.26999999999999247, -37.00000000000000000 ) ) ;
#47826=DIRECTION ( 'NONE',  ( -0.000000000000000000, -0.000000000000000000, -1.000000000000000000 ) ) ;
#47843=CARTESIAN_POINT ( 'NONE',  ( 0.000000000000000000, -22.26999999999999247, -0.5000000000000004441 ) ) ;
#47935=CYLINDRICAL_SURFACE ( 'NONE', #130197, 2.999999999999999112 ) ;
#47937=SURFACE_STYLE_USAGE ( .BOTH. , #77864 ) ;
#47975=EDGE_CURVE ( 'NONE', #878, #121504, #62503, .T. ) ;
#47978=ORIENTED_EDGE ( 'NONE', *, *, #71272, .T. ) ;
#47984=ORIENTED_EDGE ( 'NONE', *, *, #80069, .F. ) ;
#47985=CARTESIAN_POINT ( 'NONE',  ( -18.91353603094692204, 2.162493570128502185, -30.33479532556184211 ) ) ;
#47992=LINE ( 'NONE', #77935, #69344 ) ;
#48000=DIRECTION ( 'NONE',  ( -0.000000000000000000, -0.000000000000000000, 1.000000000000000000 ) ) ;
#48045=FILL_AREA_STYLE_COLOUR ( '', #97635 ) ;
#48065=CIRCLE ( 'NONE', #140551, 3.000000000000002665 ) ;
#48070=( NAMED_UNIT ( * ) SI_UNIT ( $, .STERADIAN. ) SOLID_ANGLE_UNIT ( ) );
#48074=VERTEX_POINT ( 'NONE', #3718 ) ;
#48121=DIRECTION ( 'NONE',  ( -1.000000000000000000, 0.000000000000000000, 0.000000000000000000 ) ) ;
#48139=ORIENTED_EDGE ( 'NONE', *, *, #44544, .T. ) ;
#48189=ORIENTED_EDGE ( 'NONE', *, *, #79247, .T. ) ;
#48214=FACE_OUTER_BOUND ( 'NONE', #57221, .T. ) ;
#48262=CARTESIAN_POINT ( 'NONE',  ( -16.15307943227677612, 1.820290827408419521, -33.22442919644333870 ) ) ;
#48279=EDGE_CURVE ( 'NONE', #39230, #23998, #6861, .T. ) ;
#48311=AXIS2_PLACEMENT_3D ( 'NONE', #1758, #23560, #112711 ) ;
#48324=AXIS2_PLACEMENT_3D ( 'NONE', #640, #12236, #123891 ) ;
#48336=AXIS2_PLACEMENT_3D ( 'NONE', #59510, #29001, #137045 ) ;
#48368=( LENGTH_UNIT ( ) NAMED_UNIT ( * ) SI_UNIT ( .MILLI., .METRE. ) );
#48379=EDGE_CURVE ( 'NONE', #69904, #122313, #30529, .T. ) ;
#48404=ORIENTED_EDGE ( 'NONE', *, *, #94870, .T. ) ;
#48432=VECTOR ( 'NONE', #86704, 1000.000000000000000 ) ;
#48499=CARTESIAN_POINT ( 'NONE',  ( 9.524999999999995026, -4.870000000000013429, -40.00000000000000000 ) ) ;
#48532=CARTESIAN_POINT ( 'NONE',  ( 7.139999999999956160, -35.56014942880460694, -11.72188031596273206 ) ) ;
#48556=SURFACE_STYLE_USAGE ( .BOTH. , #81937 ) ;
#48560=DIRECTION ( 'NONE',  ( 0.000000000000000000, -1.000000000000000000, 0.000000000000000000 ) ) ;
#48563=ORIENTED_EDGE ( 'NONE', *, *, #42043, .F. ) ;
#48569=ORIENTED_EDGE ( 'NONE', *, *, #13335, .F. ) ;
#48591=CIRCLE ( 'NONE', #4540, 2.999999999999999112 ) ;
#48592=( GEOMETRIC_REPRESENTATION_CONTEXT ( 3 ) GLOBAL_UNCERTAINTY_ASSIGNED_CONTEXT ( ( #91150 ) ) GLOBAL_UNIT_ASSIGNED_CONTEXT ( ( #71137, #136363, #138520 ) ) REPRESENTATION_CONTEXT ( 'NONE', 'WORKASPACE' ) );
#48620=( LENGTH_UNIT ( ) NAMED_UNIT ( * ) SI_UNIT ( .MILLI., .METRE. ) );
#48657=ORIENTED_EDGE ( 'NONE', *, *, #66430, .T. ) ;
#48658=SURFACE_STYLE_USAGE ( .BOTH. , #50093 ) ;
#48675=VERTEX_POINT ( 'NONE', #17316 ) ;
#48691=CARTESIAN_POINT ( 'NONE',  ( -31.92499999999997584, -7.730000000000015525, 3.180000000000000160 ) ) ;
#48718=AXIS2_PLACEMENT_3D ( 'NONE', #77617, #66722, #130563 ) ;
#48725=CARTESIAN_POINT ( 'NONE',  ( -7.140000000000001457, -35.13237070076360169, 17.62370837922860289 ) ) ;
#48727=ORIENTED_EDGE ( 'NONE', *, *, #8257, .T. ) ;
#48737=CARTESIAN_POINT ( 'NONE',  ( 12.19999999999999574, -27.55040120718572894, 16.07347811296898854 ) ) ;
#48747=ORIENTED_EDGE ( 'NONE', *, *, #72922, .T. ) ;
#48749=ADVANCED_FACE ( 'NONE', ( #29607 ), #30338, .T. ) ;
#48775=ORIENTED_EDGE ( 'NONE', *, *, #74636, .T. ) ;
#48784=DIRECTION ( 'NONE',  ( -1.000000000000000000, -3.115803279706882722E-16, 0.000000000000000000 ) ) ;
#48797=CYLINDRICAL_SURFACE ( 'NONE', #49644, 0.5000000000000004441 ) ;
#48808=SURFACE_STYLE_FILL_AREA ( #16124 ) ;
#48871=LINE ( 'NONE', #25665, #11152 ) ;
#48891=UNCERTAINTY_MEASURE_WITH_UNIT (LENGTH_MEASURE( 1.000000000000000082E-05 ), #35470, 'distance_accuracy_value', 'NONE');
#48917=AXIS2_PLACEMENT_3D ( 'NONE', #107998, #29735, #119592 ) ;
#48951=AXIS2_PLACEMENT_3D ( 'NONE', #77365, #98373, #133159 ) ;
#48995=CARTESIAN_POINT ( 'NONE',  ( -13.33265045070550237, 6.437115738644505925, -28.78119739759756968 ) ) ;
#49012=EDGE_CURVE ( 'NONE', #109349, #129328, #125193, .T. ) ;
#49020=AXIS2_PLACEMENT_3D ( 'NONE', #109666, #10340, #54594 ) ;
#49070=STYLED_ITEM ( 'NONE', ( #105300 ), #25816 ) ;
#49109=FILL_AREA_STYLE_COLOUR ( '', #130286 ) ;
#49116=DIRECTION ( 'NONE',  ( 0.000000000000000000, 0.000000000000000000, -1.000000000000000000 ) ) ;
#49126=ORIENTED_EDGE ( 'NONE', *, *, #135087, .F. ) ;
#49275=MECHANICAL_DESIGN_GEOMETRIC_PRESENTATION_REPRESENTATION('',(#102555),#47031);
#49320=EDGE_CURVE ( 'NONE', #9707, #1800, #62074, .T. ) ;
#49363=DIRECTION ( 'NONE',  ( 0.000000000000000000, 0.000000000000000000, -1.000000000000000000 ) ) ;
#49372=ORIENTED_EDGE ( 'NONE', *, *, #45248, .F. ) ;
#49383=CARTESIAN_POINT ( 'NONE',  ( 12.19999999999999574, -59.76999999999998892, -40.00000000000000000 ) ) ;
#49420=VECTOR ( 'NONE', #120553, 1000.000000000000114 ) ;
#49421=CARTESIAN_POINT ( 'NONE',  ( -8.173355474122208975, 12.20286799362002483, -25.50874979209409688 ) ) ;
#49434=DIRECTION ( 'NONE',  ( -0.000000000000000000, -1.000000000000000000, -0.000000000000000000 ) ) ;
#49461=DIRECTION ( 'NONE',  ( 0.000000000000000000, 0.000000000000000000, 1.000000000000000000 ) ) ;
#49543=( LENGTH_UNIT ( ) NAMED_UNIT ( * ) SI_UNIT ( .MILLI., .METRE. ) );
#49589=AXIS2_PLACEMENT_3D ( 'NONE', #77023, #134240, #89299 ) ;
#49599=LINE ( 'NONE', #8163, #103831 ) ;
#49644=AXIS2_PLACEMENT_3D ( 'NONE', #22883, #33820, #133834 ) ;
#49656=CARTESIAN_POINT ( 'NONE',  ( -17.01299345042646749, -0.9444868035190713274, -36.39086428169088094 ) ) ;
#49726=CARTESIAN_POINT ( 'NONE',  ( -8.727265903332346753, 10.25892755801883638, -28.67759622474984127 ) ) ;
#49728=EDGE_CURVE ( 'NONE', #1800, #132295, #114118, .T. ) ;
#49732=LINE ( 'NONE', #137436, #137843 ) ;
#49735=ORIENTED_EDGE ( 'NONE', *, *, #56252, .T. ) ;
#49738=CARTESIAN_POINT ( 'NONE',  ( -14.08979869950237251, -1.618973607074043919, -40.00000000000000000 ) ) ;
#49792=DIRECTION ( 'NONE',  ( -1.000000000000000000, -1.369518533665900312E-16, 0.000000000000000000 ) ) ;
#49818=DIRECTION ( 'NONE',  ( 0.000000000000000000, 1.000000000000000000, 0.000000000000000000 ) ) ;
#49868=CARTESIAN_POINT ( 'NONE',  ( 12.69999999999999574, -35.15000000000000568, -39.50000000000000000 ) ) ;
#49884=VECTOR ( 'NONE', #99324, 1000.000000000000000 ) ;
#49885=ADVANCED_FACE ( 'NONE', ( #136947 ), #37658, .T. ) ;
#49887=( NAMED_UNIT ( * ) PLANE_ANGLE_UNIT ( ) SI_UNIT ( $, .RADIAN. ) );
#49920=DIRECTION ( 'NONE',  ( 0.000000000000000000, -0.000000000000000000, 1.000000000000000000 ) ) ;
#49922=ORIENTED_EDGE ( 'NONE', *, *, #54979, .F. ) ;
#49956=( LENGTH_UNIT ( ) NAMED_UNIT ( * ) SI_UNIT ( .MILLI., .METRE. ) );
#49966=SURFACE_SIDE_STYLE ('',( #5700 ) ) ;
#49968=ORIENTED_EDGE ( 'NONE', *, *, #131135, .F. ) ;
#50061=DIRECTION ( 'NONE',  ( -0.000000000000000000, -0.000000000000000000, -1.000000000000000000 ) ) ;
#50065=EDGE_LOOP ( 'NONE', ( #4482, #9398, #137489, #72436 ) ) ;
#50093=SURFACE_SIDE_STYLE ('',( #125507 ) ) ;
#50098=DIRECTION ( 'NONE',  ( 1.000000000000000000, -1.451651444332054676E-15, 0.000000000000000000 ) ) ;
#50148=( NAMED_UNIT ( * ) PLANE_ANGLE_UNIT ( ) SI_UNIT ( $, .RADIAN. ) );
#50190=AXIS2_PLACEMENT_3D ( 'NONE', #75500, #29132, #97202 ) ;
#50202=EDGE_CURVE ( 'NONE', #237, #70779, #120206, .T. ) ;
#50266=DIRECTION ( 'NONE',  ( 0.000000000000000000, 0.000000000000000000, 1.000000000000000000 ) ) ;
#50307=CARTESIAN_POINT ( 'NONE',  ( 7.139999999999992575, -35.14999999999999858, -11.72188031596274804 ) ) ;
#50410=VERTEX_POINT ( 'NONE', #6929 ) ;
#50412=EDGE_CURVE ( 'NONE', #122541, #113921, #34538, .T. ) ;
#50420=CARTESIAN_POINT ( 'NONE',  ( -11.45531355849511002, 8.356207601636546300, -27.86682228225575031 ) ) ;
#50433=LINE ( 'NONE', #82353, #41489 ) ;
#50435=DIRECTION ( 'NONE',  ( -0.000000000000000000, -1.000000000000000000, -0.000000000000000000 ) ) ;
#50440=ORIENTED_EDGE ( 'NONE', *, *, #31379, .T. ) ;
#50470=LINE ( 'NONE', #74371, #30487 ) ;
#50553=CYLINDRICAL_SURFACE ( 'NONE', #112286, 3.000000000000000000 ) ;
#50565=CYLINDRICAL_SURFACE ( 'NONE', #11707, 0.5000000000000004441 ) ;
#50570=EDGE_CURVE ( 'NONE', #99547, #109349, #65699, .T. ) ;
#50587=VECTOR ( 'NONE', #89485, 1000.000000000000000 ) ;
#50602=LINE ( 'NONE', #47785, #66371 ) ;
#50603=AXIS2_PLACEMENT_3D ( 'NONE', #37762, #127614, #60230 ) ;
#50605=CARTESIAN_POINT ( 'NONE',  ( -12.70000000000000284, -34.64999999999999147, -40.00000000000000000 ) ) ;
#50622=CARTESIAN_POINT ( 'NONE',  ( -12.70000000000000462, -22.26999999999999247, -0.2071067811865474895 ) ) ;
#50652=CARTESIAN_POINT ( 'NONE',  ( -12.70000000000000284, -40.42999999999999261, -39.50000000000000000 ) ) ;
#50744=FILL_AREA_STYLE_COLOUR ( '', #102424 ) ;
#50752=CYLINDRICAL_SURFACE ( 'NONE', #48336, 0.5000000000000004441 ) ;
#50794=FACE_OUTER_BOUND ( 'NONE', #90884, .T. ) ;
#50802=CYLINDRICAL_SURFACE ( 'NONE', #106088, 0.5000000000000004441 ) ;
#50811=MECHANICAL_DESIGN_GEOMETRIC_PRESENTATION_REPRESENTATION('',(#108712),#62414);
#50834=( LENGTH_UNIT ( ) NAMED_UNIT ( * ) SI_UNIT ( .MILLI., .METRE. ) );
#50859=CARTESIAN_POINT ( 'NONE',  ( -12.20000000000000284, -40.42999999999999261, 19.06900128115122328 ) ) ;
#50924=VERTEX_POINT ( 'NONE', #40191 ) ;
#50936=CARTESIAN_POINT ( 'NONE',  ( -7.140000000000000568, -35.14999999999999147, -39.79289321881344677 ) ) ;
#50989=DIRECTION ( 'NONE',  ( -1.000000000000000000, 0.000000000000000000, -0.000000000000000000 ) ) ;
#51053=CARTESIAN_POINT ( 'NONE',  ( -7.140000000000001457, -60.26999999999998892, -11.72188031596275337 ) ) ;
#51080=( NAMED_UNIT ( * ) SI_UNIT ( $, .STERADIAN. ) SOLID_ANGLE_UNIT ( ) );
#51116=CARTESIAN_POINT ( 'NONE',  ( -34.92499999999999005, -3.270000000000012896, -40.00000000000000000 ) ) ;
#51135=CARTESIAN_POINT ( 'NONE',  ( -14.91938099157687958, 4.277364139441302449, -29.65621814313812976 ) ) ;
#51155=FACE_OUTER_BOUND ( 'NONE', #122490, .T. ) ;
#51186=CARTESIAN_POINT ( 'NONE',  ( -55.65468426143998215, -60.26999999999998892, 25.00000000000000000 ) ) ;
#51220=( GEOMETRIC_REPRESENTATION_CONTEXT ( 3 ) GLOBAL_UNCERTAINTY_ASSIGNED_CONTEXT ( ( #54778 ) ) GLOBAL_UNIT_ASSIGNED_CONTEXT ( ( #16091, #38608, #82143 ) ) REPRESENTATION_CONTEXT ( 'NONE', 'WORKASPACE' ) );
#51278=EDGE_LOOP ( 'NONE', ( #21058, #123138, #141952 ) ) ;
#51304=VERTEX_POINT ( 'NONE', #33591 ) ;
#51326=CARTESIAN_POINT ( 'NONE',  ( -7.140000000000001457, 12.19802518668052471, 4.711086268963008195 ) ) ;
#51366=( NAMED_UNIT ( * ) PLANE_ANGLE_UNIT ( ) SI_UNIT ( $, .RADIAN. ) );
#51391=( LENGTH_UNIT ( ) NAMED_UNIT ( * ) SI_UNIT ( .MILLI., .METRE. ) );
#51425=STYLED_ITEM ( 'NONE', ( #123669 ), #54318 ) ;
#51432=CARTESIAN_POINT ( 'NONE',  ( 19.28515664589288647, 1.196650378695337302, -30.59010235425025215 ) ) ;
#51454=SURFACE_STYLE_USAGE ( .BOTH. , #78733 ) ;
#51464=LINE ( 'NONE', #7919, #117471 ) ;
#51486=LINE ( 'NONE', #129020, #66859 ) ;
#51527=STYLED_ITEM ( 'NONE', ( #261 ), #100104 ) ;
#51534=CYLINDRICAL_SURFACE ( 'NONE', #35129, 0.5000000000000004441 ) ;
#51550=CYLINDRICAL_SURFACE ( 'NONE', #141569, 0.5000000000000001110 ) ;
#51598=DIRECTION ( 'NONE',  ( 0.000000000000000000, -1.000000000000000000, 0.000000000000000000 ) ) ;
#51608=AXIS2_PLACEMENT_3D ( 'NONE', #72654, #76730, #95048 ) ;
#51613=EDGE_CURVE ( 'NONE', #135652, #96844, #52955, .T. ) ;
#51615=ORIENTED_EDGE ( 'NONE', *, *, #38078, .F. ) ;
#51640=CARTESIAN_POINT ( 'NONE',  ( 7.940000000000001279, -33.26999999999999602, -10.00000000000000178 ) ) ;
#51647=ORIENTED_EDGE ( 'NONE', *, *, #126095, .F. ) ;
#51734=EDGE_CURVE ( 'NONE', #48675, #117423, #143526, .T. ) ;
#51740=( NAMED_UNIT ( * ) PLANE_ANGLE_UNIT ( ) SI_UNIT ( $, .RADIAN. ) );
#51819=SURFACE_STYLE_FILL_AREA ( #8949 ) ;
#51854=CARTESIAN_POINT ( 'NONE',  ( 12.81928177610584640, 7.016045820313829395, -30.84182252500521315 ) ) ;
#51857=ADVANCED_FACE ( 'NONE', ( #18555 ), #70856, .T. ) ;
#51873=ORIENTED_EDGE ( 'NONE', *, *, #79857, .F. ) ;
#51947=CARTESIAN_POINT ( 'NONE',  ( -7.940000000000007496, -39.92999999999999261, -10.00000000000000178 ) ) ;
#51957=ORIENTED_EDGE ( 'NONE', *, *, #133563, .T. ) ;
#52052=CARTESIAN_POINT ( 'NONE',  ( -34.92499999999997584, -21.76999999999999247, -0.5000000000000000000 ) ) ;
#52074=UNCERTAINTY_MEASURE_WITH_UNIT (LENGTH_MEASURE( 1.000000000000000082E-05 ), #53104, 'distance_accuracy_value', 'NONE');
#52092=CARTESIAN_POINT ( 'NONE',  ( 0.000000000000000000, -4.870000000000014317, 500000.0000000000582 ) ) ;
#52108=AXIS2_PLACEMENT_3D ( 'NONE', #110034, #56441, #45547 ) ;
#52122=ORIENTED_EDGE ( 'NONE', *, *, #67754, .F. ) ;
#52161=CARTESIAN_POINT ( 'NONE',  ( 19.49365931317388245, -0.02952910816523741239, -31.02252017457930577 ) ) ;
#52165=EDGE_LOOP ( 'NONE', ( #915, #14299, #12695, #110439, #19463, #53031 ) ) ;
#52169=FACE_OUTER_BOUND ( 'NONE', #14667, .T. ) ;
#52197=DIRECTION ( 'NONE',  ( 0.000000000000000000, 0.000000000000000000, 1.000000000000000000 ) ) ;
#52224=DIRECTION ( 'NONE',  ( 0.000000000000000000, 0.000000000000000000, -1.000000000000000000 ) ) ;
#52243=CARTESIAN_POINT ( 'NONE',  ( -16.50229999999999464, 3.130000000000007887, -2.396719511207313368E-16 ) ) ;
#52269=( NAMED_UNIT ( * ) SI_UNIT ( $, .STERADIAN. ) SOLID_ANGLE_UNIT ( ) );
#52281=EDGE_CURVE ( 'NONE', #106633, #56871, #22925, .T. ) ;
#52314=ORIENTED_EDGE ( 'NONE', *, *, #92959, .F. ) ;
#52346=AXIS2_PLACEMENT_3D ( 'NONE', #71009, #115158, #13012 ) ;
#52383=CARTESIAN_POINT ( 'NONE',  ( 12.69999999999999574, -25.83999999999998565, 13.17925390838734323 ) ) ;
#52387=CARTESIAN_POINT ( 'NONE',  ( -19.87251829384141288, -2.732064206673406659, -33.82029841778192747 ) ) ;
#52400=FILL_AREA_STYLE_COLOUR ( '', #1907 ) ;
#52420=( NAMED_UNIT ( * ) SI_UNIT ( $, .STERADIAN. ) SOLID_ANGLE_UNIT ( ) );
#52462=CARTESIAN_POINT ( 'NONE',  ( -17.00355154389407275, -0.9028365174813322014, -35.76436417572673321 ) ) ;
#52503=PRESENTATION_STYLE_ASSIGNMENT (( #28642 ) ) ;
#52523=EDGE_LOOP ( 'NONE', ( #127725, #63305, #100991 ) ) ;
#52541=CARTESIAN_POINT ( 'NONE',  ( 0.8904098635733341816, 12.57359452820395163, -26.74927803365304868 ) ) ;
#52583=AXIS2_PLACEMENT_3D ( 'NONE', #44110, #133960, #36099 ) ;
#52597=FILL_AREA_STYLE_COLOUR ( '', #117029 ) ;
#52615=VECTOR ( 'NONE', #82842, 1000.000000000000000 ) ;
#52690=ORIENTED_EDGE ( 'NONE', *, *, #18226, .F. ) ;
#52733=SURFACE_STYLE_USAGE ( .BOTH. , #142621 ) ;
#52749=ORIENTED_EDGE ( 'NONE', *, *, #56951, .T. ) ;
#52769=CARTESIAN_POINT ( 'NONE',  ( 31.92500000000001492, -7.729999999999995985, 3.180000000000000160 ) ) ;
#52782=SURFACE_SIDE_STYLE ('',( #53528 ) ) ;
#52785=CARTESIAN_POINT ( 'NONE',  ( 31.92500000000001492, -7.729999999999995985, 3.180000000000000160 ) ) ;
#52847=CONICAL_SURFACE ( 'NONE', #48324, 2.552699999999994418, 1.029744258676651869 ) ;
#52898=CARTESIAN_POINT ( 'NONE',  ( -31.92499999999997584, 1.196650378695321315, -30.59010235425025215 ) ) ;
#52909=CARTESIAN_POINT ( 'NONE',  ( -12.20000000000000817, -1.670812611072399357E-15, -0.5000000000000000000 ) ) ;
#52955=CIRCLE ( 'NONE', #134010, 0.5000000000000000000 ) ;
#52956=( BOUNDED_CURVE ( )  B_SPLINE_CURVE ( 3, ( #89072, #141277, #19504, #131133 ),
 .UNSPECIFIED., .F., .T. ) 
 B_SPLINE_CURVE_WITH_KNOTS ( ( 4, 4 ),
 ( 4.712388980384696779, 6.283185307179586232 ),
 .UNSPECIFIED. ) 
 CURVE ( )  GEOMETRIC_REPRESENTATION_ITEM ( )  RATIONAL_B_SPLINE_CURVE ( ( 1.000000000000000000, 0.8047378541243667138, 0.8047378541243667138, 1.000000000000000000 ) ) 
 REPRESENTATION_ITEM ( '' )  );
#52965=CARTESIAN_POINT ( 'NONE',  ( 1.868077901080408498, 12.49629736921268552, -26.81958028572744723 ) ) ;
#52974=CARTESIAN_POINT ( 'NONE',  ( 7.139999999999992575, -35.13237070076360169, 17.62370837922859934 ) ) ;
#53016=LINE ( 'NONE', #74086, #104695 ) ;
#53031=ORIENTED_EDGE ( 'NONE', *, *, #10429, .T. ) ;
#53095=EDGE_CURVE ( 'NONE', #9707, #70234, #128950, .T. ) ;
#53104=( LENGTH_UNIT ( ) NAMED_UNIT ( * ) SI_UNIT ( .MILLI., .METRE. ) );
#53123=AXIS2_PLACEMENT_3D ( 'NONE', #60427, #93737, #38648 ) ;
#53127=( NAMED_UNIT ( * ) PLANE_ANGLE_UNIT ( ) SI_UNIT ( $, .RADIAN. ) );
#53195=DIRECTION ( 'NONE',  ( 1.000000000000000000, 0.000000000000000000, 0.000000000000000000 ) ) ;
#53197=EDGE_LOOP ( 'NONE', ( #131674, #7987, #98706, #4283, #128010, #29545, #35796, #138869 ) ) ;
#53210=ORIENTED_EDGE ( 'NONE', *, *, #9786, .F. ) ;
#53230=VECTOR ( 'NONE', #94298, 1000.000000000000000 ) ;
#53231=STYLED_ITEM ( 'NONE', ( #126896 ), #63692 ) ;
#53244=CARTESIAN_POINT ( 'NONE',  ( 3.657803576507369314, 12.22753933337904009, -27.06132802995527697 ) ) ;
#53273=EDGE_LOOP ( 'NONE', ( #114796, #64433, #96710, #118732 ) ) ;
#53307=( LENGTH_UNIT ( ) NAMED_UNIT ( * ) SI_UNIT ( .MILLI., .METRE. ) );
#53373=CYLINDRICAL_SURFACE ( 'NONE', #30490, 3.000000000000002665 ) ;
#53374=( BOUNDED_CURVE ( )  B_SPLINE_CURVE ( 3, ( #33977, #66604, #11461, #65191 ),
 .UNSPECIFIED., .F., .F. ) 
 B_SPLINE_CURVE_WITH_KNOTS ( ( 4, 4 ),
 ( 1.570796326794896558, 3.141592653589793560 ),
 .UNSPECIFIED. ) 
 CURVE ( )  GEOMETRIC_REPRESENTATION_ITEM ( )  RATIONAL_B_SPLINE_CURVE ( ( 1.000000000000000000, 0.8047378541243649375, 0.8047378541243649375, 1.000000000000000000 ) ) 
 REPRESENTATION_ITEM ( '' )  );
#53394=VERTEX_POINT ( 'NONE', #120547 ) ;
#53414=CARTESIAN_POINT ( 'NONE',  ( 0.000000000000000000, -4.870000000000014317, -10.00000000000000178 ) ) ;
#53428=DIRECTION ( 'NONE',  ( 0.000000000000000000, -1.000000000000000000, 0.000000000000000000 ) ) ;
#53452=STYLED_ITEM ( 'NONE', ( #142872 ), #142559 ) ;
#53488=AXIS2_PLACEMENT_3D ( 'NONE', #42589, #22905, #120815 ) ;
#53528=SURFACE_STYLE_FILL_AREA ( #119459 ) ;
#53547=ORIENTED_EDGE ( 'NONE', *, *, #73138, .T. ) ;
#53670=CIRCLE ( 'NONE', #9648, 1.898649999999993065 ) ;
#53676=VECTOR ( 'NONE', #1899, 1000.000000000000000 ) ;
#53724=CARTESIAN_POINT ( 'NONE',  ( 3.716138108416388253, 12.21541996048661183, -27.07211710725142950 ) ) ;
#53743=FACE_OUTER_BOUND ( 'NONE', #19578, .T. ) ;
#53782=COLOUR_RGB ( '', 0.08235294, 0.09019608, 0.10196078) ;
#53816=CIRCLE ( 'NONE', #118565, 0.5000000000000004441 ) ;
#53826=VECTOR ( 'NONE', #112448, 1000.000000000000000 ) ;
#53862=ORIENTED_EDGE ( 'NONE', *, *, #107279, .F. ) ;
#53929=AXIS2_PLACEMENT_3D ( 'NONE', #115721, #36089, #93301 ) ;
#53946=( NAMED_UNIT ( * ) SI_UNIT ( $, .STERADIAN. ) SOLID_ANGLE_UNIT ( ) );
#53953=CIRCLE ( 'NONE', #9924, 0.5000000000000004441 ) ;
#53975=ORIENTED_EDGE ( 'NONE', *, *, #88898, .F. ) ;
#54000=CARTESIAN_POINT ( 'NONE',  ( 7.139999999999956160, -60.26999999999998892, -8.278119684037271497 ) ) ;
#54008=CIRCLE ( 'NONE', #135049, 3.000000000000000000 ) ;
#54010=CARTESIAN_POINT ( 'NONE',  ( -7.412718841549110316, 12.49264501416213946, -25.30319893193128777 ) ) ;
#54014=SURFACE_STYLE_USAGE ( .BOTH. , #31522 ) ;
#54055=FILL_AREA_STYLE ('',( #128716 ) ) ;
#54214=ORIENTED_EDGE ( 'NONE', *, *, #44765, .F. ) ;
#54233=LINE ( 'NONE', #101262, #53676 ) ;
#54286=PRESENTATION_STYLE_ASSIGNMENT (( #133260 ) ) ;
#54293=EDGE_LOOP ( 'NONE', ( #23538, #126315, #2273, #31935 ) ) ;
#54296=EDGE_LOOP ( 'NONE', ( #58951, #74508, #7648, #71304, #74729, #65160, #70960 ) ) ;
#54299=VECTOR ( 'NONE', #45788, 1000.000000000000000 ) ;
#54318=ADVANCED_FACE ( 'NONE', ( #35946 ), #101160, .T. ) ;
#54381=PRESENTATION_STYLE_ASSIGNMENT (( #97088 ) ) ;
#54393=ORIENTED_EDGE ( 'NONE', *, *, #59446, .F. ) ;
#54414=LINE ( 'NONE', #20301, #11827 ) ;
#54416=CIRCLE ( 'NONE', #66007, 0.5000000000000004441 ) ;
#54443=DIRECTION ( 'NONE',  ( -0.000000000000000000, -0.000000000000000000, -1.000000000000000000 ) ) ;
#54448=CARTESIAN_POINT ( 'NONE',  ( 14.93213401340503310, 4.189643424786883230, -32.27832594409215261 ) ) ;
#54507=ORIENTED_EDGE ( 'NONE', *, *, #37672, .F. ) ;
#54527=EDGE_CURVE ( 'NONE', #27902, #40406, #39852, .T. ) ;
#54562=CARTESIAN_POINT ( 'NONE',  ( -19.66071175273273752, -1.129697928112111116, -31.75000930624208451 ) ) ;
#54581=SURFACE_SIDE_STYLE ('',( #86493 ) ) ;
#54594=DIRECTION ( 'NONE',  ( 0.000000000000000000, 0.000000000000000000, -1.000000000000000000 ) ) ;
#54623=DIRECTION ( 'NONE',  ( -1.000000000000000000, 0.000000000000000000, 0.000000000000000000 ) ) ;
#54671=DIRECTION ( 'NONE',  ( 3.469446951953611033E-15, 0.000000000000000000, 1.000000000000000000 ) ) ;
#54694=DIRECTION ( 'NONE',  ( 0.000000000000000000, -0.000000000000000000, -1.000000000000000000 ) ) ;
#54703=EDGE_CURVE ( 'NONE', #72776, #97358, #73119, .T. ) ;
#54704=ORIENTED_EDGE ( 'NONE', *, *, #33903, .T. ) ;
#54710=CARTESIAN_POINT ( 'NONE',  ( 9.971754739210105356, 9.503873597802957818, -27.24537889701776905 ) ) ;
#54746=CARTESIAN_POINT ( 'NONE',  ( 16.45742106731621135, 0.9613713492673626737, -33.49048331797055766 ) ) ;
#54758=CARTESIAN_POINT ( 'NONE',  ( -12.20000000000000817, -1.670812611072399357E-15, 0.000000000000000000 ) ) ;
#54777=( NAMED_UNIT ( * ) PLANE_ANGLE_UNIT ( ) SI_UNIT ( $, .RADIAN. ) );
#54778=UNCERTAINTY_MEASURE_WITH_UNIT (LENGTH_MEASURE( 1.000000000000000082E-05 ), #16091, 'distance_accuracy_value', 'NONE');
#54826=FILL_AREA_STYLE_COLOUR ( '', #113784 ) ;
#54868=VERTEX_POINT ( 'NONE', #140072 ) ;
#54934=EDGE_CURVE ( 'NONE', #81122, #99547, #81556, .T. ) ;
#54979=EDGE_CURVE ( 'NONE', #118785, #60140, #53016, .T. ) ;
#55036=CARTESIAN_POINT ( 'NONE',  ( 19.39745846707657151, 0.5627691706057111887, -30.75765991350439421 ) ) ;
#55041=VERTEX_POINT ( 'NONE', #102276 ) ;
#55063=DIRECTION ( 'NONE',  ( -0.000000000000000000, -1.000000000000000000, -0.000000000000000000 ) ) ;
#55115=EDGE_CURVE ( 'NONE', #113156, #100573, #118556, .T. ) ;
#55134=AXIS2_PLACEMENT_3D ( 'NONE', #15600, #50435, #127255 ) ;
#55137=CIRCLE ( 'NONE', #122255, 0.5000000000000005551 ) ;
#55196=DIRECTION ( 'NONE',  ( 1.000000000000000000, 3.115803279706882722E-16, 0.000000000000000000 ) ) ;
#55218=DIRECTION ( 'NONE',  ( 0.000000000000000000, 0.000000000000000000, 1.000000000000000000 ) ) ;
#55233=DIRECTION ( 'NONE',  ( 0.000000000000000000, 0.000000000000000000, -1.000000000000000000 ) ) ;
#55247=( BOUNDED_CURVE ( )  B_SPLINE_CURVE ( 3, ( #104065, #125126, #70783, #34567 ),
 .UNSPECIFIED., .F., .T. ) 
 B_SPLINE_CURVE_WITH_KNOTS ( ( 4, 4 ),
 ( 1.570796326794896558, 3.141592653589793116 ),
 .UNSPECIFIED. ) 
 CURVE ( )  GEOMETRIC_REPRESENTATION_ITEM ( )  RATIONAL_B_SPLINE_CURVE ( ( 1.000000000000000000, 0.8047378541243649375, 0.8047378541243649375, 1.000000000000000000 ) ) 
 REPRESENTATION_ITEM ( '' )  );
#55269=COLOUR_RGB ( '', 0.40784314, 0.44705882, 0.49803922) ;
#55275=CARTESIAN_POINT ( 'NONE',  ( 13.74720049256562682, 8.866765337654086920, -27.55742918605191960 ) ) ;
#55292=FILL_AREA_STYLE ('',( #132868 ) ) ;
#55317=ADVANCED_FACE ( 'NONE', ( #73905 ), #111336, .F. ) ;
#55323=ORIENTED_EDGE ( 'NONE', *, *, #29080, .T. ) ;
#55348=DIRECTION ( 'NONE',  ( 0.000000000000000000, 0.000000000000000000, -1.000000000000000000 ) ) ;
#55352=CARTESIAN_POINT ( 'NONE',  ( -8.773457579940252170E-14, -35.14999999999997726, -39.50000000000000000 ) ) ;
#55430=DIRECTION ( 'NONE',  ( 0.000000000000000000, 0.000000000000000000, -1.000000000000000000 ) ) ;
#55437=AXIS2_PLACEMENT_3D ( 'NONE', #81573, #3248, #125778 ) ;
#55439=DIRECTION ( 'NONE',  ( 0.000000000000000000, 0.000000000000000000, -1.000000000000000000 ) ) ;
#55461=AXIS2_PLACEMENT_3D ( 'NONE', #130357, #19433, #18695 ) ;
#55485=LINE ( 'NONE', #69214, #128699 ) ;
#55565=DIRECTION ( 'NONE',  ( 0.000000000000000000, -1.000000000000000000, 0.000000000000000000 ) ) ;
#55575=DIRECTION ( 'NONE',  ( 6.694238229904089514E-15, -0.9647414015272165466, 0.2631995976047492580 ) ) ;
#55593=( GEOMETRIC_REPRESENTATION_CONTEXT ( 3 ) GLOBAL_UNCERTAINTY_ASSIGNED_CONTEXT ( ( #84021 ) ) GLOBAL_UNIT_ASSIGNED_CONTEXT ( ( #127952, #62696, #106878 ) ) REPRESENTATION_CONTEXT ( 'NONE', 'WORKASPACE' ) );
#55689=SURFACE_SIDE_STYLE ('',( #23002 ) ) ;
#55720=EDGE_LOOP ( 'NONE', ( #69471, #136992, #31825, #75350, #28730, #140338, #26167 ) ) ;
#55753=EDGE_CURVE ( 'NONE', #38181, #23998, #14238, .T. ) ;
#55798=FILL_AREA_STYLE ('',( #142782 ) ) ;
#55812=CARTESIAN_POINT ( 'NONE',  ( 16.96306865584292467, -0.7331570413090292559, -35.15540272813352374 ) ) ;
#55819=DIRECTION ( 'NONE',  ( -0.000000000000000000, -0.000000000000000000, -1.000000000000000000 ) ) ;
#55836=CARTESIAN_POINT ( 'NONE',  ( 7.939999999999994174, -35.56014942880460694, -10.00000000000000178 ) ) ;
#55853=VECTOR ( 'NONE', #60777, 1000.000000000000000 ) ;
#55861=MECHANICAL_DESIGN_GEOMETRIC_PRESENTATION_REPRESENTATION('',(#92867),#32774);
#55862=CIRCLE ( 'NONE', #21050, 0.5000000000000004441 ) ;
#55875=LINE ( 'NONE', #122515, #61492 ) ;
#55956=SURFACE_STYLE_FILL_AREA ( #11669 ) ;
#55964=STYLED_ITEM ( 'NONE', ( #30189 ), #143366 ) ;
#55971=CARTESIAN_POINT ( 'NONE',  ( -7.140000000000001457, 0.000000000000000000, -40.00000000000000000 ) ) ;
#55975=( GEOMETRIC_REPRESENTATION_CONTEXT ( 3 ) GLOBAL_UNCERTAINTY_ASSIGNED_CONTEXT ( ( #112840 ) ) GLOBAL_UNIT_ASSIGNED_CONTEXT ( ( #37146, #14683, #58964 ) ) REPRESENTATION_CONTEXT ( 'NONE', 'WORKASPACE' ) );
#55997=AXIS2_PLACEMENT_3D ( 'NONE', #107584, #86575, #31471 ) ;
#55999=MECHANICAL_DESIGN_GEOMETRIC_PRESENTATION_REPRESENTATION('',(#90660),#28132);
#56022=CARTESIAN_POINT ( 'NONE',  ( 7.939999999999994174, -39.93000000000000682, -10.00000000000000178 ) ) ;
#56042=CARTESIAN_POINT ( 'NONE',  ( 0.000000000000000000, -34.64999999999999147, 17.99210858042621908 ) ) ;
#56071=AXIS2_PLACEMENT_3D ( 'NONE', #95112, #48784, #61133 ) ;
#56105=CARTESIAN_POINT ( 'NONE',  ( 31.92500000000000782, 22.27000000000000313, -14.71147562388301822 ) ) ;
#56136=CIRCLE ( 'NONE', #32950, 2.247899999999996901 ) ;
#56164=CARTESIAN_POINT ( 'NONE',  ( 18.50044947910937765, 3.007166298682988348, -30.07082962428489381 ) ) ;
#56180=DIRECTION ( 'NONE',  ( -0.000000000000000000, -1.000000000000000000, -0.000000000000000000 ) ) ;
#56198=LINE ( 'NONE', #1027, #50587 ) ;
#56233=EDGE_CURVE ( 'NONE', #106369, #46696, #102020, .T. ) ;
#56237=UNCERTAINTY_MEASURE_WITH_UNIT (LENGTH_MEASURE( 1.000000000000000082E-05 ), #14893, 'distance_accuracy_value', 'NONE');
#56252=EDGE_CURVE ( 'NONE', #143240, #108517, #60345, .T. ) ;
#56270=CARTESIAN_POINT ( 'NONE',  ( -7.940000000000007496, -60.26999999999998892, -7.752100000000002211 ) ) ;
#56286=CARTESIAN_POINT ( 'NONE',  ( -19.93618819985229251, -3.270000000000008900, -35.71710890046286124 ) ) ;
#56295=ORIENTED_EDGE ( 'NONE', *, *, #18226, .T. ) ;
#56309=DIRECTION ( 'NONE',  ( -1.000000000000000000, 2.496005001405478586E-15, 0.000000000000000000 ) ) ;
#56331=ORIENTED_EDGE ( 'NONE', *, *, #57517, .F. ) ;
#56336=ORIENTED_EDGE ( 'NONE', *, *, #110869, .T. ) ;
#56343=SURFACE_STYLE_FILL_AREA ( #133163 ) ;
#56346=ORIENTED_EDGE ( 'NONE', *, *, #45168, .T. ) ;
#56391=CARTESIAN_POINT ( 'NONE',  ( 19.91020365697643513, -3.046927250066239434, -34.73593278446270460 ) ) ;
#56412=CARTESIAN_POINT ( 'NONE',  ( -12.19999999999999929, -59.76999999999998892, -40.00000000000000000 ) ) ;
#56441=DIRECTION ( 'NONE',  ( 1.000000000000000000, 1.369518533665900312E-16, -0.000000000000000000 ) ) ;
#56446=CARTESIAN_POINT ( 'NONE',  ( -16.50229999999999819, 3.130000000000007887, -22.35000000000000142 ) ) ;
#56487=ADVANCED_FACE ( 'NONE', ( #72556 ), #50752, .T. ) ;
#56521=SURFACE_SIDE_STYLE ('',( #134778 ) ) ;
#56533=CIRCLE ( 'NONE', #75037, 3.000000000000002665 ) ;
#56577=VERTEX_POINT ( 'NONE', #18816 ) ;
#56583=VECTOR ( 'NONE', #140794, 1000.000000000000000 ) ;
#56651=ADVANCED_FACE ( 'NONE', ( #52169 ), #131162, .T. ) ;
#56690=FILL_AREA_STYLE_COLOUR ( '', #68788 ) ;
#56746=FACE_OUTER_BOUND ( 'NONE', #35549, .T. ) ;
#56824=DIRECTION ( 'NONE',  ( -1.000000000000000000, -1.369518533665899572E-16, 0.000000000000000000 ) ) ;
#56860=( LENGTH_UNIT ( ) NAMED_UNIT ( * ) SI_UNIT ( .MILLI., .METRE. ) );
#56871=VERTEX_POINT ( 'NONE', #49738 ) ;
#56878=CARTESIAN_POINT ( 'NONE',  ( 16.63593005512386824, 5.882511235426649776, -28.99105463435266472 ) ) ;
#56889=PRESENTATION_STYLE_ASSIGNMENT (( #113347 ) ) ;
#56921=FILL_AREA_STYLE ('',( #115503 ) ) ;
#56935=EDGE_CURVE ( 'NONE', #81524, #19482, #94768, .T. ) ;
#56949=ORIENTED_EDGE ( 'NONE', *, *, #56233, .T. ) ;
#56950=LINE ( 'NONE', #93822, #88447 ) ;
#56951=EDGE_CURVE ( 'NONE', #79346, #63984, #50433, .T. ) ;
#56982=DIRECTION ( 'NONE',  ( 0.000000000000000000, 0.000000000000000000, 1.000000000000000000 ) ) ;
#57005=( GEOMETRIC_REPRESENTATION_CONTEXT ( 3 ) GLOBAL_UNCERTAINTY_ASSIGNED_CONTEXT ( ( #131616 ) ) GLOBAL_UNIT_ASSIGNED_CONTEXT ( ( #85109, #130056, #53946 ) ) REPRESENTATION_CONTEXT ( 'NONE', 'WORKASPACE' ) );
#57085=( LENGTH_UNIT ( ) NAMED_UNIT ( * ) SI_UNIT ( .MILLI., .METRE. ) );
#57217=EDGE_CURVE ( 'NONE', #70779, #137008, #2139, .T. ) ;
#57221=EDGE_LOOP ( 'NONE', ( #95398, #130154, #1094, #17392 ) ) ;
#57222=LINE ( 'NONE', #46356, #10121 ) ;
#57223=ORIENTED_EDGE ( 'NONE', *, *, #30376, .T. ) ;
#57245=ORIENTED_EDGE ( 'NONE', *, *, #104797, .T. ) ;
#57255=SURFACE_STYLE_FILL_AREA ( #12978 ) ;
#57276=EDGE_CURVE ( 'NONE', #135430, #15191, #13741, .T. ) ;
#57281=DIRECTION ( 'NONE',  ( -2.496005001405472275E-15, -1.000000000000000000, 0.000000000000000000 ) ) ;
#57349=CARTESIAN_POINT ( 'NONE',  ( -19.05499999999999261, 3.130000000000007887, -22.35000000000000142 ) ) ;
#57371=DIRECTION ( 'NONE',  ( 0.000000000000000000, -1.000000000000000000, 0.000000000000000000 ) ) ;
#57400=AXIS2_PLACEMENT_3D ( 'NONE', #106895, #130834, #74297 ) ;
#57410=CARTESIAN_POINT ( 'NONE',  ( 17.01299345043647193, -0.9444868035624204294, -36.39086428169088094 ) ) ;
#57428=CARTESIAN_POINT ( 'NONE',  ( 16.83830262477991369, 5.618291726703525057, -29.10193646598569472 ) ) ;
#57436=( LENGTH_UNIT ( ) NAMED_UNIT ( * ) SI_UNIT ( .MILLI., .METRE. ) );
#57443=CARTESIAN_POINT ( 'NONE',  ( 19.93618820137057668, -0.2699999999999959099, -36.39086428169088094 ) ) ;
#57508=STYLED_ITEM ( 'NONE', ( #87131 ), #93708 ) ;
#57517=EDGE_CURVE ( 'NONE', #61882, #50410, #17617, .T. ) ;
#57553=FILL_AREA_STYLE ('',( #13996 ) ) ;
#57557=EDGE_LOOP ( 'NONE', ( #78742, #37459, #16869, #74513 ) ) ;
#57585=MECHANICAL_DESIGN_GEOMETRIC_PRESENTATION_REPRESENTATION('',(#115366),#83020);
#57587=EDGE_CURVE ( 'NONE', #40891, #128588, #118365, .T. ) ;
#57611=DIRECTION ( 'NONE',  ( 1.000000000000000000, 3.115803279706882722E-16, -0.000000000000000000 ) ) ;
#57613=ADVANCED_FACE ( 'NONE', ( #87181 ), #64719, .T. ) ;
#57641=UNCERTAINTY_MEASURE_WITH_UNIT (LENGTH_MEASURE( 1.000000000000000082E-05 ), #49956, 'distance_accuracy_value', 'NONE');
#57649=ORIENTED_EDGE ( 'NONE', *, *, #14161, .T. ) ;
#57681=MECHANICAL_DESIGN_GEOMETRIC_PRESENTATION_REPRESENTATION('',(#103870),#41395);
#57696=CARTESIAN_POINT ( 'NONE',  ( -19.65190707646159751, -1.080577986147907454, -31.74483932211373372 ) ) ;
#57720=FILL_AREA_STYLE ('',( #68595 ) ) ;
#57788=AXIS2_PLACEMENT_3D ( 'NONE', #99195, #129698, #132610 ) ;
#57799=CARTESIAN_POINT ( 'NONE',  ( 19.65184941750880299, -1.080186769994980533, -31.74454988527380905 ) ) ;
#57981=VERTEX_POINT ( 'NONE', #117287 ) ;
#58061=VERTEX_POINT ( 'NONE', #133908 ) ;
#58105=( LENGTH_UNIT ( ) NAMED_UNIT ( * ) SI_UNIT ( .MILLI., .METRE. ) );
#58127=CARTESIAN_POINT ( 'NONE',  ( 34.92500000000001847, -6.269999999999991580, -40.00000000000000000 ) ) ;
#58142=ORIENTED_EDGE ( 'NONE', *, *, #10429, .F. ) ;
#58156=VERTEX_POINT ( 'NONE', #93961 ) ;
#58166=ORIENTED_EDGE ( 'NONE', *, *, #82792, .T. ) ;
#58173=DIRECTION ( 'NONE',  ( 3.115803279706882722E-16, -1.000000000000000000, -1.016133275908817741E-16 ) ) ;
#58264=CARTESIAN_POINT ( 'NONE',  ( 34.25389700712507590, 22.27000000000000668, -12.46204991634331094 ) ) ;
#58361=LINE ( 'NONE', #127864, #116377 ) ;
#58367=VECTOR ( 'NONE', #111374, 1000.000000000000000 ) ;
#58399=( GEOMETRIC_REPRESENTATION_CONTEXT ( 3 ) GLOBAL_UNCERTAINTY_ASSIGNED_CONTEXT ( ( #96953 ) ) GLOBAL_UNIT_ASSIGNED_CONTEXT ( ( #67876, #36616, #91037 ) ) REPRESENTATION_CONTEXT ( 'NONE', 'WORKASPACE' ) );
#58434=CARTESIAN_POINT ( 'NONE',  ( -16.84500517045543333, -0.1638869648888886532, -31.04645391278758026 ) ) ;
#58463=VECTOR ( 'NONE', #81222, 1000.000000000000000 ) ;
#58464=LINE ( 'NONE', #12028, #142765 ) ;
#58468=MECHANICAL_DESIGN_GEOMETRIC_PRESENTATION_REPRESENTATION('',(#35368),#130249);
#58472=SURFACE_STYLE_FILL_AREA ( #57720 ) ;
#58615=STYLED_ITEM ( 'NONE', ( #42441 ), #86209 ) ;
#58667=EDGE_CURVE ( 'NONE', #98685, #128930, #47493, .T. ) ;
#58682=ORIENTED_EDGE ( 'NONE', *, *, #7843, .F. ) ;
#58694=VECTOR ( 'NONE', #103744, 1000.000000000000000 ) ;
#58768=ADVANCED_FACE ( 'NONE', ( #114121 ), #123609, .F. ) ;
#58778=DIRECTION ( 'NONE',  ( -1.000000000000000000, 1.248002500702738701E-15, 0.000000000000000000 ) ) ;
#58816=VECTOR ( 'NONE', #126384, 1000.000000000000000 ) ;
#58852=ORIENTED_EDGE ( 'NONE', *, *, #135866, .F. ) ;
#58854=EDGE_CURVE ( 'NONE', #57981, #118892, #4472, .T. ) ;
#58884=SURFACE_SIDE_STYLE ('',( #94291 ) ) ;
#58892=ADVANCED_FACE ( 'NONE', ( #99479 ), #87206, .T. ) ;
#58902=CARTESIAN_POINT ( 'NONE',  ( 12.69999999999999574, -35.05528132343076209, 17.90627459364451113 ) ) ;
#58922=FACE_OUTER_BOUND ( 'NONE', #74863, .T. ) ;
#58931=FACE_OUTER_BOUND ( 'NONE', #77704, .T. ) ;
#58951=ORIENTED_EDGE ( 'NONE', *, *, #100950, .T. ) ;
#58963=LINE ( 'NONE', #3756, #126333 ) ;
#58964=( NAMED_UNIT ( * ) SI_UNIT ( $, .STERADIAN. ) SOLID_ANGLE_UNIT ( ) );
#58981=CARTESIAN_POINT ( 'NONE',  ( 33.81525066741142638, 22.26999999999999957, -13.39192763381150719 ) ) ;
#58986=SURFACE_STYLE_FILL_AREA ( #14708 ) ;
#58989=SURFACE_STYLE_USAGE ( .BOTH. , #69849 ) ;
#59043=SURFACE_STYLE_FILL_AREA ( #125692 ) ;
#59055=ADVANCED_FACE ( 'NONE', ( #58922 ), #35725, .T. ) ;
#59140=SURFACE_STYLE_USAGE ( .BOTH. , #3941 ) ;
#59183=CARTESIAN_POINT ( 'NONE',  ( -8.378674182341532273, 12.11998467473676833, -25.56646076112756916 ) ) ;
#59197=CARTESIAN_POINT ( 'NONE',  ( -7.940000000000001279, -33.26999999999999602, -10.00000000000000178 ) ) ;
#59220=CARTESIAN_POINT ( 'NONE',  ( -34.92499999999997584, 22.27000000000000668, -7.752744394707050901 ) ) ;
#59239=CARTESIAN_POINT ( 'NONE',  ( 17.29169637474938526, -1.887777690644416140, -32.52073842440807283 ) ) ;
#59248=ORIENTED_EDGE ( 'NONE', *, *, #53095, .T. ) ;
#59321=VECTOR ( 'NONE', #72851, 1000.000000000000000 ) ;
#59353=FACE_BOUND ( 'NONE', #10647, .T. ) ;
#59357=ORIENTED_EDGE ( 'NONE', *, *, #118976, .F. ) ;
#59363=CARTESIAN_POINT ( 'NONE',  ( -7.140000000000001457, -35.14999999999999147, -40.00000000000000000 ) ) ;
#59442=EDGE_CURVE ( 'NONE', #25054, #129819, #129641, .T. ) ;
#59446=EDGE_CURVE ( 'NONE', #84209, #89560, #70335, .T. ) ;
#59510=CARTESIAN_POINT ( 'NONE',  ( 12.19999999999999574, 0.000000000000000000, -39.50000000000000000 ) ) ;
#59608=ORIENTED_EDGE ( 'NONE', *, *, #73471, .F. ) ;
#59646=CARTESIAN_POINT ( 'NONE',  ( -34.42499999999997584, 0.000000000000000000, 0.000000000000000000 ) ) ;
#59667=DIRECTION ( 'NONE',  ( -0.000000000000000000, 1.000000000000000000, -0.000000000000000000 ) ) ;
#59670=CARTESIAN_POINT ( 'NONE',  ( 9.524999999999991473, -4.870000000000013429, -10.00000000000000178 ) ) ;
#59684=FILL_AREA_STYLE ('',( #3124 ) ) ;
#59720=EDGE_LOOP ( 'NONE', ( #138054, #100681, #134379, #102987 ) ) ;
#59728=( LENGTH_UNIT ( ) NAMED_UNIT ( * ) SI_UNIT ( .MILLI., .METRE. ) );
#59738=LINE ( 'NONE', #60460, #44943 ) ;
#59778=VERTEX_POINT ( 'NONE', #114952 ) ;
#59865=CARTESIAN_POINT ( 'NONE',  ( -15.78892356518500328, 2.636128110293266769, -32.92760517736494563 ) ) ;
#59873=CYLINDRICAL_SURFACE ( 'NONE', #128107, 0.5000000000000005551 ) ;
#59938=VERTEX_POINT ( 'NONE', #119262 ) ;
#59982=FACE_OUTER_BOUND ( 'NONE', #51278, .T. ) ;
#60028=VECTOR ( 'NONE', #24263, 1000.000000000000000 ) ;
#60063=LINE ( 'NONE', #59363, #137429 ) ;
#60140=VERTEX_POINT ( 'NONE', #126404 ) ;
#60227=EDGE_CURVE ( 'NONE', #71803, #42501, #31986, .T. ) ;
#60230=DIRECTION ( 'NONE',  ( 0.000000000000000000, 0.000000000000000000, 1.000000000000000000 ) ) ;
#60265=FILL_AREA_STYLE ('',( #16728 ) ) ;
#60284=CARTESIAN_POINT ( 'NONE',  ( -14.50845100080809225, 8.197497501871428227, -27.90950007455948523 ) ) ;
#60316=CIRCLE ( 'NONE', #16265, 0.5000000000000004441 ) ;
#60345=CIRCLE ( 'NONE', #9347, 2.552699999999997971 ) ;
#60391=DIRECTION ( 'NONE',  ( 0.3240768213499726214, 0.9146165434626271074, 0.2417659866237898969 ) ) ;
#60403=CARTESIAN_POINT ( 'NONE',  ( -34.92499999999999005, 2.729999999999986215, -36.39086428169088094 ) ) ;
#60427=CARTESIAN_POINT ( 'NONE',  ( -7.940000000000007496, -35.56014942880460694, -10.00000000000000178 ) ) ;
#60460=CARTESIAN_POINT ( 'NONE',  ( -12.69999999999999929, -59.76999999999998892, -40.00000000000000000 ) ) ;
#60479=CARTESIAN_POINT ( 'NONE',  ( 12.69999999999999574, -22.33999999999998565, -0.5000000000000000000 ) ) ;
#60499=VECTOR ( 'NONE', #109507, 1000.000000000000000 ) ;
#60515=DIRECTION ( 'NONE',  ( -1.369518533665900312E-16, 1.000000000000000000, -0.000000000000000000 ) ) ;
#60541=ORIENTED_EDGE ( 'NONE', *, *, #3341, .T. ) ;
#60543=EDGE_LOOP ( 'NONE', ( #109149, #8998, #120935 ) ) ;
#60554=( LENGTH_UNIT ( ) NAMED_UNIT ( * ) SI_UNIT ( .MILLI., .METRE. ) );
#60568=FACE_OUTER_BOUND ( 'NONE', #21315, .T. ) ;
#60569=APPLICATION_CONTEXT ( 'automotive_design' ) ;
#60577=ORIENTED_EDGE ( 'NONE', *, *, #49012, .F. ) ;
#60595=EDGE_CURVE ( 'NONE', #50924, #79752, #3025, .T. ) ;
#60598=AXIS2_PLACEMENT_3D ( 'NONE', #6522, #20290, #52224 ) ;
#60611=CARTESIAN_POINT ( 'NONE',  ( -9.486600348837527008, 9.794720693715408544, -29.02262996827379737 ) ) ;
#60631=EDGE_CURVE ( 'NONE', #237, #64363, #109038, .T. ) ;
#60638=STYLED_ITEM ( 'NONE', ( #69271 ), #143376 ) ;
#60659=UNCERTAINTY_MEASURE_WITH_UNIT (LENGTH_MEASURE( 1.000000000000000082E-05 ), #123568, 'distance_accuracy_value', 'NONE');
#60694=CARTESIAN_POINT ( 'NONE',  ( 12.69999999999999574, -35.13237070076361590, 17.62370837922860645 ) ) ;
#60777=DIRECTION ( 'NONE',  ( -0.000000000000000000, -1.000000000000000000, -0.000000000000000000 ) ) ;
#60862=CARTESIAN_POINT ( 'NONE',  ( 7.939999999999994174, -60.26999999999998892, -10.00000000000000178 ) ) ;
#60874=FILL_AREA_STYLE_COLOUR ( '', #120694 ) ;
#60888=CARTESIAN_POINT ( 'NONE',  ( -12.20000000000000284, -34.64999999999999147, 17.49210858042621908 ) ) ;
#60919=ORIENTED_EDGE ( 'NONE', *, *, #14087, .F. ) ;
#60973=FILL_AREA_STYLE_COLOUR ( '', #120002 ) ;
#60986=LINE ( 'NONE', #28319, #125418 ) ;
#61003=ORIENTED_EDGE ( 'NONE', *, *, #95216, .T. ) ;
#61007=AXIS2_PLACEMENT_3D ( 'NONE', #106082, #138765, #116282 ) ;
#61020=CARTESIAN_POINT ( 'NONE',  ( -16.45742106731621845, 0.9613713492673547911, -33.49048331797055766 ) ) ;
#61028=CARTESIAN_POINT ( 'NONE',  ( -16.86802775199585014, 5.611381925338908339, -29.11273303788685141 ) ) ;
#61045=CARTESIAN_POINT ( 'NONE',  ( 19.93618820137057668, -0.2700000000508058218, -36.99999999997771738 ) ) ;
#61100=DIRECTION ( 'NONE',  ( 0.000000000000000000, 0.000000000000000000, 1.000000000000000000 ) ) ;
#61133=DIRECTION ( 'NONE',  ( 3.115803279706882722E-16, -1.000000000000000000, 0.000000000000000000 ) ) ;
#61135=CIRCLE ( 'NONE', #5154, 0.5000000000000004441 ) ;
#61169=VECTOR ( 'NONE', #108300, 1000.000000000000000 ) ;
#61201=ORIENTED_EDGE ( 'NONE', *, *, #24635, .F. ) ;
#61237=CARTESIAN_POINT ( 'NONE',  ( 0.000000000000000000, -60.26999999999998892, -40.00000000000000000 ) ) ;
#61281=DIRECTION ( 'NONE',  ( 1.000000000000000000, 0.000000000000000000, 0.000000000000000000 ) ) ;
#61287=CARTESIAN_POINT ( 'NONE',  ( -19.28515664589289003, 1.196650378695324646, -30.59010235425024149 ) ) ;
#61303=PRODUCT_CONTEXT ( 'NONE', #60569, 'mechanical' ) ;
#61334=CARTESIAN_POINT ( 'NONE',  ( -8.807277435403058519, 10.22259551701957214, -26.82144004025722950 ) ) ;
#61357=CARTESIAN_POINT ( 'NONE',  ( -7.134088674951100550, -39.92999999999999261, 19.02448003456068548 ) ) ;
#61375=EDGE_LOOP ( 'NONE', ( #105357, #10820, #47071, #69694 ) ) ;
#61378=DIRECTION ( 'NONE',  ( 0.000000000000000000, 0.000000000000000000, -1.000000000000000000 ) ) ;
#61478=SPHERICAL_SURFACE ( 'NONE', #115604, 0.5000000000000000000 ) ;
#61482=DIRECTION ( 'NONE',  ( 0.000000000000000000, 0.000000000000000000, 1.000000000000000000 ) ) ;
#61492=VECTOR ( 'NONE', #81186, 1000.000000000000000 ) ;
#61576=DIRECTION ( 'NONE',  ( 0.000000000000000000, 0.000000000000000000, 1.000000000000000000 ) ) ;
#61600=CARTESIAN_POINT ( 'NONE',  ( 0.000000000000000000, -21.76999999999999247, 0.000000000000000000 ) ) ;
#61603=VERTEX_POINT ( 'NONE', #13917 ) ;
#61619=LINE ( 'NONE', #104352, #109315 ) ;
#61634=ORIENTED_EDGE ( 'NONE', *, *, #1970, .T. ) ;
#61641=DIRECTION ( 'NONE',  ( -0.000000000000000000, -1.000000000000000000, -0.000000000000000000 ) ) ;
#61654=CARTESIAN_POINT ( 'NONE',  ( 7.139999999999984581, -39.92999999999998550, -39.79289321881344677 ) ) ;
#61748=CARTESIAN_POINT ( 'NONE',  ( -7.213366709350353290, 11.05501350725457499, -28.05856295898191632 ) ) ;
#61749=SURFACE_STYLE_USAGE ( .BOTH. , #18926 ) ;
#61759=ORIENTED_EDGE ( 'NONE', *, *, #133838, .F. ) ;
#61796=ORIENTED_EDGE ( 'NONE', *, *, #46901, .T. ) ;
#61802=PRODUCT_DEFINITION_CONTEXT ( 'detailed design', #72652, 'design' ) ;
#61810=( LENGTH_UNIT ( ) NAMED_UNIT ( * ) SI_UNIT ( .MILLI., .METRE. ) );
#61841=VERTEX_POINT ( 'NONE', #48725 ) ;
#61881=EDGE_CURVE ( 'NONE', #17782, #89560, #47701, .T. ) ;
#61882=VERTEX_POINT ( 'NONE', #76188 ) ;
#61901=CARTESIAN_POINT ( 'NONE',  ( -7.140000000000001457, -39.92999999999999261, -39.50000000000000000 ) ) ;
#61905=VERTEX_POINT ( 'NONE', #108054 ) ;
#61925=EDGE_CURVE ( 'NONE', #113156, #68517, #53816, .T. ) ;
#61959=DIRECTION ( 'NONE',  ( 0.000000000000000000, -0.000000000000000000, -1.000000000000000000 ) ) ;
#62023=CARTESIAN_POINT ( 'NONE',  ( -9.209127552564122965, 9.981455117011716283, -26.96467221759983346 ) ) ;
#62031=EDGE_LOOP ( 'NONE', ( #142196, #105894, #110656, #120132, #65207, #62475, #129396, #40061 ) ) ;
#62034=DIRECTION ( 'NONE',  ( 0.000000000000000000, -1.000000000000000000, 0.000000000000000000 ) ) ;
#62060=CARTESIAN_POINT ( 'NONE',  ( -34.25456027042017837, 22.27000000000000668, -12.45996461598220506 ) ) ;
#62074=LINE ( 'NONE', #51186, #44179 ) ;
#62076=CARTESIAN_POINT ( 'NONE',  ( 19.93618820068612152, -3.269999999999996909, -36.05349808876643181 ) ) ;
#62143=DIRECTION ( 'NONE',  ( 0.000000000000000000, 0.000000000000000000, -1.000000000000000000 ) ) ;
#62168=EDGE_LOOP ( 'NONE', ( #26504, #30713, #126703, #34982 ) ) ;
#62171=CIRCLE ( 'NONE', #136244, 3.000000000000000888 ) ;
#62209=( GEOMETRIC_REPRESENTATION_CONTEXT ( 3 ) GLOBAL_UNCERTAINTY_ASSIGNED_CONTEXT ( ( #137328 ) ) GLOBAL_UNIT_ASSIGNED_CONTEXT ( ( #94250, #124745, #4317 ) ) REPRESENTATION_CONTEXT ( 'NONE', 'WORKASPACE' ) );
#62215=VECTOR ( 'NONE', #114800, 1000.000000000000114 ) ;
#62219=EDGE_CURVE ( 'NONE', #78214, #39230, #86173, .T. ) ;
#62255=SURFACE_STYLE_FILL_AREA ( #84030 ) ;
#62297=CARTESIAN_POINT ( 'NONE',  ( 12.69999999999999574, -40.43000000000000682, 19.45086547876359617 ) ) ;
#62360=CARTESIAN_POINT ( 'NONE',  ( 6.932893218813437564, -40.13710678118655295, -40.00000000000000000 ) ) ;
#62362=LINE ( 'NONE', #7936, #119133 ) ;
#62386=ORIENTED_EDGE ( 'NONE', *, *, #79247, .F. ) ;
#62414=( GEOMETRIC_REPRESENTATION_CONTEXT ( 3 ) GLOBAL_UNCERTAINTY_ASSIGNED_CONTEXT ( ( #98431 ) ) GLOBAL_UNIT_ASSIGNED_CONTEXT ( ( #119110, #53127, #108200 ) ) REPRESENTATION_CONTEXT ( 'NONE', 'WORKASPACE' ) );
#62417=LINE ( 'NONE', #41340, #53230 ) ;
#62426=ADVANCED_FACE ( 'NONE', ( #69431 ), #135410, .F. ) ;
#62436=DIRECTION ( 'NONE',  ( 0.000000000000000000, 0.000000000000000000, 1.000000000000000000 ) ) ;
#62457=CARTESIAN_POINT ( 'NONE',  ( 7.139999999999955271, -35.56014942880460694, -8.278119684037269721 ) ) ;
#62475=ORIENTED_EDGE ( 'NONE', *, *, #50570, .T. ) ;
#62479=VECTOR ( 'NONE', #94897, 1000.000000000000000 ) ;
#62503=CIRCLE ( 'NONE', #74080, 2.247900000000000453 ) ;
#62504=VECTOR ( 'NONE', #10009, 1000.000000000000000 ) ;
#62515=CARTESIAN_POINT ( 'NONE',  ( 34.92500000000002558, -21.76999999999999247, 0.000000000000000000 ) ) ;
#62524=EDGE_LOOP ( 'NONE', ( #56331, #110330, #54704 ) ) ;
#62534=EDGE_LOOP ( 'NONE', ( #141128, #1684, #104983, #121310 ) ) ;
#62546=DIRECTION ( 'NONE',  ( -1.000000000000000000, 3.654646145370261567E-15, 0.000000000000000000 ) ) ;
#62549=ORIENTED_EDGE ( 'NONE', *, *, #27339, .F. ) ;
#62586=DIRECTION ( 'NONE',  ( 0.000000000000000000, 0.000000000000000000, 1.000000000000000000 ) ) ;
#62588=DIRECTION ( 'NONE',  ( 0.000000000000000000, -1.000000000000000000, 0.000000000000000000 ) ) ;
#62612=CARTESIAN_POINT ( 'NONE',  ( -7.940000000000007496, -35.76999999999998892, -10.00000000000000178 ) ) ;
#62651=CARTESIAN_POINT ( 'NONE',  ( -16.55914779396249514, 0.6742760034310938400, -33.57941237570724979 ) ) ;
#62652=ORIENTED_EDGE ( 'NONE', *, *, #104680, .T. ) ;
#62674=EDGE_CURVE ( 'NONE', #58061, #55041, #127124, .T. ) ;
#62696=( NAMED_UNIT ( * ) PLANE_ANGLE_UNIT ( ) SI_UNIT ( $, .RADIAN. ) );
#62725=EDGE_LOOP ( 'NONE', ( #102447, #43521, #122974, #94509 ) ) ;
#62736=CARTESIAN_POINT ( 'NONE',  ( 12.10645530542133841, 7.761932032390377323, -28.16843179005226006 ) ) ;
#62760=EDGE_LOOP ( 'NONE', ( #9621, #6729, #76450 ) ) ;
#62767=PRESENTATION_STYLE_ASSIGNMENT (( #117803 ) ) ;
#62775=DIRECTION ( 'NONE',  ( -1.000000000000000000, 0.000000000000000000, 0.000000000000000000 ) ) ;
#62789=MECHANICAL_DESIGN_GEOMETRIC_PRESENTATION_REPRESENTATION('',(#141518),#122997);
#62862=EDGE_CURVE ( 'NONE', #80081, #17782, #39185, .T. ) ;
#62995=( GEOMETRIC_REPRESENTATION_CONTEXT ( 3 ) GLOBAL_UNCERTAINTY_ASSIGNED_CONTEXT ( ( #31919 ) ) GLOBAL_UNIT_ASSIGNED_CONTEXT ( ( #61810, #17547, #48070 ) ) REPRESENTATION_CONTEXT ( 'NONE', 'WORKASPACE' ) );
#63051=( NAMED_UNIT ( * ) PLANE_ANGLE_UNIT ( ) SI_UNIT ( $, .RADIAN. ) );
#63061=DIRECTION ( 'NONE',  ( 1.000000000000000000, -1.248002500702738701E-15, 0.000000000000000000 ) ) ;
#63067=LINE ( 'NONE', #140577, #113150 ) ;
#63119=SURFACE_STYLE_USAGE ( .BOTH. , #18110 ) ;
#63131=( GEOMETRIC_REPRESENTATION_CONTEXT ( 3 ) GLOBAL_UNCERTAINTY_ASSIGNED_CONTEXT ( ( #103937 ) ) GLOBAL_UNIT_ASSIGNED_CONTEXT ( ( #48620, #47250, #26158 ) ) REPRESENTATION_CONTEXT ( 'NONE', 'WORKASPACE' ) );
#63181=AXIS2_PLACEMENT_3D ( 'NONE', #70883, #41080, #82458 ) ;
#63191=CARTESIAN_POINT ( 'NONE',  ( 0.4414447833044549130, 12.59086548424452090, -26.73346183226842498 ) ) ;
#63196=DIRECTION ( 'NONE',  ( 1.000000000000000000, 3.115803279706882722E-16, -0.000000000000000000 ) ) ;
#63277=SURFACE_STYLE_FILL_AREA ( #32031 ) ;
#63305=ORIENTED_EDGE ( 'NONE', *, *, #45748, .T. ) ;
#63324=VERTEX_POINT ( 'NONE', #128972 ) ;
#63341=CARTESIAN_POINT ( 'NONE',  ( -6.932893218813454439, -40.13710678118653874, -40.00000000000000000 ) ) ;
#63349=DIRECTION ( 'NONE',  ( -0.000000000000000000, -1.000000000000000000, -0.000000000000000000 ) ) ;
#63353=VECTOR ( 'NONE', #18479, 1000.000000000000000 ) ;
#63364=EDGE_CURVE ( 'NONE', #129025, #4192, #75328, .T. ) ;
#63390=ORIENTED_EDGE ( 'NONE', *, *, #13335, .T. ) ;
#63392=CARTESIAN_POINT ( 'NONE',  ( -16.96322138488664066, -0.7337853718385520807, -35.15696433214895933 ) ) ;
#63433=AXIS2_PLACEMENT_3D ( 'NONE', #60862, #84708, #8520 ) ;
#63465=CARTESIAN_POINT ( 'NONE',  ( -3.244551382801596606, 12.29205737877197713, -27.00337393511194151 ) ) ;
#63479=AXIS2_PLACEMENT_3D ( 'NONE', #982, #101018, #45266 ) ;
#63518=EDGE_LOOP ( 'NONE', ( #53547, #123093, #130983, #139775 ) ) ;
#63533=UNCERTAINTY_MEASURE_WITH_UNIT (LENGTH_MEASURE( 1.000000000000000082E-05 ), #98576, 'distance_accuracy_value', 'NONE');
#63611=DIRECTION ( 'NONE',  ( 0.000000000000000000, -0.2631995976047492580, -0.9647414015272165466 ) ) ;
#63646=LINE ( 'NONE', #51326, #130282 ) ;
#63685=SURFACE_SIDE_STYLE ('',( #31745 ) ) ;
#63692=ADVANCED_FACE ( 'NONE', ( #50794 ), #103034, .F. ) ;
#63694=FILL_AREA_STYLE_COLOUR ( '', #100453 ) ;
#63767=CARTESIAN_POINT ( 'NONE',  ( -12.20000000000000284, -35.14999999999999147, 17.49210858042621908 ) ) ;
#63775=CARTESIAN_POINT ( 'NONE',  ( 19.91089914266474281, -3.052838087030619096, -34.75743929853354786 ) ) ;
#63786=PRESENTATION_STYLE_ASSIGNMENT (( #30430 ) ) ;
#63864=AXIS2_PLACEMENT_3D ( 'NONE', #139653, #40332, #70813 ) ;
#63907=DIRECTION ( 'NONE',  ( 1.000000000000000000, 0.000000000000000000, 0.000000000000000000 ) ) ;
#63920=CARTESIAN_POINT ( 'NONE',  ( 0.000000000000000000, -21.76999999999999247, -0.5000000000000000000 ) ) ;
#63936=EDGE_CURVE ( 'NONE', #28467, #7925, #89143, .T. ) ;
#63984=VERTEX_POINT ( 'NONE', #134072 ) ;
#64007=DIRECTION ( 'NONE',  ( 1.248002500702736137E-15, 1.000000000000000000, 0.000000000000000000 ) ) ;
#64050=ORIENTED_EDGE ( 'NONE', *, *, #45248, .T. ) ;
#64101=EDGE_CURVE ( 'NONE', #31365, #53394, #25601, .T. ) ;
#64151=CARTESIAN_POINT ( 'NONE',  ( 0.9490416316764018756, 12.57141199504220808, -25.28239494629447037 ) ) ;
#64153=DIRECTION ( 'NONE',  ( 1.000000000000000000, -0.000000000000000000, -0.000000000000000000 ) ) ;
#64172=CARTESIAN_POINT ( 'NONE',  ( -12.70000000000000462, -22.26999999999999247, -39.50000000000000000 ) ) ;
#64184=DIRECTION ( 'NONE',  ( 1.000000000000000000, -0.000000000000000000, -0.000000000000000000 ) ) ;
#64199=CARTESIAN_POINT ( 'NONE',  ( -7.122370700763609008, -39.92999999999999261, 19.06900128115122328 ) ) ;
#64204=VERTEX_POINT ( 'NONE', #52052 ) ;
#64260=DIRECTION ( 'NONE',  ( 0.000000000000000000, 0.000000000000000000, 1.000000000000000000 ) ) ;
#64319=VERTEX_POINT ( 'NONE', #76681 ) ;
#64363=VERTEX_POINT ( 'NONE', #132504 ) ;
#64407=DIRECTION ( 'NONE',  ( 1.000000000000000000, -1.248002500702738504E-15, 3.404785525682858480E-16 ) ) ;
#64414=AXIS2_PLACEMENT_3D ( 'NONE', #46712, #122775, #69135 ) ;
#64433=ORIENTED_EDGE ( 'NONE', *, *, #36778, .F. ) ;
#64469=ORIENTED_EDGE ( 'NONE', *, *, #1223, .F. ) ;
#64485=AXIS2_PLACEMENT_3D ( 'NONE', #31859, #43449, #42761 ) ;
#64507=SURFACE_SIDE_STYLE ('',( #121723 ) ) ;
#64511=ORIENTED_EDGE ( 'NONE', *, *, #10016, .F. ) ;
#64519=ORIENTED_EDGE ( 'NONE', *, *, #6966, .T. ) ;
#64598=CARTESIAN_POINT ( 'NONE',  ( 12.19999999999999574, 12.19802518668052649, 4.711086268963014412 ) ) ;
#64691=EDGE_CURVE ( 'NONE', #142234, #40966, #44271, .T. ) ;
#64719=PLANE ( 'NONE',  #31976 ) ;
#64776=CIRCLE ( 'NONE', #87943, 2.247899999999996901 ) ;
#64785=AXIS2_PLACEMENT_3D ( 'NONE', #62612, #84380, #128568 ) ;
#64870=CARTESIAN_POINT ( 'NONE',  ( -5.035040864892940782, 11.85438914953258305, -27.38739306153288311 ) ) ;
#64894=SURFACE_SIDE_STYLE ('',( #110491 ) ) ;
#64988=AXIS2_PLACEMENT_3D ( 'NONE', #43330, #129597, #21575 ) ;
#65037=ORIENTED_EDGE ( 'NONE', *, *, #68056, .F. ) ;
#65059=EDGE_CURVE ( 'NONE', #128930, #14912, #54414, .T. ) ;
#65069=STYLED_ITEM ( 'NONE', ( #129136 ), #142469 ) ;
#65078=( LENGTH_UNIT ( ) NAMED_UNIT ( * ) SI_UNIT ( .MILLI., .METRE. ) );
#65102=VECTOR ( 'NONE', #47318, 1000.000000000000000 ) ;
#65160=ORIENTED_EDGE ( 'NONE', *, *, #120338, .T. ) ;
#65174=AXIS2_PLACEMENT_3D ( 'NONE', #105723, #85405, #138385 ) ;
#65191=CARTESIAN_POINT ( 'NONE',  ( 12.69999999999999574, -22.26999999999999247, -0.5000000000000004441 ) ) ;
#65207=ORIENTED_EDGE ( 'NONE', *, *, #54934, .T. ) ;
#65211=EDGE_CURVE ( 'NONE', #13983, #92723, #6364, .T. ) ;
#65214=FILL_AREA_STYLE ('',( #50744 ) ) ;
#65265=STYLED_ITEM ( 'NONE', ( #54381 ), #131675 ) ;
#65292=( NAMED_UNIT ( * ) SI_UNIT ( $, .STERADIAN. ) SOLID_ANGLE_UNIT ( ) );
#65315=ORIENTED_EDGE ( 'NONE', *, *, #53095, .F. ) ;
#65327=CARTESIAN_POINT ( 'NONE',  ( 2.335353848949925037, 12.43939446707911678, -26.87120046541300766 ) ) ;
#65330=LINE ( 'NONE', #42142, #49884 ) ;
#65382=MECHANICAL_DESIGN_GEOMETRIC_PRESENTATION_REPRESENTATION('',(#134819),#95456);
#65386=ORIENTED_EDGE ( 'NONE', *, *, #63364, .T. ) ;
#65394=ORIENTED_EDGE ( 'NONE', *, *, #10204, .F. ) ;
#65400=LINE ( 'NONE', #59, #54299 ) ;
#65406=DIRECTION ( 'NONE',  ( 0.000000000000000000, 0.000000000000000000, -1.000000000000000000 ) ) ;
#65438=ORIENTED_EDGE ( 'NONE', *, *, #77651, .F. ) ;
#65472=PRESENTATION_STYLE_ASSIGNMENT (( #99463 ) ) ;
#65551=TOROIDAL_SURFACE ( 'NONE', #132706, 2.500000000000000000, 0.5000000000000000000 ) ;
#65614=CARTESIAN_POINT ( 'NONE',  ( -0.9646429025310692129, 12.58792797458966284, -26.73614525879442994 ) ) ;
#65628=EDGE_CURVE ( 'NONE', #51304, #129328, #28208, .T. ) ;
#65632=AXIS2_PLACEMENT_3D ( 'NONE', #116224, #70623, #3839 ) ;
#65662=DIRECTION ( 'NONE',  ( 0.000000000000000000, 0.000000000000000000, -1.000000000000000000 ) ) ;
#65663=MECHANICAL_DESIGN_GEOMETRIC_PRESENTATION_REPRESENTATION('',(#111990),#95716);
#65677=DIRECTION ( 'NONE',  ( 0.000000000000000000, 0.000000000000000000, -1.000000000000000000 ) ) ;
#65699=LINE ( 'NONE', #9071, #48432 ) ;
#65721=CARTESIAN_POINT ( 'NONE',  ( -19.93618820137057668, -6.270000000050818478, -36.99999999997771738 ) ) ;
#65731=( NAMED_UNIT ( * ) SI_UNIT ( $, .STERADIAN. ) SOLID_ANGLE_UNIT ( ) );
#65732=EDGE_LOOP ( 'NONE', ( #21994, #126677, #57649, #23089 ) ) ;
#65744=CIRCLE ( 'NONE', #33343, 0.5000000000000004441 ) ;
#65791=EDGE_CURVE ( 'NONE', #109867, #58061, #73662, .T. ) ;
#65808=ORIENTED_EDGE ( 'NONE', *, *, #130115, .F. ) ;
#65904=ADVANCED_FACE ( 'NONE', ( #76535, #101104, #89524 ), #133753, .T. ) ;
#65909=( BOUNDED_CURVE ( )  B_SPLINE_CURVE ( 3, ( #92259, #124195, #27732, #135111 ),
 .UNSPECIFIED., .F., .T. ) 
 B_SPLINE_CURVE_WITH_KNOTS ( ( 4, 4 ),
 ( 3.141592653589798889, 4.446051736530363563 ),
 .UNSPECIFIED. ) 
 CURVE ( )  GEOMETRIC_REPRESENTATION_ITEM ( )  RATIONAL_B_SPLINE_CURVE ( ( 1.000000000000000000, 0.8631550219135040170, 0.8631550219135040170, 1.000000000000000000 ) ) 
 REPRESENTATION_ITEM ( '' )  );
#65955=CARTESIAN_POINT ( 'NONE',  ( 12.19999999999999574, -40.43000000000000682, 19.06900128115122683 ) ) ;
#65998=ORIENTED_EDGE ( 'NONE', *, *, #58667, .F. ) ;
#66007=AXIS2_PLACEMENT_3D ( 'NONE', #74420, #6948, #85989 ) ;
#66055=SURFACE_STYLE_FILL_AREA ( #42875 ) ;
#66090=LINE ( 'NONE', #23252, #138444 ) ;
#66112=CARTESIAN_POINT ( 'NONE',  ( 34.42500000000002558, -22.26999999999999247, 0.000000000000000000 ) ) ;
#66131=CARTESIAN_POINT ( 'NONE',  ( 12.69999999999999574, -27.68200100598810565, 15.59110741220538188 ) ) ;
#66168=DIRECTION ( 'NONE',  ( 1.000000000000000000, 0.000000000000000000, 0.000000000000000000 ) ) ;
#66186=LINE ( 'NONE', #56042, #118044 ) ;
#66225=DIRECTION ( 'NONE',  ( 1.321231229586337907E-16, -0.9647414015272155474, 0.2631995976047525887 ) ) ;
#66298=CARTESIAN_POINT ( 'NONE',  ( 13.39767433127539498, 6.360963242914233540, -31.21237421153560021 ) ) ;
#66322=FILL_AREA_STYLE ('',( #121385 ) ) ;
#66345=DIRECTION ( 'NONE',  ( 0.000000000000000000, -1.000000000000000000, -0.000000000000000000 ) ) ;
#66371=VECTOR ( 'NONE', #81108, 1000.000000000000000 ) ;
#66402=AXIS2_PLACEMENT_3D ( 'NONE', #114041, #116894, #14732 ) ;
#66430=EDGE_CURVE ( 'NONE', #3531, #60140, #105227, .T. ) ;
#66477=ADVANCED_FACE ( 'NONE', ( #21611 ), #32495, .F. ) ;
#66506=UNCERTAINTY_MEASURE_WITH_UNIT (LENGTH_MEASURE( 1.000000000000000082E-05 ), #60554, 'distance_accuracy_value', 'NONE');
#66527=ORIENTED_EDGE ( 'NONE', *, *, #59446, .T. ) ;
#66531=AXIS2_PLACEMENT_3D ( 'NONE', #92041, #89904, #58778 ) ;
#66604=CARTESIAN_POINT ( 'NONE',  ( 12.49289321881344605, -22.06289321881344634, -3.073261146000583341E-16 ) ) ;
#66641=( NAMED_UNIT ( * ) SI_UNIT ( $, .STERADIAN. ) SOLID_ANGLE_UNIT ( ) );
#66677=CARTESIAN_POINT ( 'NONE',  ( 16.84504724602342662, -0.2737008427375496322, -34.33975653689201124 ) ) ;
#66710=ORIENTED_EDGE ( 'NONE', *, *, #59442, .F. ) ;
#66722=DIRECTION ( 'NONE',  ( -0.2248289345038712861, 0.9743982503113672866, -2.004349902429943025E-16 ) ) ;
#66772=AXIS2_PLACEMENT_3D ( 'NONE', #97457, #140964, #38287 ) ;
#66782=EDGE_CURVE ( 'NONE', #137008, #20082, #6940, .T. ) ;
#66802=CARTESIAN_POINT ( 'NONE',  ( 12.69999999999999574, 0.000000000000000000, -39.50000000000000000 ) ) ;
#66804=CARTESIAN_POINT ( 'NONE',  ( 1.953608656376216022E-15, -6.270000000000002238, -37.00000000000000000 ) ) ;
#66809=FACE_OUTER_BOUND ( 'NONE', #31739, .T. ) ;
#66859=VECTOR ( 'NONE', #29696, 1000.000000000000000 ) ;
#66861=DIRECTION ( 'NONE',  ( -0.000000000000000000, -0.000000000000000000, 1.000000000000000000 ) ) ;
#66874=DIRECTION ( 'NONE',  ( -0.000000000000000000, 1.000000000000000000, -0.000000000000000000 ) ) ;
#66934=CARTESIAN_POINT ( 'NONE',  ( 0.000000000000000000, -4.870000000000014317, -40.00000000000000000 ) ) ;
#66948=VERTEX_POINT ( 'NONE', #126369 ) ;
#66960=CARTESIAN_POINT ( 'NONE',  ( -7.140000000000001457, -35.56014942880461405, -8.278119684037248405 ) ) ;
#66987=SURFACE_SIDE_STYLE ('',( #135806 ) ) ;
#66988=CARTESIAN_POINT ( 'NONE',  ( -12.70000000000000284, -34.64999999999999147, 17.49210858042622263 ) ) ;
#67022=STYLED_ITEM ( 'NONE', ( #43312 ), #127113 ) ;
#67095=ORIENTED_EDGE ( 'NONE', *, *, #122040, .T. ) ;
#67121=CARTESIAN_POINT ( 'NONE',  ( -19.75037474193593567, -1.784389841569742785, -32.42466272773691571 ) ) ;
#67226=CARTESIAN_POINT ( 'NONE',  ( 17.47198025047039494, -2.800541402284825843, -34.03206192796267970 ) ) ;
#67237=CIRCLE ( 'NONE', #48718, 3.000000000000000000 ) ;
#67255=EDGE_CURVE ( 'NONE', #96844, #140981, #138621, .T. ) ;
#67275=PRESENTATION_STYLE_ASSIGNMENT (( #46260 ) ) ;
#67304=DIRECTION ( 'NONE',  ( -1.000000000000000000, -0.000000000000000000, -0.000000000000000000 ) ) ;
#67351=CIRCLE ( 'NONE', #4769, 1.898649999999994842 ) ;
#67375=VERTEX_POINT ( 'NONE', #10909 ) ;
#67378=ORIENTED_EDGE ( 'NONE', *, *, #47975, .F. ) ;
#67411=CYLINDRICAL_SURFACE ( 'NONE', #116040, 9.524999999999995026 ) ;
#67431=CARTESIAN_POINT ( 'NONE',  ( -7.140000000000001457, -39.92999999999999261, -7.899272885403729738 ) ) ;
#67532=ORIENTED_EDGE ( 'NONE', *, *, #118347, .T. ) ;
#67575=DIRECTION ( 'NONE',  ( 0.000000000000000000, 0.2631995976047483699, 0.9647414015272167687 ) ) ;
#67607=FILL_AREA_STYLE ('',( #1560 ) ) ;
#67613=LINE ( 'NONE', #111802, #125810 ) ;
#67642=AXIS2_PLACEMENT_3D ( 'NONE', #76894, #108023, #43517 ) ;
#67651=ORIENTED_EDGE ( 'NONE', *, *, #121803, .T. ) ;
#67672=TOROIDAL_SURFACE ( 'NONE', #30599, 31.92999999999999261, 3.000000000000000000 ) ;
#67692=ORIENTED_EDGE ( 'NONE', *, *, #28429, .F. ) ;
#67696=EDGE_CURVE ( 'NONE', #126832, #113508, #61619, .T. ) ;
#67728=SURFACE_STYLE_USAGE ( .BOTH. , #35088 ) ;
#67754=EDGE_CURVE ( 'NONE', #75784, #55041, #38411, .T. ) ;
#67787=EDGE_LOOP ( 'NONE', ( #9269, #67095, #58852 ) ) ;
#67864=CARTESIAN_POINT ( 'NONE',  ( 9.524999999999991473, -4.870000000000013429, -10.00000000000000178 ) ) ;
#67876=( LENGTH_UNIT ( ) NAMED_UNIT ( * ) SI_UNIT ( .MILLI., .METRE. ) );
#67908=SURFACE_STYLE_USAGE ( .BOTH. , #135967 ) ;
#67962=ORIENTED_EDGE ( 'NONE', *, *, #35240, .F. ) ;
#67982=SURFACE_STYLE_USAGE ( .BOTH. , #78107 ) ;
#68026=CARTESIAN_POINT ( 'NONE',  ( -34.42499999999997584, -21.76999999999999247, 0.000000000000000000 ) ) ;
#68056=EDGE_CURVE ( 'NONE', #111777, #122541, #35421, .T. ) ;
#68110=CARTESIAN_POINT ( 'NONE',  ( -34.42499999999997584, 0.000000000000000000, -0.5000000000000000000 ) ) ;
#68169=ORIENTED_EDGE ( 'NONE', *, *, #133838, .T. ) ;
#68246=DIRECTION ( 'NONE',  ( 0.000000000000000000, 0.2631995976047483699, 0.9647414015272167687 ) ) ;
#68266=CARTESIAN_POINT ( 'NONE',  ( 19.04500000000000881, 3.130000000000007887, -2.396719511207313368E-16 ) ) ;
#68286=ORIENTED_EDGE ( 'NONE', *, *, #58854, .T. ) ;
#68307=EDGE_LOOP ( 'NONE', ( #64469, #51957, #139019, #115685 ) ) ;
#68325=CARTESIAN_POINT ( 'NONE',  ( 16.52898522435346607, 6.019049105522195298, -28.93301309892516215 ) ) ;
#68375=DIRECTION ( 'NONE',  ( 2.496005001405478586E-15, 1.000000000000000000, -0.000000000000000000 ) ) ;
#68381=EDGE_LOOP ( 'NONE', ( #67378, #135259 ) ) ;
#68481=CARTESIAN_POINT ( 'NONE',  ( -12.19999999999999574, -60.26999999999998892, 25.00000000000000000 ) ) ;
#68510=SURFACE_STYLE_USAGE ( .BOTH. , #3883 ) ;
#68517=VERTEX_POINT ( 'NONE', #106680 ) ;
#68568=CARTESIAN_POINT ( 'NONE',  ( -17.33028271673254750, -2.068042672074010380, -32.75052031823620524 ) ) ;
#68571=SURFACE_STYLE_FILL_AREA ( #134535 ) ;
#68591=FACE_OUTER_BOUND ( 'NONE', #131003, .T. ) ;
#68595=FILL_AREA_STYLE_COLOUR ( '', #80176 ) ;
#68649=CARTESIAN_POINT ( 'NONE',  ( -33.81889366174460321, 22.27000000000001023, -13.38643001103286423 ) ) ;
#68723=CIRCLE ( 'NONE', #6141, 1.898649999999994842 ) ;
#68788=COLOUR_RGB ( '', 0.72549020, 0.75294118, 0.79215686) ;
#68791=( NAMED_UNIT ( * ) SI_UNIT ( $, .STERADIAN. ) SOLID_ANGLE_UNIT ( ) );
#68793=AXIS2_PLACEMENT_3D ( 'NONE', #117725, #130078, #140240 ) ;
#68800=CYLINDRICAL_SURFACE ( 'NONE', #41271, 0.5000000000000000000 ) ;
#68828=ORIENTED_EDGE ( 'NONE', *, *, #1970, .F. ) ;
#68905=FILL_AREA_STYLE_COLOUR ( '', #135952 ) ;
#68928=AXIS2_PLACEMENT_3D ( 'NONE', #4819, #17183, #73701 ) ;
#68966=SURFACE_SIDE_STYLE ('',( #26852 ) ) ;
#68968=DIRECTION ( 'NONE',  ( -3.115803279706882722E-16, 1.000000000000000000, 0.000000000000000000 ) ) ;
#69043=DIRECTION ( 'NONE',  ( 0.000000000000000000, 1.000000000000000000, 0.000000000000000000 ) ) ;
#69082=CARTESIAN_POINT ( 'NONE',  ( -34.42499999999997584, -21.76999999999999247, -0.5000000000000000000 ) ) ;
#69135=DIRECTION ( 'NONE',  ( -1.000000000000000000, 0.000000000000000000, 0.000000000000000000 ) ) ;
#69214=CARTESIAN_POINT ( 'NONE',  ( -7.140000000000001457, -39.92999999999999261, -40.00000000000000000 ) ) ;
#69271=PRESENTATION_STYLE_ASSIGNMENT (( #12716 ) ) ;
#69293=ORIENTED_EDGE ( 'NONE', *, *, #100410, .F. ) ;
#69298=EDGE_LOOP ( 'NONE', ( #52122, #140517, #65808, #90963 ) ) ;
#69300=FACE_OUTER_BOUND ( 'NONE', #83446, .T. ) ;
#69329=ORIENTED_EDGE ( 'NONE', *, *, #58854, .F. ) ;
#69342=AXIS2_PLACEMENT_3D ( 'NONE', #125564, #69043, #1583 ) ;
#69344=VECTOR ( 'NONE', #16008, 1000.000000000000000 ) ;
#69357=CARTESIAN_POINT ( 'NONE',  ( 12.19999999999999574, -28.33999999999998565, 13.17925390838734323 ) ) ;
#69378=CARTESIAN_POINT ( 'NONE',  ( 16.96838079760940232, -0.7556382844926715636, -35.24774147208035657 ) ) ;
#69416=CIRCLE ( 'NONE', #6838, 2.552699999999997971 ) ;
#69431=FACE_OUTER_BOUND ( 'NONE', #11745, .T. ) ;
#69471=ORIENTED_EDGE ( 'NONE', *, *, #45770, .T. ) ;
#69508=( LENGTH_UNIT ( ) NAMED_UNIT ( * ) SI_UNIT ( .MILLI., .METRE. ) );
#69509=CARTESIAN_POINT ( 'NONE',  ( -12.69999999999999929, -59.76999999999998892, -40.00000000000000000 ) ) ;
#69521=( BOUNDED_CURVE ( )  B_SPLINE_CURVE ( 3, ( #75253, #50622, #7066, #20108 ),
 .UNSPECIFIED., .F., .T. ) 
 B_SPLINE_CURVE_WITH_KNOTS ( ( 4, 4 ),
 ( 0.000000000000000000, 1.570796326794896558 ),
 .UNSPECIFIED. ) 
 CURVE ( )  GEOMETRIC_REPRESENTATION_ITEM ( )  RATIONAL_B_SPLINE_CURVE ( ( 1.000000000000000000, 0.8047378541243649375, 0.8047378541243649375, 1.000000000000000000 ) ) 
 REPRESENTATION_ITEM ( '' )  );
#69545=( GEOMETRIC_REPRESENTATION_CONTEXT ( 3 ) GLOBAL_UNCERTAINTY_ASSIGNED_CONTEXT ( ( #112863 ) ) GLOBAL_UNIT_ASSIGNED_CONTEXT ( ( #130384, #73845, #8534 ) ) REPRESENTATION_CONTEXT ( 'NONE', 'WORKASPACE' ) );
#69694=ORIENTED_EDGE ( 'NONE', *, *, #77316, .F. ) ;
#69746=CARTESIAN_POINT ( 'NONE',  ( -7.217967065889526523, 12.56012801747615448, -25.25494078541189680 ) ) ;
#69754=CARTESIAN_POINT ( 'NONE',  ( 31.92500000000001492, -6.269999999999992468, -37.00000000000000000 ) ) ;
#69841=AXIS2_PLACEMENT_3D ( 'NONE', #90578, #134814, #123218 ) ;
#69849=SURFACE_SIDE_STYLE ('',( #137931 ) ) ;
#69871=CARTESIAN_POINT ( 'NONE',  ( 6.639999999999984581, -40.29840020119762301, 19.55137198191483350 ) ) ;
#69873=SURFACE_STYLE_USAGE ( .BOTH. , #66987 ) ;
#69889=MECHANICAL_DESIGN_GEOMETRIC_PRESENTATION_REPRESENTATION('',(#49070),#28255);
#69904=VERTEX_POINT ( 'NONE', #31494 ) ;
#69905=DIRECTION ( 'NONE',  ( 0.000000000000000000, 0.000000000000000000, -1.000000000000000000 ) ) ;
#69982=CARTESIAN_POINT ( 'NONE',  ( -12.19999999999999929, -59.76999999999998892, -39.50000000000000000 ) ) ;
#70068=CARTESIAN_POINT ( 'NONE',  ( -11.54697671733239872, 10.46529571468478181, -26.63845132861668930 ) ) ;
#70096=CARTESIAN_POINT ( 'NONE',  ( 12.19999999999999574, -40.43000000000000682, 19.06900128115122683 ) ) ;
#70125=CARTESIAN_POINT ( 'NONE',  ( 16.77034657092882597, -0.01012368044107444208, -34.06770708329295161 ) ) ;
#70169=DIRECTION ( 'NONE',  ( -1.000000000000000000, 0.000000000000000000, 0.000000000000000000 ) ) ;
#70170=CARTESIAN_POINT ( 'NONE',  ( 0.000000000000000000, -4.870000000000014317, -40.00000000000000000 ) ) ;
#70234=VERTEX_POINT ( 'NONE', #114056 ) ;
#70256=CARTESIAN_POINT ( 'NONE',  ( 31.92500000000002203, -21.76999999999999247, -40.00000000000000000 ) ) ;
#70335=LINE ( 'NONE', #136243, #37031 ) ;
#70339=EDGE_CURVE ( 'NONE', #58156, #13978, #83261, .T. ) ;
#70391=ORIENTED_EDGE ( 'NONE', *, *, #93437, .F. ) ;
#70457=LINE ( 'NONE', #106564, #85815 ) ;
#70484=CARTESIAN_POINT ( 'NONE',  ( 12.19999999999999574, -34.51840020119763608, 17.97447928118983640 ) ) ;
#70542=DIRECTION ( 'NONE',  ( 1.000000000000000000, 0.000000000000000000, 0.000000000000000000 ) ) ;
#70553=DIRECTION ( 'NONE',  ( 0.000000000000000000, 0.000000000000000000, 1.000000000000000000 ) ) ;
#70559=EDGE_CURVE ( 'NONE', #106633, #67375, #109600, .T. ) ;
#70613=MECHANICAL_DESIGN_GEOMETRIC_PRESENTATION_REPRESENTATION('',(#10322),#8045);
#70623=DIRECTION ( 'NONE',  ( 0.000000000000000000, 0.000000000000000000, 1.000000000000000000 ) ) ;
#70624=ORIENTED_EDGE ( 'NONE', *, *, #66782, .F. ) ;
#70758=ADVANCED_FACE ( 'NONE', ( #105149 ), #80566, .T. ) ;
#70779=VERTEX_POINT ( 'NONE', #137800 ) ;
#70783=CARTESIAN_POINT ( 'NONE',  ( 12.69999999999999574, -22.26999999999999247, -39.79289321881344677 ) ) ;
#70813=DIRECTION ( 'NONE',  ( -1.000000000000000000, -1.369518533665899572E-16, 0.000000000000000000 ) ) ;
#70816=FACE_OUTER_BOUND ( 'NONE', #97147, .T. ) ;
#70830=DIRECTION ( 'NONE',  ( 1.049727191138614875E-16, -0.5150380749100594846, 0.8571673007021091140 ) ) ;
#70856=SPHERICAL_SURFACE ( 'NONE', #41473, 0.5000000000000000000 ) ;
#70860=SURFACE_STYLE_USAGE ( .BOTH. , #114335 ) ;
#70883=CARTESIAN_POINT ( 'NONE',  ( 12.19999999999999574, -25.83999999999998565, 2.999999999999999112 ) ) ;
#70925=FILL_AREA_STYLE_COLOUR ( '', #28035 ) ;
#70960=ORIENTED_EDGE ( 'NONE', *, *, #97500, .T. ) ;
#70970=CIRCLE ( 'NONE', #8402, 2.552699999999994418 ) ;
#71009=CARTESIAN_POINT ( 'NONE',  ( -34.42499999999997584, -21.76999999999999247, -0.5000000000000000000 ) ) ;
#71016=CARTESIAN_POINT ( 'NONE',  ( 19.93618820137057668, -6.269999999999996021, -37.00000000000000000 ) ) ;
#71063=( NAMED_UNIT ( * ) PLANE_ANGLE_UNIT ( ) SI_UNIT ( $, .RADIAN. ) );
#71097=EDGE_LOOP ( 'NONE', ( #113650, #28644, #127996, #89495 ) ) ;
#71132=DIRECTION ( 'NONE',  ( 1.000000000000000000, 3.469446951953611428E-15, -9.465303761398244822E-16 ) ) ;
#71137=( LENGTH_UNIT ( ) NAMED_UNIT ( * ) SI_UNIT ( .MILLI., .METRE. ) );
#71157=CARTESIAN_POINT ( 'NONE',  ( -1.089366964280113814, 13.74372519030773532, -24.36966481856508437 ) ) ;
#71183=VERTEX_POINT ( 'NONE', #82522 ) ;
#71259=CARTESIAN_POINT ( 'NONE',  ( -19.28515664589289003, 1.963325189347658428, -33.49048331797055766 ) ) ;
#71272=EDGE_CURVE ( 'NONE', #118457, #72919, #94090, .T. ) ;
#71304=ORIENTED_EDGE ( 'NONE', *, *, #27339, .T. ) ;
#71326=EDGE_CURVE ( 'NONE', #38058, #42501, #128182, .T. ) ;
#71385=CARTESIAN_POINT ( 'NONE',  ( -14.08979869950237074, -1.618973607074043475, -36.99999999997771738 ) ) ;
#71455=CARTESIAN_POINT ( 'NONE',  ( -9.853871626853138110, 9.550302695096817729, -29.19944056394587761 ) ) ;
#71490=CARTESIAN_POINT ( 'NONE',  ( -34.64589307847458599, 22.27000000000001023, -11.14749280822901767 ) ) ;
#71544=ORIENTED_EDGE ( 'NONE', *, *, #8418, .T. ) ;
#71596=EDGE_LOOP ( 'NONE', ( #21014, #112264, #133219, #42426 ) ) ;
#71629=SURFACE_STYLE_USAGE ( .BOTH. , #27370 ) ;
#71636=SURFACE_SIDE_STYLE ('',( #55956 ) ) ;
#71646=ORIENTED_EDGE ( 'NONE', *, *, #87129, .F. ) ;
#71736=CARTESIAN_POINT ( 'NONE',  ( 12.69999999999999574, -22.26999999999999247, -0.5000000000000004441 ) ) ;
#71785=VERTEX_POINT ( 'NONE', #3000 ) ;
#71803=VERTEX_POINT ( 'NONE', #2256 ) ;
#71835=ORIENTED_EDGE ( 'NONE', *, *, #63936, .T. ) ;
#71838=VECTOR ( 'NONE', #78804, 1000.000000000000000 ) ;
#71867=FACE_OUTER_BOUND ( 'NONE', #22395, .T. ) ;
#71870=CARTESIAN_POINT ( 'NONE',  ( 7.122370700763592133, -39.92999999999999972, 19.06900128115122328 ) ) ;
#71898=LINE ( 'NONE', #105200, #103257 ) ;
#71906=ORIENTED_EDGE ( 'NONE', *, *, #134000, .F. ) ;
#71949=SPHERICAL_SURFACE ( 'NONE', #40552, 0.5000000000000000000 ) ;
#71951=PRESENTATION_STYLE_ASSIGNMENT (( #126992 ) ) ;
#72019=ADVANCED_FACE ( 'NONE', ( #71867 ), #124787, .F. ) ;
#72043=CYLINDRICAL_SURFACE ( 'NONE', #65632, 0.5000000000000004441 ) ;
#72049=STYLED_ITEM ( 'NONE', ( #12930 ), #84438 ) ;
#72148=EDGE_LOOP ( 'NONE', ( #118369, #110479, #4226, #65037 ) ) ;
#72151=SURFACE_STYLE_FILL_AREA ( #115563 ) ;
#72200=ADVANCED_FACE ( 'NONE', ( #35512 ), #122458, .F. ) ;
#72224=MECHANICAL_DESIGN_GEOMETRIC_PRESENTATION_REPRESENTATION('',(#93081),#62995);
#72264=ADVANCED_FACE ( 'NONE', ( #131944 ), #67411, .F. ) ;
#72325=( GEOMETRIC_REPRESENTATION_CONTEXT ( 3 ) GLOBAL_UNCERTAINTY_ASSIGNED_CONTEXT ( ( #130196 ) ) GLOBAL_UNIT_ASSIGNED_CONTEXT ( ( #96070, #46768, #12638 ) ) REPRESENTATION_CONTEXT ( 'NONE', 'WORKASPACE' ) );
#72366=FACE_OUTER_BOUND ( 'NONE', #134277, .T. ) ;
#72397=CIRCLE ( 'NONE', #83974, 1.898649999999993065 ) ;
#72401=CARTESIAN_POINT ( 'NONE',  ( -34.92499999999997584, -6.270000000000012008, -37.00000000000000000 ) ) ;
#72436=ORIENTED_EDGE ( 'NONE', *, *, #127583, .T. ) ;
#72442=UNCERTAINTY_MEASURE_WITH_UNIT (LENGTH_MEASURE( 1.000000000000000082E-05 ), #34641, 'distance_accuracy_value', 'NONE');
#72464=MECHANICAL_DESIGN_GEOMETRIC_PRESENTATION_REPRESENTATION('',(#58615),#14562);
#72465=DIRECTION ( 'NONE',  ( -1.000000000000000000, 0.000000000000000000, 0.000000000000000000 ) ) ;
#72493=ORIENTED_EDGE ( 'NONE', *, *, #46465, .T. ) ;
#72546=ADVANCED_FACE ( 'NONE', ( #7073 ), #129593, .F. ) ;
#72551=ORIENTED_EDGE ( 'NONE', *, *, #100523, .T. ) ;
#72556=FACE_OUTER_BOUND ( 'NONE', #44964, .T. ) ;
#72575=ORIENTED_EDGE ( 'NONE', *, *, #65211, .F. ) ;
#72599=DIRECTION ( 'NONE',  ( -1.451651444332056451E-15, -1.000000000000000000, 0.000000000000000000 ) ) ;
#72651=ORIENTED_EDGE ( 'NONE', *, *, #10204, .T. ) ;
#72652=APPLICATION_CONTEXT ( 'automotive_design' ) ;
#72653=CARTESIAN_POINT ( 'NONE',  ( -9.900005234295676360, 9.518575983135214358, -29.22208412987195914 ) ) ;
#72654=CARTESIAN_POINT ( 'NONE',  ( -19.05499999999999261, 3.130000000000007887, 0.000000000000000000 ) ) ;
#72661=EDGE_CURVE ( 'NONE', #39230, #129328, #54233, .T. ) ;
#72687=VECTOR ( 'NONE', #63061, 1000.000000000000000 ) ;
#72738=ORIENTED_EDGE ( 'NONE', *, *, #84570, .F. ) ;
#72760=DIRECTION ( 'NONE',  ( 0.000000000000000000, 0.000000000000000000, 1.000000000000000000 ) ) ;
#72776=VERTEX_POINT ( 'NONE', #46944 ) ;
#72824=ORIENTED_EDGE ( 'NONE', *, *, #64101, .F. ) ;
#72851=DIRECTION ( 'NONE',  ( -0.000000000000000000, -1.000000000000000000, -0.000000000000000000 ) ) ;
#72889=DIRECTION ( 'NONE',  ( 0.000000000000000000, 1.000000000000000000, 0.000000000000000000 ) ) ;
#72919=VERTEX_POINT ( 'NONE', #19955 ) ;
#72922=EDGE_CURVE ( 'NONE', #135430, #21068, #50470, .T. ) ;
#72973=FACE_OUTER_BOUND ( 'NONE', #110120, .T. ) ;
#73017=DIRECTION ( 'NONE',  ( 0.000000000000000000, 1.000000000000000000, 0.000000000000000000 ) ) ;
#73036=DIRECTION ( 'NONE',  ( 0.000000000000000000, 0.000000000000000000, -1.000000000000000000 ) ) ;
#73050=VERTEX_POINT ( 'NONE', #32287 ) ;
#73119=B_SPLINE_CURVE_WITH_KNOTS ( 'NONE', 3,
 ( #45926, #122014, #24155, #92240, #122744, #13961, #14704, #124182, #58264, #22681, #58981, #11821, #79299, #2362, #111883, #90113, #114014, #80004, #102453, #56105 ),
 .UNSPECIFIED., .F., .F.,
 ( 4, 2, 2, 2, 2, 2, 2, 2, 2, 4 ),
 ( 3.469446951953614189E-18, 0.002043365256125570517, 0.003065047884188353174, 0.004086730512251135830, 0.005108413140313918487, 0.006130095768376701143, 0.006640937082408094640, 0.007151778396439487269, 0.007662619710470881633, 0.008173461024502275130 ),
 .UNSPECIFIED. ) ;
#73138=EDGE_CURVE ( 'NONE', #116824, #103756, #13988, .T. ) ;
#73265=CARTESIAN_POINT ( 'NONE',  ( 7.139999999999985469, -39.92999999999999972, 18.93259187797431764 ) ) ;
#73299=VECTOR ( 'NONE', #140454, 1000.000000000000000 ) ;
#73335=CARTESIAN_POINT ( 'NONE',  ( -14.95213108811772784, 4.188779951252514344, -32.28871390651440976 ) ) ;
#73433=ORIENTED_EDGE ( 'NONE', *, *, #60595, .F. ) ;
#73471=EDGE_CURVE ( 'NONE', #92630, #132295, #120455, .T. ) ;
#73472=SPHERICAL_SURFACE ( 'NONE', #41916, 0.5000000000000000000 ) ;
#73496=CIRCLE ( 'NONE', #85065, 2.499999999999998668 ) ;
#73540=SURFACE_STYLE_FILL_AREA ( #119847 ) ;
#73543=CARTESIAN_POINT ( 'NONE',  ( -12.19999999999999929, -59.76999999999998892, -39.50000000000000000 ) ) ;
#73589=EDGE_LOOP ( 'NONE', ( #121535, #114149, #32574, #735 ) ) ;
#73593=EDGE_CURVE ( 'NONE', #68517, #100573, #46674, .T. ) ;
#73596=CARTESIAN_POINT ( 'NONE',  ( 11.08707631394196724, 10.76818482829728829, -26.45687733286667154 ) ) ;
#73618=CARTESIAN_POINT ( 'NONE',  ( 7.139999999999997904, -35.14999999999999858, 17.49210858042622263 ) ) ;
#73622=ORIENTED_EDGE ( 'NONE', *, *, #85080, .F. ) ;
#73662=LINE ( 'NONE', #141789, #123120 ) ;
#73698=EDGE_LOOP ( 'NONE', ( #89265, #65438, #108915, #11128 ) ) ;
#73701=DIRECTION ( 'NONE',  ( 1.000000000000000000, 0.000000000000000000, 0.000000000000000000 ) ) ;
#73727=SURFACE_SIDE_STYLE ('',( #37553 ) ) ;
#73754=EDGE_CURVE ( 'NONE', #34379, #50924, #28085, .T. ) ;
#73783=CARTESIAN_POINT ( 'NONE',  ( 12.19999999999999574, -28.33999999999998565, 13.17925390838734323 ) ) ;
#73823=UNCERTAINTY_MEASURE_WITH_UNIT (LENGTH_MEASURE( 1.000000000000000082E-05 ), #40008, 'distance_accuracy_value', 'NONE');
#73831=( NAMED_UNIT ( * ) PLANE_ANGLE_UNIT ( ) SI_UNIT ( $, .RADIAN. ) );
#73845=( NAMED_UNIT ( * ) PLANE_ANGLE_UNIT ( ) SI_UNIT ( $, .RADIAN. ) );
#73888=COLOUR_RGB ( '', 0.09019608, 0.27058824, 0.51372549) ;
#73905=FACE_OUTER_BOUND ( 'NONE', #103681, .T. ) ;
#73941=EDGE_CURVE ( 'NONE', #59938, #137008, #104443, .T. ) ;
#74017=ORIENTED_EDGE ( 'NONE', *, *, #9084, .F. ) ;
#74077=CYLINDRICAL_SURFACE ( 'NONE', #138239, 1.898649999999994842 ) ;
#74080=AXIS2_PLACEMENT_3D ( 'NONE', #74193, #63349, #107519 ) ;
#74086=CARTESIAN_POINT ( 'NONE',  ( -55.65468426143998215, -34.51840020119762187, 17.97447928118982929 ) ) ;
#74136=LINE ( 'NONE', #28501, #44703 ) ;
#74159=VECTOR ( 'NONE', #94789, 1000.000000000000000 ) ;
#74193=CARTESIAN_POINT ( 'NONE',  ( -7.940000000000007496, -60.26999999999998892, -10.00000000000000178 ) ) ;
#74219=ORIENTED_EDGE ( 'NONE', *, *, #40855, .F. ) ;
#74297=DIRECTION ( 'NONE',  ( 0.000000000000000000, 0.000000000000000000, 1.000000000000000000 ) ) ;
#74309=EDGE_CURVE ( 'NONE', #64363, #61603, #40427, .T. ) ;
#74318=CARTESIAN_POINT ( 'NONE',  ( 1.826117250740552755, 12.50058190090600441, -26.81569114864833381 ) ) ;
#74361=LINE ( 'NONE', #27985, #38171 ) ;
#74371=CARTESIAN_POINT ( 'NONE',  ( 7.939999999999994174, -60.26999999999998892, -7.752100000000004876 ) ) ;
#74380=CARTESIAN_POINT ( 'NONE',  ( -19.05499999999999261, 3.130000000000007887, -22.35000000000000142 ) ) ;
#74409=CIRCLE ( 'NONE', #11855, 2.247899999999996901 ) ;
#74420=CARTESIAN_POINT ( 'NONE',  ( -12.20000000000000284, -25.83999999999998920, 13.17925390838734323 ) ) ;
#74479=( GEOMETRIC_REPRESENTATION_CONTEXT ( 3 ) GLOBAL_UNCERTAINTY_ASSIGNED_CONTEXT ( ( #33190 ) ) GLOBAL_UNIT_ASSIGNED_CONTEXT ( ( #75858, #141839, #13414 ) ) REPRESENTATION_CONTEXT ( 'NONE', 'WORKASPACE' ) );
#74508=ORIENTED_EDGE ( 'NONE', *, *, #86397, .T. ) ;
#74511=EDGE_LOOP ( 'NONE', ( #102966, #6789, #129092, #18600, #117712, #112267, #27046 ) ) ;
#74513=ORIENTED_EDGE ( 'NONE', *, *, #63936, .F. ) ;
#74598=ADVANCED_FACE ( 'NONE', ( #141758 ), #86661, .T. ) ;
#74625=STYLED_ITEM ( 'NONE', ( #90709 ), #26149 ) ;
#74636=EDGE_CURVE ( 'NONE', #50410, #108517, #79389, .T. ) ;
#74722=( NAMED_UNIT ( * ) SI_UNIT ( $, .STERADIAN. ) SOLID_ANGLE_UNIT ( ) );
#74729=ORIENTED_EDGE ( 'NONE', *, *, #95027, .T. ) ;
#74750=( NAMED_UNIT ( * ) PLANE_ANGLE_UNIT ( ) SI_UNIT ( $, .RADIAN. ) );
#74777=CARTESIAN_POINT ( 'NONE',  ( 6.639999999999993463, -34.51840020119762897, 17.97447928118983285 ) ) ;
#74799=CARTESIAN_POINT ( 'NONE',  ( 0.000000000000000000, -4.870000000000014317, -36.99999999997771738 ) ) ;
#74863=EDGE_LOOP ( 'NONE', ( #56949, #132796, #124056 ) ) ;
#74891=DIRECTION ( 'NONE',  ( -0.000000000000000000, 1.000000000000000000, -0.000000000000000000 ) ) ;
#74973=EDGE_CURVE ( 'NONE', #42501, #85630, #7456, .T. ) ;
#74975=CARTESIAN_POINT ( 'NONE',  ( -21.60769999999998703, 3.130000000000008331, 0.000000000000000000 ) ) ;
#74984=COLOUR_RGB ( '', 0.72549020, 0.75294118, 0.79215686) ;
#74985=PLANE ( 'NONE',  #91643 ) ;
#75037=AXIS2_PLACEMENT_3D ( 'NONE', #130712, #62586, #87890 ) ;
#75049=CARTESIAN_POINT ( 'NONE',  ( 2.682347683340221334, 13.58957659137172591, -24.48930257366534846 ) ) ;
#75055=CARTESIAN_POINT ( 'NONE',  ( 12.19999999999999574, -40.43000000000000682, -39.50000000000000000 ) ) ;
#75211=ORIENTED_EDGE ( 'NONE', *, *, #105266, .F. ) ;
#75237=EDGE_CURVE ( 'NONE', #72919, #83224, #136931, .T. ) ;
#75253=CARTESIAN_POINT ( 'NONE',  ( -12.70000000000000462, -22.26999999999999247, -0.5000000000000004441 ) ) ;
#75294=DIRECTION ( 'NONE',  ( 0.000000000000000000, 0.000000000000000000, -1.000000000000000000 ) ) ;
#75328=LINE ( 'NONE', #86193, #62479 ) ;
#75350=ORIENTED_EDGE ( 'NONE', *, *, #40258, .F. ) ;
#75468=CARTESIAN_POINT ( 'NONE',  ( -1.915787159634013470, 12.50960769155452468, -26.80828596576004941 ) ) ;
#75475=CARTESIAN_POINT ( 'NONE',  ( 6.932893218813446445, -34.80096641561353010, 18.05156865852269021 ) ) ;
#75500=CARTESIAN_POINT ( 'NONE',  ( -12.19999999999999929, -59.76999999999998892, -39.50000000000000000 ) ) ;
#75537=ORIENTED_EDGE ( 'NONE', *, *, #45168, .F. ) ;
#75547=SURFACE_STYLE_USAGE ( .BOTH. , #8791 ) ;
#75646=ORIENTED_EDGE ( 'NONE', *, *, #117639, .F. ) ;
#75667=DIRECTION ( 'NONE',  ( -0.000000000000000000, -0.000000000000000000, 1.000000000000000000 ) ) ;
#75703=CARTESIAN_POINT ( 'NONE',  ( 7.940000000000001279, -35.14999999999999858, -8.101350000000007157 ) ) ;
#75704=ORIENTED_EDGE ( 'NONE', *, *, #22505, .T. ) ;
#75741=CARTESIAN_POINT ( 'NONE',  ( 4.546519005068298647, 12.01231087727541968, -27.25263027609279831 ) ) ;
#75784=VERTEX_POINT ( 'NONE', #76530 ) ;
#75847=ORIENTED_EDGE ( 'NONE', *, *, #88898, .T. ) ;
#75858=( LENGTH_UNIT ( ) NAMED_UNIT ( * ) SI_UNIT ( .MILLI., .METRE. ) );
#75862=DIRECTION ( 'NONE',  ( 0.000000000000000000, 0.000000000000000000, 1.000000000000000000 ) ) ;
#75934=FILL_AREA_STYLE ('',( #107817 ) ) ;
#75946=LINE ( 'NONE', #119417, #99316 ) ;
#75963=PLANE ( 'NONE',  #55461 ) ;
#75975=DIRECTION ( 'NONE',  ( 3.115803279706882722E-16, -1.000000000000000000, 0.000000000000000000 ) ) ;
#76009=( GEOMETRIC_REPRESENTATION_CONTEXT ( 3 ) GLOBAL_UNCERTAINTY_ASSIGNED_CONTEXT ( ( #102567 ) ) GLOBAL_UNIT_ASSIGNED_CONTEXT ( ( #21150, #41467, #108844 ) ) REPRESENTATION_CONTEXT ( 'NONE', 'WORKASPACE' ) );
#76127=DIRECTION ( 'NONE',  ( 1.369518533665900312E-16, -1.000000000000000000, 0.000000000000000000 ) ) ;
#76158=CARTESIAN_POINT ( 'NONE',  ( -7.140000000000001457, -35.62922597241578160, -11.84864515520818706 ) ) ;
#76188=CARTESIAN_POINT ( 'NONE',  ( 19.04500000000000171, 3.130000000000007887, -23.88381690219165776 ) ) ;
#76229=CARTESIAN_POINT ( 'NONE',  ( -12.70000000000000284, -40.42999999999999261, 19.06900128115121973 ) ) ;
#76269=AXIS2_PLACEMENT_3D ( 'NONE', #71385, #84419, #4616 ) ;
#76272=ORIENTED_EDGE ( 'NONE', *, *, #94898, .T. ) ;
#76305=CARTESIAN_POINT ( 'NONE',  ( -19.93618820135885272, -3.270000000000008455, -36.39086428169088094 ) ) ;
#76325=( NAMED_UNIT ( * ) SI_UNIT ( $, .STERADIAN. ) SOLID_ANGLE_UNIT ( ) );
#76417=EDGE_CURVE ( 'NONE', #87140, #78214, #125132, .T. ) ;
#76420=DIRECTION ( 'NONE',  ( -1.000000000000000000, 0.000000000000000000, 0.000000000000000000 ) ) ;
#76449=DIRECTION ( 'NONE',  ( 1.000000000000000000, 8.854317741964955179E-16, 0.000000000000000000 ) ) ;
#76450=ORIENTED_EDGE ( 'NONE', *, *, #54527, .T. ) ;
#76455=( GEOMETRIC_REPRESENTATION_CONTEXT ( 3 ) GLOBAL_UNCERTAINTY_ASSIGNED_CONTEXT ( ( #5489 ) ) GLOBAL_UNIT_ASSIGNED_CONTEXT ( ( #69508, #136877, #16501 ) ) REPRESENTATION_CONTEXT ( 'NONE', 'WORKASPACE' ) );
#76465=CARTESIAN_POINT ( 'NONE',  ( 7.952899274893373338, 10.68804939725090541, -26.53793298327174455 ) ) ;
#76508=CARTESIAN_POINT ( 'NONE',  ( 12.19999999999999574, -40.43000000000000682, -39.50000000000000000 ) ) ;
#76516=LINE ( 'NONE', #54758, #20679 ) ;
#76530=CARTESIAN_POINT ( 'NONE',  ( -31.92499999999997584, -6.270000000000012008, -40.00000000000000000 ) ) ;
#76535=FACE_BOUND ( 'NONE', #68381, .T. ) ;
#76536=UNCERTAINTY_MEASURE_WITH_UNIT (LENGTH_MEASURE( 1.000000000000000082E-05 ), #56860, 'distance_accuracy_value', 'NONE');
#76549=AXIS2_PLACEMENT_3D ( 'NONE', #119957, #20670, #9798 ) ;
#76585=SURFACE_STYLE_FILL_AREA ( #32346 ) ;
#76681=CARTESIAN_POINT ( 'NONE',  ( -12.19999999999999929, -60.26999999999998892, -39.50000000000000000 ) ) ;
#76730=DIRECTION ( 'NONE',  ( -0.000000000000000000, -0.000000000000000000, 1.000000000000000000 ) ) ;
#76743=DIRECTION ( 'NONE',  ( -0.000000000000000000, 1.000000000000000000, 2.242629915582283412E-16 ) ) ;
#76752=EDGE_CURVE ( 'NONE', #32290, #38181, #99318, .T. ) ;
#76789=EDGE_LOOP ( 'NONE', ( #115371, #22603, #82702, #48563, #115280, #16020 ) ) ;
#76791=VECTOR ( 'NONE', #106501, 1000.000000000000000 ) ;
#76826=SURFACE_STYLE_USAGE ( .BOTH. , #56521 ) ;
#76847=( NAMED_UNIT ( * ) SI_UNIT ( $, .STERADIAN. ) SOLID_ANGLE_UNIT ( ) );
#76894=CARTESIAN_POINT ( 'NONE',  ( -7.940000000000007496, -35.76999999999998892, -10.00000000000000178 ) ) ;
#76952=CARTESIAN_POINT ( 'NONE',  ( -55.65468426143998215, -25.33999999999998920, 13.17925390838734323 ) ) ;
#77023=CARTESIAN_POINT ( 'NONE',  ( -34.42499999999997584, -21.76999999999999247, -0.5000000000000000000 ) ) ;
#77036=CIRCLE ( 'NONE', #120971, 0.5000000000000004441 ) ;
#77076=CARTESIAN_POINT ( 'NONE',  ( 19.04500000000000881, 3.130000000000007887, -2.396719511207313368E-16 ) ) ;
#77097=ADVANCED_FACE ( 'NONE', ( #25706 ), #36580, .T. ) ;
#77138=CIRCLE ( 'NONE', #61007, 6.000000000000000000 ) ;
#77169=VECTOR ( 'NONE', #50061, 1000.000000000000000 ) ;
#77181=CARTESIAN_POINT ( 'NONE',  ( 31.92500000000001492, -3.269999999999992468, -37.00000000000000000 ) ) ;
#77195=( NAMED_UNIT ( * ) PLANE_ANGLE_UNIT ( ) SI_UNIT ( $, .RADIAN. ) );
#77200=ORIENTED_EDGE ( 'NONE', *, *, #141052, .F. ) ;
#77202=CARTESIAN_POINT ( 'NONE',  ( -12.20000000000000107, -34.51840020119762187, 17.97447928118982929 ) ) ;
#77316=EDGE_CURVE ( 'NONE', #87614, #131559, #15508, .T. ) ;
#77365=CARTESIAN_POINT ( 'NONE',  ( 0.000000000000000000, -21.76999999999999247, -39.50000000000000000 ) ) ;
#77395=EDGE_CURVE ( 'NONE', #44308, #112461, #17470, .T. ) ;
#77417=ORIENTED_EDGE ( 'NONE', *, *, #120535, .T. ) ;
#77436=DIRECTION ( 'NONE',  ( -1.000000000000000000, -3.115803279706882722E-16, 0.000000000000000000 ) ) ;
#77458=FACE_OUTER_BOUND ( 'NONE', #10763, .T. ) ;
#77460=ORIENTED_EDGE ( 'NONE', *, *, #57217, .F. ) ;
#77539=CARTESIAN_POINT ( 'NONE',  ( 7.139999999999992575, -35.14999999999999858, -40.00000000000000000 ) ) ;
#77544=ORIENTED_EDGE ( 'NONE', *, *, #17622, .F. ) ;
#77548=LINE ( 'NONE', #121716, #56583 ) ;
#77558=ADVANCED_FACE ( 'NONE', ( #110180 ), #5055, .F. ) ;
#77567=CARTESIAN_POINT ( 'NONE',  ( -6.994446791092093669E-14, -39.92999999999999261, 19.06900128115121618 ) ) ;
#77603=CARTESIAN_POINT ( 'NONE',  ( -7.140000000000001457, -35.69931899287965393, -11.97485302731578294 ) ) ;
#77610=VERTEX_POINT ( 'NONE', #134108 ) ;
#77617=CARTESIAN_POINT ( 'NONE',  ( 14.08979869950237074, -1.618973607074033483, -36.99999999997771738 ) ) ;
#77629=VECTOR ( 'NONE', #16322, 1000.000000000000000 ) ;
#77630=ORIENTED_EDGE ( 'NONE', *, *, #106837, .T. ) ;
#77631=ORIENTED_EDGE ( 'NONE', *, *, #33306, .T. ) ;
#77651=EDGE_CURVE ( 'NONE', #54868, #32290, #4219, .T. ) ;
#77690=CARTESIAN_POINT ( 'NONE',  ( -12.20000000000000284, -40.42999999999999261, 19.06900128115121973 ) ) ;
#77704=EDGE_LOOP ( 'NONE', ( #56295, #83155, #54214, #108724 ) ) ;
#77713=AXIS2_PLACEMENT_3D ( 'NONE', #1775, #136611, #47528 ) ;
#77750=SURFACE_SIDE_STYLE ('',( #42274 ) ) ;
#77805=PRESENTATION_STYLE_ASSIGNMENT (( #79275 ) ) ;
#77849=DIRECTION ( 'NONE',  ( 0.000000000000000000, 0.000000000000000000, -1.000000000000000000 ) ) ;
#77864=SURFACE_SIDE_STYLE ('',( #126863 ) ) ;
#77905=COLOUR_RGB ( '', 0.72549020, 0.75294118, 0.79215686) ;
#77928=UNCERTAINTY_MEASURE_WITH_UNIT (LENGTH_MEASURE( 1.000000000000000082E-05 ), #7896, 'distance_accuracy_value', 'NONE');
#77935=CARTESIAN_POINT ( 'NONE',  ( 16.49230000000001439, 3.130000000000008331, -22.35000000000000142 ) ) ;
#77987=LINE ( 'NONE', #46086, #135106 ) ;
#77990=MECHANICAL_DESIGN_GEOMETRIC_PRESENTATION_REPRESENTATION('',(#45615),#89558);
#78005=CARTESIAN_POINT ( 'NONE',  ( -17.43071299949562558, -2.562240267135510230, -33.48616200217535521 ) ) ;
#78035=DIRECTION ( 'NONE',  ( 0.000000000000000000, 0.000000000000000000, -1.000000000000000000 ) ) ;
#78057=FACE_OUTER_BOUND ( 'NONE', #62725, .T. ) ;
#78107=SURFACE_SIDE_STYLE ('',( #112166 ) ) ;
#78180=DIRECTION ( 'NONE',  ( 0.000000000000000000, 0.000000000000000000, 1.000000000000000000 ) ) ;
#78213=CARTESIAN_POINT ( 'NONE',  ( 31.92500000000002203, -22.26999999999999247, -37.00000000000000000 ) ) ;
#78214=VERTEX_POINT ( 'NONE', #16793 ) ;
#78234=DIRECTION ( 'NONE',  ( -0.000000000000000000, -0.000000000000000000, -1.000000000000000000 ) ) ;
#78237=VERTEX_POINT ( 'NONE', #62457 ) ;
#78240=DIRECTION ( 'NONE',  ( 0.000000000000000000, 0.000000000000000000, 1.000000000000000000 ) ) ;
#78268=CARTESIAN_POINT ( 'NONE',  ( 7.139999999999992575, -35.14999999999999858, -8.278119684037271497 ) ) ;
#78367=DIRECTION ( 'NONE',  ( -1.400468248933914810E-15, -0.9647414015272155474, 0.2631995976047525887 ) ) ;
#78396=CARTESIAN_POINT ( 'NONE',  ( -7.140000000000001457, -34.64999999999999147, 17.49210858042621908 ) ) ;
#78456=CARTESIAN_POINT ( 'NONE',  ( 6.671778046239097648, 12.72213433738527932, -25.13690993948508279 ) ) ;
#78523=DIRECTION ( 'NONE',  ( 1.000000000000000000, -2.496005001405478586E-15, -0.000000000000000000 ) ) ;
#78530=( BOUNDED_CURVE ( )  B_SPLINE_CURVE ( 3, ( #18480, #61357, #27967, #39578 ),
 .UNSPECIFIED., .F., .T. ) 
 B_SPLINE_CURVE_WITH_KNOTS ( ( 4, 4 ),
 ( 4.446051736530344911, 4.712388980384676351 ),
 .UNSPECIFIED. ) 
 CURVE ( )  GEOMETRIC_REPRESENTATION_ITEM ( )  RATIONAL_B_SPLINE_CURVE ( ( 1.000000000000000000, 0.9940974367313476501, 0.9940974367313476501, 1.000000000000000000 ) ) 
 REPRESENTATION_ITEM ( '' )  );
#78560=AXIS2_PLACEMENT_3D ( 'NONE', #43354, #42661, #31759 ) ;
#78592=CARTESIAN_POINT ( 'NONE',  ( 15.78777360247684847, 2.639113497459678825, -32.92661230006952877 ) ) ;
#78611=( GEOMETRIC_REPRESENTATION_CONTEXT ( 3 ) GLOBAL_UNCERTAINTY_ASSIGNED_CONTEXT ( ( #109985 ) ) GLOBAL_UNIT_ASSIGNED_CONTEXT ( ( #65078, #30279, #44780 ) ) REPRESENTATION_CONTEXT ( 'NONE', 'WORKASPACE' ) );
#78640=CARTESIAN_POINT ( 'NONE',  ( 12.69999999999999574, -40.43000000000000682, -39.50000000000000000 ) ) ;
#78705=CARTESIAN_POINT ( 'NONE',  ( -17.53594656315045341, -3.178915670909185032, -35.18142205605356310 ) ) ;
#78714=AXIS2_PLACEMENT_3D ( 'NONE', #129579, #86098, #132496 ) ;
#78733=SURFACE_SIDE_STYLE ('',( #31130 ) ) ;
#78742=ORIENTED_EDGE ( 'NONE', *, *, #93437, .T. ) ;
#78776=DIRECTION ( 'NONE',  ( 0.000000000000000000, -0.2631995976047557528, -0.9647414015272147703 ) ) ;
#78794=CLOSED_SHELL ( 'NONE', ( #133086, #38349, #72546, #13615, #26510, #117793, #136365, #66477, #133701, #72019, #107130, #72264, #47075, #141893, #72200, #92115, #32540, #56651, #114939, #74598, #106085, #139027, #25816, #131675, #47523, #91052, #106917, #55317, #63692, #110241, #65904, #57613, #58768, #84973, #142559, #100104, #54318, #41862, #48749, #26149, #133441, #19464, #143376, #93708, #98629, #133817, #114719, #115617, #106840, #143366, #86209, #129368, #110939, #143506, #139343, #127113, #84438, #15692, #103236, #78835, #58892, #16183, #7388, #99545, #93406, #125643, #141940, #2383, #108794, #105787, #103281, #125244, #125339, #62426, #85041, #77558, #125580, #26443, #93243, #10753, #108151, #92223, #19986, #25167, #110201, #35298, #18081, #105432, #128393, #49885, #78880, #34222, #113957, #138335, #10291, #82686, #82436, #70758, #56487, #59055, #110713, #87051, #131539, #26079, #77097, #7572, #134883, #91109, #24973, #81576, #40615, #106493, #86090, #28613, #100968, #116939, #139757, #107167, #136326, #51857, #39442, #21239, #84766, #103912, #84590, #3417, #129181, #133542, #84585 ) ) ;
#78804=DIRECTION ( 'NONE',  ( 0.000000000000000000, 0.000000000000000000, 1.000000000000000000 ) ) ;
#78823=MECHANICAL_DESIGN_GEOMETRIC_PRESENTATION_REPRESENTATION('',(#115811),#130052);
#78824=CARTESIAN_POINT ( 'NONE',  ( 16.55061708910404761, 0.6983515413187854071, -33.57195487390330157 ) ) ;
#78835=ADVANCED_FACE ( 'NONE', ( #131817 ), #22293, .T. ) ;
#78880=ADVANCED_FACE ( 'NONE', ( #96990 ), #107878, .T. ) ;
#78891=ORIENTED_EDGE ( 'NONE', *, *, #87004, .T. ) ;
#79021=FACE_OUTER_BOUND ( 'NONE', #73698, .T. ) ;
#79071=EDGE_CURVE ( 'NONE', #59778, #99826, #93998, .T. ) ;
#79099=VECTOR ( 'NONE', #37082, 1000.000000000000000 ) ;
#79153=MECHANICAL_DESIGN_GEOMETRIC_PRESENTATION_REPRESENTATION('',(#21155),#37418);
#79163=CARTESIAN_POINT ( 'NONE',  ( -17.01299345043647548, -0.9444868035624306435, 500000.0000000000582 ) ) ;
#79211=ORIENTED_EDGE ( 'NONE', *, *, #112253, .F. ) ;
#79213=EDGE_CURVE ( 'NONE', #124237, #97431, #77987, .T. ) ;
#79247=EDGE_CURVE ( 'NONE', #122313, #13983, #35566, .T. ) ;
#79271=VECTOR ( 'NONE', #22816, 1000.000000000000000 ) ;
#79273=LINE ( 'NONE', #123474, #118975 ) ;
#79275=SURFACE_STYLE_USAGE ( .BOTH. , #88691 ) ;
#79299=CARTESIAN_POINT ( 'NONE',  ( 33.40690130215642029, 22.26999999999999957, -13.94180635367735555 ) ) ;
#79346=VERTEX_POINT ( 'NONE', #16240 ) ;
#79389=LINE ( 'NONE', #98927, #28297 ) ;
#79471=FILL_AREA_STYLE_COLOUR ( '', #28209 ) ;
#79480=COLOUR_RGB ( '', 0.08235294, 0.09019608, 0.10196078) ;
#79504=EDGE_CURVE ( 'NONE', #131250, #31365, #32905, .T. ) ;
#79557=CARTESIAN_POINT ( 'NONE',  ( -33.41687398106825668, 22.27000000000000668, -13.94762968036370054 ) ) ;
#79564=UNCERTAINTY_MEASURE_WITH_UNIT (LENGTH_MEASURE( 1.000000000000000082E-05 ), #33390, 'distance_accuracy_value', 'NONE');
#79578=CARTESIAN_POINT ( 'NONE',  ( 19.48939575397828960, -0.003013263964889829026, -31.00984187987698704 ) ) ;
#79626=DIRECTION ( 'NONE',  ( -0.000000000000000000, -0.000000000000000000, -1.000000000000000000 ) ) ;
#79639=ORIENTED_EDGE ( 'NONE', *, *, #35327, .F. ) ;
#79689=EDGE_CURVE ( 'NONE', #40406, #82818, #36962, .T. ) ;
#79752=VERTEX_POINT ( 'NONE', #51432 ) ;
#79756=DIRECTION ( 'NONE',  ( 0.000000000000000000, 0.000000000000000000, -1.000000000000000000 ) ) ;
#79772=EDGE_CURVE ( 'NONE', #44308, #40891, #72397, .T. ) ;
#79810=( NAMED_UNIT ( * ) SI_UNIT ( $, .STERADIAN. ) SOLID_ANGLE_UNIT ( ) );
#79825=AXIS2_PLACEMENT_3D ( 'NONE', #85712, #32067, #9568 ) ;
#79857=EDGE_CURVE ( 'NONE', #103352, #64319, #61135, .T. ) ;
#79868=SURFACE_STYLE_USAGE ( .BOTH. , #90715 ) ;
#79891=ORIENTED_EDGE ( 'NONE', *, *, #100005, .F. ) ;
#79923=CIRCLE ( 'NONE', #82186, 31.92999999999999261 ) ;
#79925=EDGE_LOOP ( 'NONE', ( #113779, #68286, #85888, #105090 ) ) ;
#79966=ORIENTED_EDGE ( 'NONE', *, *, #99136, .T. ) ;
#80004=CARTESIAN_POINT ( 'NONE',  ( 32.27133846272768380, 22.27000000000000668, -14.68128223927440956 ) ) ;
#80008=CYLINDRICAL_SURFACE ( 'NONE', #21084, 3.000000000000000000 ) ;
#80058=( NAMED_UNIT ( * ) SI_UNIT ( $, .STERADIAN. ) SOLID_ANGLE_UNIT ( ) );
#80066=FILL_AREA_STYLE ('',( #88784 ) ) ;
#80069=EDGE_CURVE ( 'NONE', #22073, #39230, #111784, .T. ) ;
#80081=VERTEX_POINT ( 'NONE', #128111 ) ;
#80127=AXIS2_PLACEMENT_3D ( 'NONE', #61045, #118192, #117481 ) ;
#80128=ORIENTED_EDGE ( 'NONE', *, *, #73138, .F. ) ;
#80132=DIRECTION ( 'NONE',  ( 1.000000000000000000, 0.000000000000000000, 0.000000000000000000 ) ) ;
#80160=CARTESIAN_POINT ( 'NONE',  ( -19.48942811940429465, -0.003197019174711220046, -31.00987262783852572 ) ) ;
#80176=COLOUR_RGB ( '', 0.66274510, 0.83137255, 0.94901961) ;
#80182=EDGE_CURVE ( 'NONE', #46696, #22146, #77036, .T. ) ;
#80201=CARTESIAN_POINT ( 'NONE',  ( 19.93618820137057668, -3.269999999999996465, -36.39086428169088094 ) ) ;
#80213=( GEOMETRIC_REPRESENTATION_CONTEXT ( 3 ) GLOBAL_UNCERTAINTY_ASSIGNED_CONTEXT ( ( #82246 ) ) GLOBAL_UNIT_ASSIGNED_CONTEXT ( ( #95802, #19668, #10902 ) ) REPRESENTATION_CONTEXT ( 'NONE', 'WORKASPACE' ) );
#80249=CARTESIAN_POINT ( 'NONE',  ( -12.70000000000000284, -34.64999999999999147, -40.00000000000000000 ) ) ;
#80389=LINE ( 'NONE', #126022, #43669 ) ;
#80566=CYLINDRICAL_SURFACE ( 'NONE', #134288, 0.5000000000000004441 ) ;
#80613=CARTESIAN_POINT ( 'NONE',  ( 12.69999999999999574, -59.76999999999998892, -40.00000000000000000 ) ) ;
#80624=ORIENTED_EDGE ( 'NONE', *, *, #94898, .F. ) ;
#80630=VECTOR ( 'NONE', #8162, 1000.000000000000000 ) ;
#80658=AXIS2_PLACEMENT_3D ( 'NONE', #92636, #124576, #25251 ) ;
#80670=SURFACE_STYLE_USAGE ( .BOTH. , #36436 ) ;
#80700=DIRECTION ( 'NONE',  ( -3.115803279706882722E-16, 1.000000000000000000, 0.000000000000000000 ) ) ;
#80806=EDGE_CURVE ( 'NONE', #75784, #66948, #128140, .T. ) ;
#80842=CARTESIAN_POINT ( 'NONE',  ( -12.49289321881344783, -60.26999999999998181, 25.00000000000000355 ) ) ;
#80912=( GEOMETRIC_REPRESENTATION_CONTEXT ( 3 ) GLOBAL_UNCERTAINTY_ASSIGNED_CONTEXT ( ( #34787 ) ) GLOBAL_UNIT_ASSIGNED_CONTEXT ( ( #94824, #51366, #40498 ) ) REPRESENTATION_CONTEXT ( 'NONE', 'WORKASPACE' ) );
#80927=ORIENTED_EDGE ( 'NONE', *, *, #82792, .F. ) ;
#80965=CARTESIAN_POINT ( 'NONE',  ( 6.640000000000060965, 12.19802518668051583, 4.711086268963014412 ) ) ;
#81008=ORIENTED_EDGE ( 'NONE', *, *, #86207, .F. ) ;
#81049=AXIS2_PLACEMENT_3D ( 'NONE', #10197, #123811, #121103 ) ;
#81108=DIRECTION ( 'NONE',  ( 0.000000000000000000, -1.000000000000000000, 0.000000000000000000 ) ) ;
#81122=VERTEX_POINT ( 'NONE', #112656 ) ;
#81178=CARTESIAN_POINT ( 'NONE',  ( 7.139999999999991687, -35.62922597241576739, -11.84864515520817640 ) ) ;
#81186=DIRECTION ( 'NONE',  ( 1.000000000000000000, 3.115803279706882722E-16, -0.000000000000000000 ) ) ;
#81222=DIRECTION ( 'NONE',  ( 1.000000000000000000, 3.115803279706882722E-16, 0.000000000000000000 ) ) ;
#81330=PLANE ( 'NONE',  #11310 ) ;
#81400=FACE_OUTER_BOUND ( 'NONE', #132975, .T. ) ;
#81427=LINE ( 'NONE', #135098, #3816 ) ;
#81433=LINE ( 'NONE', #59670, #52615 ) ;
#81439=VERTEX_POINT ( 'NONE', #78268 ) ;
#81481=AXIS2_PLACEMENT_3D ( 'NONE', #56022, #100215, #45155 ) ;
#81524=VERTEX_POINT ( 'NONE', #103542 ) ;
#81544=CARTESIAN_POINT ( 'NONE',  ( 7.139999999999991687, -35.76999999999998892, -7.899272885403729738 ) ) ;
#81556=CIRCLE ( 'NONE', #90528, 2.499999999999998668 ) ;
#81573=CARTESIAN_POINT ( 'NONE',  ( 7.139999999999993463, -34.64999999999999858, 17.49210858042622263 ) ) ;
#81576=ADVANCED_FACE ( 'NONE', ( #101422 ), #112100, .T. ) ;
#81580=AXIS2_PLACEMENT_3D ( 'NONE', #88162, #22854, #108427 ) ;
#81621=DIRECTION ( 'NONE',  ( 1.321231229586337907E-16, -0.9647414015272155474, 0.2631995976047525887 ) ) ;
#81640=CARTESIAN_POINT ( 'NONE',  ( -14.47644487788491396, 4.930979942669944549, -31.94426976426194287 ) ) ;
#81647=LINE ( 'NONE', #13467, #26269 ) ;
#81655=FACE_OUTER_BOUND ( 'NONE', #53197, .T. ) ;
#81676=ORIENTED_EDGE ( 'NONE', *, *, #66782, .T. ) ;
#81678=AXIS2_PLACEMENT_3D ( 'NONE', #33626, #47387, #56824 ) ;
#81697=CARTESIAN_POINT ( 'NONE',  ( 17.01299345042646749, -0.9444868035190607802, -36.39086428169088094 ) ) ;
#81707=MECHANICAL_DESIGN_GEOMETRIC_PRESENTATION_REPRESENTATION('',(#100206),#109511);
#81735=MECHANICAL_DESIGN_GEOMETRIC_PRESENTATION_REPRESENTATION('',(#21481),#16821);
#81892=CIRCLE ( 'NONE', #86422, 0.5000000000000013323 ) ;
#81922=EDGE_CURVE ( 'NONE', #117423, #16702, #36702, .T. ) ;
#81937=SURFACE_SIDE_STYLE ('',( #24650 ) ) ;
#81959=EDGE_LOOP ( 'NONE', ( #84094, #96437, #68828, #34121 ) ) ;
#82000=FILL_AREA_STYLE_COLOUR ( '', #5225 ) ;
#82007=ORIENTED_EDGE ( 'NONE', *, *, #58667, .T. ) ;
#82041=CARTESIAN_POINT ( 'NONE',  ( 12.69999999999999574, -60.06289321881344279, 24.72882142070205091 ) ) ;
#82072=ORIENTED_EDGE ( 'NONE', *, *, #43324, .T. ) ;
#82124=ORIENTED_EDGE ( 'NONE', *, *, #95216, .F. ) ;
#82143=( NAMED_UNIT ( * ) SI_UNIT ( $, .STERADIAN. ) SOLID_ANGLE_UNIT ( ) );
#82164=SURFACE_SIDE_STYLE ('',( #47414 ) ) ;
#82171=SURFACE_STYLE_USAGE ( .BOTH. , #95858 ) ;
#82186=AXIS2_PLACEMENT_3D ( 'NONE', #93109, #63196, #103256 ) ;
#82246=UNCERTAINTY_MEASURE_WITH_UNIT (LENGTH_MEASURE( 1.000000000000000082E-05 ), #95802, 'distance_accuracy_value', 'NONE');
#82263=CARTESIAN_POINT ( 'NONE',  ( -12.70000000000000817, -1.739288537755694446E-15, -0.5000000000000004441 ) ) ;
#82283=AXIS2_PLACEMENT_3D ( 'NONE', #39004, #115091, #82513 ) ;
#82290=EDGE_LOOP ( 'NONE', ( #138277, #34857, #48189 ) ) ;
#82306=SHAPE_DEFINITION_REPRESENTATION ( #108328, #88538 ) ;
#82341=CARTESIAN_POINT ( 'NONE',  ( -13.57767111518905523, 9.030084587337581681, -27.47540428435809901 ) ) ;
#82353=CARTESIAN_POINT ( 'NONE',  ( 6.640000000000043201, -9.638965590364918103E-15, -40.00000000000000000 ) ) ;
#82381=UNCERTAINTY_MEASURE_WITH_UNIT (LENGTH_MEASURE( 1.000000000000000082E-05 ), #24133, 'distance_accuracy_value', 'NONE');
#82393=CARTESIAN_POINT ( 'NONE',  ( 19.93294383519271662, -3.241747265911685716, -35.72051902601952378 ) ) ;
#82400=ORIENTED_EDGE ( 'NONE', *, *, #112375, .T. ) ;
#82403=DIRECTION ( 'NONE',  ( 0.000000000000000000, -1.000000000000000000, 0.000000000000000000 ) ) ;
#82436=ADVANCED_FACE ( 'NONE', ( #84368 ), #73472, .T. ) ;
#82443=ORIENTED_EDGE ( 'NONE', *, *, #4280, .F. ) ;
#82458=DIRECTION ( 'NONE',  ( 1.000000000000000000, 0.000000000000000000, 0.000000000000000000 ) ) ;
#82460=EDGE_LOOP ( 'NONE', ( #67692, #119903, #103389, #93607 ) ) ;
#82475=EDGE_LOOP ( 'NONE', ( #42450, #48569, #113855, #95369 ) ) ;
#82513=DIRECTION ( 'NONE',  ( 0.000000000000000000, 0.000000000000000000, -1.000000000000000000 ) ) ;
#82517=DIRECTION ( 'NONE',  ( 0.000000000000000000, 0.000000000000000000, 1.000000000000000000 ) ) ;
#82522=CARTESIAN_POINT ( 'NONE',  ( 34.92500000000001847, -6.269999999999991580, -37.00000000000000000 ) ) ;
#82527=MECHANICAL_DESIGN_GEOMETRIC_PRESENTATION_REPRESENTATION('',(#89451),#117171);
#82554=TOROIDAL_SURFACE ( 'NONE', #101059, 9.000000000000001776, 3.000000000000000000 ) ;
#82606=AXIS2_PLACEMENT_3D ( 'NONE', #126035, #14404, #102853 ) ;
#82612=DIRECTION ( 'NONE',  ( 0.000000000000000000, -0.000000000000000000, 1.000000000000000000 ) ) ;
#82677=DIRECTION ( 'NONE',  ( -0.000000000000000000, 1.000000000000000000, -0.000000000000000000 ) ) ;
#82686=ADVANCED_FACE ( 'NONE', ( #95012 ), #51550, .T. ) ;
#82702=ORIENTED_EDGE ( 'NONE', *, *, #66430, .F. ) ;
#82736=CARTESIAN_POINT ( 'NONE',  ( -5.226068967585342229, 13.12700265372691000, -24.83981276247084224 ) ) ;
#82792=EDGE_CURVE ( 'NONE', #118671, #32290, #26221, .T. ) ;
#82811=SURFACE_SIDE_STYLE ('',( #93678 ) ) ;
#82818=VERTEX_POINT ( 'NONE', #52243 ) ;
#82840=DIRECTION ( 'NONE',  ( 1.000000000000000000, 3.115803279706882722E-16, 0.000000000000000000 ) ) ;
#82842=DIRECTION ( 'NONE',  ( 0.8571673007021118895, 1.049727191138618079E-16, -0.5150380749100549327 ) ) ;
#82860=( NAMED_UNIT ( * ) SI_UNIT ( $, .STERADIAN. ) SOLID_ANGLE_UNIT ( ) );
#82984=DIRECTION ( 'NONE',  ( -0.000000000000000000, -0.000000000000000000, 1.000000000000000000 ) ) ;
#83003=VECTOR ( 'NONE', #83648, 1000.000000000000000 ) ;
#83004=STYLED_ITEM ( 'NONE', ( #105132 ), #106917 ) ;
#83006=SURFACE_STYLE_FILL_AREA ( #38782 ) ;
#83020=( GEOMETRIC_REPRESENTATION_CONTEXT ( 3 ) GLOBAL_UNCERTAINTY_ASSIGNED_CONTEXT ( ( #134831 ) ) GLOBAL_UNIT_ASSIGNED_CONTEXT ( ( #21217, #10326, #76325 ) ) REPRESENTATION_CONTEXT ( 'NONE', 'WORKASPACE' ) );
#83041=CARTESIAN_POINT ( 'NONE',  ( -10.22679612720078346, 11.22999999113994996, -26.15788125827728905 ) ) ;
#83063=DIRECTION ( 'NONE',  ( 1.000000000000000000, 0.000000000000000000, 0.000000000000000000 ) ) ;
#83068=ORIENTED_EDGE ( 'NONE', *, *, #129034, .F. ) ;
#83112=CARTESIAN_POINT ( 'NONE',  ( -12.70000000000000462, -22.26999999999999247, -39.50000000000000000 ) ) ;
#83155=ORIENTED_EDGE ( 'NONE', *, *, #88359, .F. ) ;
#83159=ORIENTED_EDGE ( 'NONE', *, *, #127583, .F. ) ;
#83188=FILL_AREA_STYLE ('',( #93345 ) ) ;
#83211=AXIS2_PLACEMENT_3D ( 'NONE', #22077, #64184, #43150 ) ;
#83212=DIRECTION ( 'NONE',  ( 0.000000000000000000, 1.000000000000000000, 0.000000000000000000 ) ) ;
#83224=VERTEX_POINT ( 'NONE', #10515 ) ;
#83261=CIRCLE ( 'NONE', #53123, 1.898649999999994842 ) ;
#83270=CARTESIAN_POINT ( 'NONE',  ( -12.20000000000000462, -22.26999999999999247, -40.00000000000000000 ) ) ;
#83395=VECTOR ( 'NONE', #127915, 1000.000000000000000 ) ;
#83396=SURFACE_SIDE_STYLE ('',( #26159 ) ) ;
#83446=EDGE_LOOP ( 'NONE', ( #105411, #7902, #13018, #101429 ) ) ;
#83467=SURFACE_STYLE_FILL_AREA ( #40678 ) ;
#83495=CARTESIAN_POINT ( 'NONE',  ( -13.69211732441125662, 5.972909523125048636, -31.41169802726832927 ) ) ;
#83505=DIRECTION ( 'NONE',  ( -0.000000000000000000, -0.000000000000000000, 1.000000000000000000 ) ) ;
#83566=ORIENTED_EDGE ( 'NONE', *, *, #14352, .F. ) ;
#83648=DIRECTION ( 'NONE',  ( 0.8571673007021110013, 0.000000000000000000, 0.5150380749100563760 ) ) ;
#83702=COLOUR_RGB ( '', 0.72549020, 0.75294118, 0.79215686) ;
#83723=STYLED_ITEM ( 'NONE', ( #45418 ), #55317 ) ;
#83778=AXIS2_PLACEMENT_3D ( 'NONE', #69982, #133084, #80132 ) ;
#83782=CARTESIAN_POINT ( 'NONE',  ( -6.713483559403754519, 11.28174313718248634, -26.16288089844056941 ) ) ;
#83801=FACE_OUTER_BOUND ( 'NONE', #98670, .T. ) ;
#83915=STYLED_ITEM ( 'NONE', ( #94551 ), #143506 ) ;
#83939=CARTESIAN_POINT ( 'NONE',  ( 12.19999999999999574, -40.43000000000000682, 19.06900128115122683 ) ) ;
#83948=FACE_OUTER_BOUND ( 'NONE', #113922, .T. ) ;
#83953=( LENGTH_UNIT ( ) NAMED_UNIT ( * ) SI_UNIT ( .MILLI., .METRE. ) );
#83959=CIRCLE ( 'NONE', #81580, 0.5000000000000000000 ) ;
#83974=AXIS2_PLACEMENT_3D ( 'NONE', #141264, #30372, #40556 ) ;
#83980=EDGE_CURVE ( 'NONE', #132883, #126576, #14342, .T. ) ;
#84021=UNCERTAINTY_MEASURE_WITH_UNIT (LENGTH_MEASURE( 1.000000000000000082E-05 ), #127952, 'distance_accuracy_value', 'NONE');
#84030=FILL_AREA_STYLE ('',( #63694 ) ) ;
#84094=ORIENTED_EDGE ( 'NONE', *, *, #104839, .T. ) ;
#84160=ORIENTED_EDGE ( 'NONE', *, *, #47667, .T. ) ;
#84181=FACE_OUTER_BOUND ( 'NONE', #61375, .T. ) ;
#84205=FACE_OUTER_BOUND ( 'NONE', #12247, .T. ) ;
#84209=VERTEX_POINT ( 'NONE', #23834 ) ;
#84249=DIRECTION ( 'NONE',  ( -0.000000000000000000, 0.000000000000000000, 1.000000000000000000 ) ) ;
#84264=AXIS2_PLACEMENT_3D ( 'NONE', #14253, #12099, #143337 ) ;
#84368=FACE_OUTER_BOUND ( 'NONE', #14631, .T. ) ;
#84380=DIRECTION ( 'NONE',  ( -0.000000000000000000, -1.000000000000000000, -0.000000000000000000 ) ) ;
#84419=DIRECTION ( 'NONE',  ( -0.2248289345038709253, -0.9743982503113675087, 2.708646368993815516E-16 ) ) ;
#84438=ADVANCED_FACE ( 'NONE', ( #126011 ), #26681, .T. ) ;
#84470=DIRECTION ( 'NONE',  ( -1.000000000000000000, 0.000000000000000000, 0.000000000000000000 ) ) ;
#84486=CARTESIAN_POINT ( 'NONE',  ( -12.79760398132481392, 9.635117458823907910, -27.13457238307817576 ) ) ;
#84507=LINE ( 'NONE', #73618, #63353 ) ;
#84570=EDGE_CURVE ( 'NONE', #95348, #97698, #74409, .T. ) ;
#84585=ADVANCED_FACE ( 'NONE', ( #97641 ), #100517, .T. ) ;
#84590=ADVANCED_FACE ( 'NONE', ( #78057 ), #32407, .T. ) ;
#84648=AXIS2_PLACEMENT_3D ( 'NONE', #30875, #141027, #65677 ) ;
#84708=DIRECTION ( 'NONE',  ( -0.000000000000000000, -1.000000000000000000, -0.000000000000000000 ) ) ;
#84747=( GEOMETRIC_REPRESENTATION_CONTEXT ( 3 ) GLOBAL_UNCERTAINTY_ASSIGNED_CONTEXT ( ( #114273 ) ) GLOBAL_UNIT_ASSIGNED_CONTEXT ( ( #50834, #74750, #85579 ) ) REPRESENTATION_CONTEXT ( 'NONE', 'WORKASPACE' ) );
#84766=ADVANCED_FACE ( 'NONE', ( #104606 ), #112113, .T. ) ;
#84787=CARTESIAN_POINT ( 'NONE',  ( 12.69999999999999574, -21.76999999999999247, -40.00000000000000000 ) ) ;
#84794=CYLINDRICAL_SURFACE ( 'NONE', #44589, 2.999999999999999112 ) ;
#84840=CARTESIAN_POINT ( 'NONE',  ( 19.04500000000000881, 3.130000000000007887, -22.35000000000000142 ) ) ;
#84901=CARTESIAN_POINT ( 'NONE',  ( -6.640000000000001457, -34.51840020119762187, 17.97447928118982929 ) ) ;
#84911=ORIENTED_EDGE ( 'NONE', *, *, #36778, .T. ) ;
#84929=FACE_OUTER_BOUND ( 'NONE', #14686, .T. ) ;
#84973=ADVANCED_FACE ( 'NONE', ( #100170 ), #121180, .T. ) ;
#85018=CARTESIAN_POINT ( 'NONE',  ( -19.39744865953807818, 0.5628245286959329130, -30.75764528037382561 ) ) ;
#85037=AXIS2_PLACEMENT_3D ( 'NONE', #64598, #87066, #22483 ) ;
#85041=ADVANCED_FACE ( 'NONE', ( #24727 ), #7302, .F. ) ;
#85065=AXIS2_PLACEMENT_3D ( 'NONE', #85886, #64153, #5446 ) ;
#85080=EDGE_CURVE ( 'NONE', #109962, #119435, #60986, .T. ) ;
#85106=ORIENTED_EDGE ( 'NONE', *, *, #49012, .T. ) ;
#85109=( LENGTH_UNIT ( ) NAMED_UNIT ( * ) SI_UNIT ( .MILLI., .METRE. ) );
#85132=CARTESIAN_POINT ( 'NONE',  ( 7.139999999999956160, -60.26999999999998892, -7.899272885403742173 ) ) ;
#85136=PLANE ( 'NONE',  #101930 ) ;
#85154=LINE ( 'NONE', #129367, #23423 ) ;
#85163=CARTESIAN_POINT ( 'NONE',  ( 9.194147813897108890, 10.01345926878055792, -26.94908941227603094 ) ) ;
#85179=CARTESIAN_POINT ( 'NONE',  ( -31.92499999999997584, -6.270000000000012008, -37.00000000000000000 ) ) ;
#85210=CARTESIAN_POINT ( 'NONE',  ( 7.940000000000001279, -33.26999999999999602, -11.89864999999999462 ) ) ;
#85218=COLOUR_RGB ( '', 0.72549020, 0.75294118, 0.79215686) ;
#85233=CARTESIAN_POINT ( 'NONE',  ( 6.639999999999993463, -34.51840020119762897, 17.97447928118983285 ) ) ;
#85347=CARTESIAN_POINT ( 'NONE',  ( -7.140000000000001457, -35.14999999999999147, -11.72188031596275337 ) ) ;
#85377=DIRECTION ( 'NONE',  ( -0.000000000000000000, -1.000000000000000000, -0.000000000000000000 ) ) ;
#85405=DIRECTION ( 'NONE',  ( 0.000000000000000000, -1.016133275908817741E-16, 1.000000000000000000 ) ) ;
#85409=FILL_AREA_STYLE_COLOUR ( '', #99604 ) ;
#85477=LINE ( 'NONE', #84787, #76791 ) ;
#85481=EDGE_LOOP ( 'NONE', ( #128034, #100116, #8466, #82443 ) ) ;
#85552=COLOUR_RGB ( '', 0.31764706, 0.68627451, 0.89019608) ;
#85554=VECTOR ( 'NONE', #21027, 1000.000000000000000 ) ;
#85579=( NAMED_UNIT ( * ) SI_UNIT ( $, .STERADIAN. ) SOLID_ANGLE_UNIT ( ) );
#85597=CARTESIAN_POINT ( 'NONE',  ( -3.295843663686523595, 12.28244488499750275, -27.01195477951401713 ) ) ;
#85616=( NAMED_UNIT ( * ) PLANE_ANGLE_UNIT ( ) SI_UNIT ( $, .RADIAN. ) );
#85621=VERTEX_POINT ( 'NONE', #85347 ) ;
#85630=VERTEX_POINT ( 'NONE', #41144 ) ;
#85712=CARTESIAN_POINT ( 'NONE',  ( -34.42499999999997584, -21.76999999999999247, -37.00000000000000000 ) ) ;
#85715=EDGE_CURVE ( 'NONE', #2907, #61841, #63646, .T. ) ;
#85753=CARTESIAN_POINT ( 'NONE',  ( -6.640000000000001457, -40.42999999999999261, -40.00000000000000000 ) ) ;
#85815=VECTOR ( 'NONE', #6515, 1000.000000000000114 ) ;
#85856=ORIENTED_EDGE ( 'NONE', *, *, #36173, .T. ) ;
#85860=CARTESIAN_POINT ( 'NONE',  ( 12.19999999999999574, -39.93000000000000682, 19.06900128115122683 ) ) ;
#85884=CARTESIAN_POINT ( 'NONE',  ( 4.286292163570115221, 13.35440448566885685, -24.66944867099426375 ) ) ;
#85886=CARTESIAN_POINT ( 'NONE',  ( 12.69999999999999574, -28.33999999999998565, 13.17925390838734323 ) ) ;
#85888=ORIENTED_EDGE ( 'NONE', *, *, #98465, .T. ) ;
#85943=COLOUR_RGB ( '', 0.08235294, 0.09019608, 0.10196078) ;
#85974=VECTOR ( 'NONE', #55196, 1000.000000000000000 ) ;
#85989=DIRECTION ( 'NONE',  ( 1.000000000000000000, 0.000000000000000000, 0.000000000000000000 ) ) ;
#86090=ADVANCED_FACE ( 'NONE', ( #51155 ), #128702, .T. ) ;
#86094=CARTESIAN_POINT ( 'NONE',  ( -21.60769999999998703, 3.130000000000008331, -22.35000000000000142 ) ) ;
#86098=DIRECTION ( 'NONE',  ( 0.000000000000000000, 0.000000000000000000, 1.000000000000000000 ) ) ;
#86115=( NAMED_UNIT ( * ) SI_UNIT ( $, .STERADIAN. ) SOLID_ANGLE_UNIT ( ) );
#86160=AXIS2_PLACEMENT_3D ( 'NONE', #103401, #49792, #82403 ) ;
#86173=LINE ( 'NONE', #118782, #42225 ) ;
#86193=CARTESIAN_POINT ( 'NONE',  ( 7.139999999999985469, -39.92999999999999972, -40.00000000000000000 ) ) ;
#86207=EDGE_CURVE ( 'NONE', #112438, #89438, #1021, .T. ) ;
#86209=ADVANCED_FACE ( 'NONE', ( #88061 ), #109806, .T. ) ;
#86213=EDGE_CURVE ( 'NONE', #112438, #56577, #9896, .T. ) ;
#86223=SPHERICAL_SURFACE ( 'NONE', #57788, 0.5000000000000000000 ) ;
#86226=DIRECTION ( 'NONE',  ( 3.071323233543530392E-32, -2.242629915582283412E-16, 1.000000000000000000 ) ) ;
#86235=CARTESIAN_POINT ( 'NONE',  ( 19.88523551879106677, -2.838375494165454871, -34.13199556651682798 ) ) ;
#86237=SURFACE_STYLE_USAGE ( .BOTH. , #42021 ) ;
#86263=CIRCLE ( 'NONE', #26031, 2.500000000000002220 ) ;
#86349=CARTESIAN_POINT ( 'NONE',  ( 8.763039537514666577, 10.25773029732260611, -28.68199181715783297 ) ) ;
#86397=EDGE_CURVE ( 'NONE', #99826, #86478, #2443, .T. ) ;
#86400=DIRECTION ( 'NONE',  ( 1.000000000000000000, -0.000000000000000000, -0.000000000000000000 ) ) ;
#86422=AXIS2_PLACEMENT_3D ( 'NONE', #33010, #121393, #118539 ) ;
#86478=VERTEX_POINT ( 'NONE', #5302 ) ;
#86493=SURFACE_STYLE_FILL_AREA ( #55292 ) ;
#86549=FACE_OUTER_BOUND ( 'NONE', #72148, .T. ) ;
#86575=DIRECTION ( 'NONE',  ( -0.000000000000000000, -0.000000000000000000, 1.000000000000000000 ) ) ;
#86583=( NAMED_UNIT ( * ) PLANE_ANGLE_UNIT ( ) SI_UNIT ( $, .RADIAN. ) );
#86598=ORIENTED_EDGE ( 'NONE', *, *, #10111, .F. ) ;
#86630=CARTESIAN_POINT ( 'NONE',  ( 7.528865486064717061, 10.89722440034706885, -26.40697315731449990 ) ) ;
#86661=CYLINDRICAL_SURFACE ( 'NONE', #46874, 34.92999999999999261 ) ;
#86704=DIRECTION ( 'NONE',  ( -3.071323233543530392E-32, 2.242629915582283412E-16, -1.000000000000000000 ) ) ;
#86724=DIRECTION ( 'NONE',  ( -1.000000000000000000, 0.000000000000000000, 0.000000000000000000 ) ) ;
#86790=CIRCLE ( 'NONE', #52108, 2.999999999999999112 ) ;
#86886=( LENGTH_UNIT ( ) NAMED_UNIT ( * ) SI_UNIT ( .MILLI., .METRE. ) );
#86905=CIRCLE ( 'NONE', #17444, 2.999999999999999112 ) ;
#86950=( LENGTH_UNIT ( ) NAMED_UNIT ( * ) SI_UNIT ( .MILLI., .METRE. ) );
#87004=EDGE_CURVE ( 'NONE', #23962, #38919, #125823, .T. ) ;
#87027=COLOUR_RGB ( '', 0.72549020, 0.75294118, 0.79215686) ;
#87040=CARTESIAN_POINT ( 'NONE',  ( 12.19999999999999574, -22.33999999999998565, 3.000000000000000000 ) ) ;
#87051=ADVANCED_FACE ( 'NONE', ( #104627 ), #72043, .T. ) ;
#87066=DIRECTION ( 'NONE',  ( 0.000000000000000000, 0.9647414015272156584, -0.2631995976047526442 ) ) ;
#87069=SURFACE_SIDE_STYLE ('',( #66055 ) ) ;
#87127=COLOUR_RGB ( '', 0.09019608, 0.27058824, 0.51372549) ;
#87129=EDGE_CURVE ( 'NONE', #71803, #118457, #30661, .T. ) ;
#87131=PRESENTATION_STYLE_ASSIGNMENT (( #75547 ) ) ;
#87140=VERTEX_POINT ( 'NONE', #52383 ) ;
#87181=FACE_OUTER_BOUND ( 'NONE', #62031, .T. ) ;
#87206=PLANE ( 'NONE',  #143415 ) ;
#87223=AXIS2_PLACEMENT_3D ( 'NONE', #63920, #18973, #31295 ) ;
#87291=AXIS2_PLACEMENT_3D ( 'NONE', #110277, #123347, #55218 ) ;
#87328=CARTESIAN_POINT ( 'NONE',  ( 6.656140668332151122, 11.28355271028802065, -26.16006910964023291 ) ) ;
#87333=SURFACE_STYLE_FILL_AREA ( #143128 ) ;
#87334=CIRCLE ( 'NONE', #103454, 17.46000000000000085 ) ;
#87355=DIRECTION ( 'NONE',  ( -1.000000000000000000, -3.115803279706882722E-16, -0.000000000000000000 ) ) ;
#87448=FACE_OUTER_BOUND ( 'NONE', #123749, .T. ) ;
#87474=DIRECTION ( 'NONE',  ( -0.000000000000000000, -0.000000000000000000, 1.000000000000000000 ) ) ;
#87493=CARTESIAN_POINT ( 'NONE',  ( -7.940000000000007496, -39.92999999999999261, -10.00000000000000178 ) ) ;
#87526=ORIENTED_EDGE ( 'NONE', *, *, #60227, .F. ) ;
#87613=EDGE_LOOP ( 'NONE', ( #40901, #18608, #82007, #41730, #45228, #36993 ) ) ;
#87614=VERTEX_POINT ( 'NONE', #87702 ) ;
#87702=CARTESIAN_POINT ( 'NONE',  ( -12.70000000000000462, -22.33999999999998565, -0.5000000000000000000 ) ) ;
#87744=ORIENTED_EDGE ( 'NONE', *, *, #6127, .F. ) ;
#87763=CARTESIAN_POINT ( 'NONE',  ( 17.01299345043647193, -0.9444868035624204294, -36.39086428169088094 ) ) ;
#87890=DIRECTION ( 'NONE',  ( 1.000000000000000000, 0.000000000000000000, 0.000000000000000000 ) ) ;
#87900=DIRECTION ( 'NONE',  ( -0.000000000000000000, -1.000000000000000000, -0.000000000000000000 ) ) ;
#87905=EDGE_CURVE ( 'NONE', #131559, #41660, #69521, .T. ) ;
#87938=AXIS2_PLACEMENT_3D ( 'NONE', #87040, #118941, #9431 ) ;
#87939=LINE ( 'NONE', #132181, #122487 ) ;
#87943=AXIS2_PLACEMENT_3D ( 'NONE', #51947, #18550, #139691 ) ;
#88026=AXIS2_PLACEMENT_3D ( 'NONE', #103511, #124578, #136161 ) ;
#88037=CARTESIAN_POINT ( 'NONE',  ( 0.4249279634646616621, 12.59097312579417327, -26.73336350209328671 ) ) ;
#88038=ORIENTED_EDGE ( 'NONE', *, *, #65211, .T. ) ;
#88061=FACE_OUTER_BOUND ( 'NONE', #140511, .T. ) ;
#88095=CIRCLE ( 'NONE', #108850, 2.552699999999994418 ) ;
#88108=FILL_AREA_STYLE ('',( #10516 ) ) ;
#88133=AXIS2_PLACEMENT_3D ( 'NONE', #80965, #3362, #26573 ) ;
#88158=CARTESIAN_POINT ( 'NONE',  ( -34.92499999999997584, 22.27000000000000668, -0.5000000000000004441 ) ) ;
#88162=CARTESIAN_POINT ( 'NONE',  ( -12.20000000000000462, -22.33999999999998565, -0.5000000000000000000 ) ) ;
#88226=VERTEX_POINT ( 'NONE', #138181 ) ;
#88321=SURFACE_SIDE_STYLE ('',( #561 ) ) ;
#88359=EDGE_CURVE ( 'NONE', #48675, #38058, #74361, .T. ) ;
#88382=CARTESIAN_POINT ( 'NONE',  ( 19.93303239253585346, -3.242521478231688015, -35.72961117458194735 ) ) ;
#88429=DIRECTION ( 'NONE',  ( 0.000000000000000000, -0.2555582702174445942, 0.9667936545734397980 ) ) ;
#88445=ORIENTED_EDGE ( 'NONE', *, *, #87129, .T. ) ;
#88447=VECTOR ( 'NONE', #106087, 1000.000000000000000 ) ;
#88491=CARTESIAN_POINT ( 'NONE',  ( 7.174018035375743452, 11.05446268434087465, -28.05475473402666253 ) ) ;
#88529=ORIENTED_EDGE ( 'NONE', *, *, #79504, .F. ) ;
#88538=SHAPE_REPRESENTATION ( '1.1 Sliding Jaw', ( #127880 ), #35272 ) ;
#88571=DIRECTION ( 'NONE',  ( 0.000000000000000000, 1.000000000000000000, 0.000000000000000000 ) ) ;
#88604=DIRECTION ( 'NONE',  ( 0.000000000000000000, 0.000000000000000000, 1.000000000000000000 ) ) ;
#88626=CARTESIAN_POINT ( 'NONE',  ( 14.86712903272168340, 7.883176524338217028, -28.07512293021272143 ) ) ;
#88637=DIRECTION ( 'NONE',  ( 0.000000000000000000, 0.000000000000000000, -1.000000000000000000 ) ) ;
#88659=VERTEX_POINT ( 'NONE', #140661 ) ;
#88691=SURFACE_SIDE_STYLE ('',( #44489 ) ) ;
#88701=CARTESIAN_POINT ( 'NONE',  ( -31.92499999999997584, -21.76999999999999247, -40.00000000000000000 ) ) ;
#88771=CARTESIAN_POINT ( 'NONE',  ( 16.10925740115140314, 1.961328573423360089, -30.40648711071796839 ) ) ;
#88784=FILL_AREA_STYLE_COLOUR ( '', #85218 ) ;
#88791=( NAMED_UNIT ( * ) SI_UNIT ( $, .STERADIAN. ) SOLID_ANGLE_UNIT ( ) );
#88831=EDGE_CURVE ( 'NONE', #78237, #14912, #26661, .T. ) ;
#88889=CARTESIAN_POINT ( 'NONE',  ( -17.01299345042646749, -0.9444868035190714384, -36.39086428169088094 ) ) ;
#88898=EDGE_CURVE ( 'NONE', #66948, #20082, #86905, .T. ) ;
#88973=ORIENTED_EDGE ( 'NONE', *, *, #40258, .T. ) ;
#88986=ORIENTED_EDGE ( 'NONE', *, *, #44980, .T. ) ;
#88989=CARTESIAN_POINT ( 'NONE',  ( 19.75016440660220951, -1.782848796972203331, -32.42302261545219011 ) ) ;
#88991=( BOUNDED_CURVE ( )  B_SPLINE_CURVE ( 3, ( #124809, #58902, #122121, #70484 ),
 .UNSPECIFIED., .F., .F. ) 
 B_SPLINE_CURVE_WITH_KNOTS ( ( 4, 4 ),
 ( 2.276824562219553395E-15, 1.570796326794894338 ),
 .UNSPECIFIED. ) 
 CURVE ( )  GEOMETRIC_REPRESENTATION_ITEM ( )  RATIONAL_B_SPLINE_CURVE ( ( 1.000000000000000000, 0.8047378541243661587, 0.8047378541243661587, 1.000000000000000000 ) ) 
 REPRESENTATION_ITEM ( '' )  );
#89008=CYLINDRICAL_SURFACE ( 'NONE', #16071, 0.5000000000000004441 ) ;
#89036=DIRECTION ( 'NONE',  ( 0.000000000000000000, 0.000000000000000000, -1.000000000000000000 ) ) ;
#89049=VERTEX_POINT ( 'NONE', #5683 ) ;
#89072=CARTESIAN_POINT ( 'NONE',  ( 6.639999999999993463, -34.64999999999999858, -40.00000000000000000 ) ) ;
#89097=ORIENTED_EDGE ( 'NONE', *, *, #120810, .F. ) ;
#89128=EDGE_CURVE ( 'NONE', #83224, #89438, #99988, .T. ) ;
#89143=LINE ( 'NONE', #77567, #11613 ) ;
#89177=CARTESIAN_POINT ( 'NONE',  ( -7.140000000000002345, -35.56014942880460694, -11.72188031596274982 ) ) ;
#89248=CARTESIAN_POINT ( 'NONE',  ( 9.524999999999998579, -4.870000000000013429, -40.00000000000000000 ) ) ;
#89265=ORIENTED_EDGE ( 'NONE', *, *, #136983, .T. ) ;
#89282=( NAMED_UNIT ( * ) SI_UNIT ( $, .STERADIAN. ) SOLID_ANGLE_UNIT ( ) );
#89299=DIRECTION ( 'NONE',  ( 0.000000000000000000, 0.000000000000000000, -1.000000000000000000 ) ) ;
#89320=CARTESIAN_POINT ( 'NONE',  ( 12.14969952407321507, 10.07123342099957064, -26.87533215267990983 ) ) ;
#89325=DIRECTION ( 'NONE',  ( 1.000000000000000000, 3.115803279706882722E-16, 0.000000000000000000 ) ) ;
#89374=( BOUNDED_SURFACE ( )  B_SPLINE_SURFACE ( 3, 2, ( 
 ( #88889, #1802, #23604 ),
 ( #34488, #22855, #56286 ),
 ( #135253, #78705, #91711 ),
 ( #33794, #100465, #122925 ),
 ( #402, #78005, #122184 ),
 ( #46102, #68568, #67121 ),
 ( #90277, #134530, #35229 ),
 ( #24322, #112754, #57696 ),
 ( #124348, #2537, #46846 ),
 ( #91033, #35942, #80160 ),
 ( #113451, #58434, #102613 ),
 ( #3263, #47555, #61287 ) ),
 .UNSPECIFIED., .F., .F., .F. ) 
 B_SPLINE_SURFACE_WITH_KNOTS ( ( 4, 2, 2, 2, 2, 4 ),
 ( 3, 3 ),
 ( 0.000000000000000000, 0.0009975800291739328821, 0.001995160058347865764, 0.002493950072934832205, 0.002992740087521798646, 0.003990320116695731528 ),
 ( 0.000000000000000000, 1.000000000000000000 ),
 .UNSPECIFIED. ) 
 GEOMETRIC_REPRESENTATION_ITEM ( )  RATIONAL_B_SPLINE_SURFACE ( (
 ( 1.000000000000000000, 0.7825691453495835503, 1.000000000000000000),
 ( 1.000000000000000000, 0.7825473240981194456, 1.000000000000000000),
 ( 1.000000000000000000, 0.7821547027292599097, 1.000000000000000000),
 ( 1.000000000000000000, 0.7799370077755589659, 1.000000000000000000),
 ( 1.000000000000000000, 0.7781753367904327146, 1.000000000000000000),
 ( 1.000000000000000000, 0.7735157641301041442, 1.000000000000000000),
 ( 1.000000000000000000, 0.7716557628207030284, 1.000000000000000000),
 ( 1.000000000000000000, 0.7671421219664820157, 1.000000000000000000),
 ( 1.000000000000000000, 0.7644786082298313801, 1.000000000000000000),
 ( 1.000000000000000000, 0.7550095275972034115, 1.000000000000000000),
 ( 1.000000000000000000, 0.7469941267412624208, 1.000000000000000000),
 ( 1.000000000000000000, 0.7366656399173064917, 1.000000000000000000) ) ) 
 REPRESENTATION_ITEM ( '' )  SURFACE ( )  );
#89405=TOROIDAL_SURFACE ( 'NONE', #80127, 6.000000000000000000, 3.000000000000000000 ) ;
#89438=VERTEX_POINT ( 'NONE', #83112 ) ;
#89451=STYLED_ITEM ( 'NONE', ( #112094 ), #106085 ) ;
#89454=CARTESIAN_POINT ( 'NONE',  ( 14.64989824621740233, 4.671147552932954916, -29.50326184817846098 ) ) ;
#89457=EDGE_CURVE ( 'NONE', #30341, #27902, #36054, .T. ) ;
#89485=DIRECTION ( 'NONE',  ( 1.000000000000000000, 3.115803279706882722E-16, -0.000000000000000000 ) ) ;
#89495=ORIENTED_EDGE ( 'NONE', *, *, #136290, .T. ) ;
#89524=FACE_OUTER_BOUND ( 'NONE', #59720, .T. ) ;
#89546=CYLINDRICAL_SURFACE ( 'NONE', #77713, 0.5000000000000004441 ) ;
#89558=( GEOMETRIC_REPRESENTATION_CONTEXT ( 3 ) GLOBAL_UNCERTAINTY_ASSIGNED_CONTEXT ( ( #33050 ) ) GLOBAL_UNIT_ASSIGNED_CONTEXT ( ( #33490, #121166, #35637 ) ) REPRESENTATION_CONTEXT ( 'NONE', 'WORKASPACE' ) );
#89560=VERTEX_POINT ( 'NONE', #85233 ) ;
#89633=CARTESIAN_POINT ( 'NONE',  ( -12.20000000000000284, -25.47159979880235881, 14.98806839329795260 ) ) ;
#89664=UNCERTAINTY_MEASURE_WITH_UNIT (LENGTH_MEASURE( 1.000000000000000082E-05 ), #57436, 'distance_accuracy_value', 'NONE');
#89677=CARTESIAN_POINT ( 'NONE',  ( 17.49081203853565825, -2.909728817766679132, -34.30943779066389254 ) ) ;
#89904=DIRECTION ( 'NONE',  ( 1.248002500702738701E-15, 1.000000000000000000, -0.000000000000000000 ) ) ;
#89956=LINE ( 'NONE', #66802, #53826 ) ;
#89974=FILL_AREA_STYLE_COLOUR ( '', #118458 ) ;
#90023=SURFACE_STYLE_FILL_AREA ( #67607 ) ;
#90078=CARTESIAN_POINT ( 'NONE',  ( 31.92500000000002203, -21.76999999999999247, -39.50000000000000000 ) ) ;
#90083=( NAMED_UNIT ( * ) SI_UNIT ( $, .STERADIAN. ) SOLID_ANGLE_UNIT ( ) );
#90113=CARTESIAN_POINT ( 'NONE',  ( 32.75030053044775968, 22.27000000000001023, -14.49242101875391064 ) ) ;
#90130=ORIENTED_EDGE ( 'NONE', *, *, #55115, .F. ) ;
#90147=( LENGTH_UNIT ( ) NAMED_UNIT ( * ) SI_UNIT ( .MILLI., .METRE. ) );
#90232=( LENGTH_UNIT ( ) NAMED_UNIT ( * ) SI_UNIT ( .MILLI., .METRE. ) );
#90275=ORIENTED_EDGE ( 'NONE', *, *, #31078, .F. ) ;
#90277=CARTESIAN_POINT ( 'NONE',  ( -16.82844983938008454, -0.2153006699122482492, -34.28771444467989937 ) ) ;
#90396=STYLED_ITEM ( 'NONE', ( #25253 ), #114939 ) ;
#90454=ORIENTED_EDGE ( 'NONE', *, *, #50202, .F. ) ;
#90524=DIRECTION ( 'NONE',  ( 1.369518533665900312E-16, -1.000000000000000000, 0.000000000000000000 ) ) ;
#90528=AXIS2_PLACEMENT_3D ( 'NONE', #140744, #141479, #142213 ) ;
#90574=B_SPLINE_CURVE_WITH_KNOTS ( 'NONE', 3,
 ( #132677, #33368, #121736, #22415, #66677, #11533, #55812, #100015, #123390, #57410 ),
 .UNSPECIFIED., .F., .F.,
 ( 4, 2, 2, 2, 4 ),
 ( 0.000000000000000000, 0.0009358269096809158352, 0.001871653819361831670, 0.002807480729042747397, 0.003743307638723663341 ),
 .UNSPECIFIED. ) ;
#90578=CARTESIAN_POINT ( 'NONE',  ( 7.140000000000044089, -1.036479131253094653E-14, -40.00000000000000000 ) ) ;
#90609=CIRCLE ( 'NONE', #2608, 3.500000000000000444 ) ;
#90654=CARTESIAN_POINT ( 'NONE',  ( 0.000000000000000000, -35.14999999999999147, -40.00000000000000000 ) ) ;
#90660=STYLED_ITEM ( 'NONE', ( #818 ), #84973 ) ;
#90709=PRESENTATION_STYLE_ASSIGNMENT (( #126860 ) ) ;
#90712=COLOUR_RGB ( '', 0.40784314, 0.44705882, 0.49803922) ;
#90715=SURFACE_SIDE_STYLE ('',( #46529 ) ) ;
#90722=AXIS2_PLACEMENT_3D ( 'NONE', #17277, #85377, #141946 ) ;
#90779=LINE ( 'NONE', #80613, #132411 ) ;
#90838=LINE ( 'NONE', #135067, #135353 ) ;
#90884=EDGE_LOOP ( 'NONE', ( #13758, #104164, #136099, #7546, #97663, #127248, #135390 ) ) ;
#90894=FILL_AREA_STYLE_COLOUR ( '', #41227 ) ;
#90963=ORIENTED_EDGE ( 'NONE', *, *, #62674, .T. ) ;
#91005=FACE_OUTER_BOUND ( 'NONE', #62534, .T. ) ;
#91033=CARTESIAN_POINT ( 'NONE',  ( -16.63174071259636833, 0.4494130005253863525, -33.70036845157063254 ) ) ;
#91037=( NAMED_UNIT ( * ) SI_UNIT ( $, .STERADIAN. ) SOLID_ANGLE_UNIT ( ) );
#91052=ADVANCED_FACE ( 'NONE', ( #95977 ), #74985, .T. ) ;
#91055=ORIENTED_EDGE ( 'NONE', *, *, #51734, .T. ) ;
#91102=VERTEX_POINT ( 'NONE', #44505 ) ;
#91109=ADVANCED_FACE ( 'NONE', ( #13239 ), #121304, .T. ) ;
#91121=ORIENTED_EDGE ( 'NONE', *, *, #15831, .F. ) ;
#91150=UNCERTAINTY_MEASURE_WITH_UNIT (LENGTH_MEASURE( 1.000000000000000082E-05 ), #71137, 'distance_accuracy_value', 'NONE');
#91195=( NAMED_UNIT ( * ) SI_UNIT ( $, .STERADIAN. ) SOLID_ANGLE_UNIT ( ) );
#91246=DIRECTION ( 'NONE',  ( 0.000000000000000000, 0.000000000000000000, -1.000000000000000000 ) ) ;
#91388=CIRCLE ( 'NONE', #93658, 0.5000000000000004441 ) ;
#91409=ORIENTED_EDGE ( 'NONE', *, *, #106755, .F. ) ;
#91472=CARTESIAN_POINT ( 'NONE',  ( 4.161307151687957173, 13.37712895942531688, -24.65215201657544952 ) ) ;
#91532=ORIENTED_EDGE ( 'NONE', *, *, #20291, .T. ) ;
#91537=SURFACE_STYLE_FILL_AREA ( #102432 ) ;
#91591=DIRECTION ( 'NONE',  ( -0.000000000000000000, -1.000000000000000000, -0.000000000000000000 ) ) ;
#91615=LINE ( 'NONE', #137270, #42287 ) ;
#91625=DIRECTION ( 'NONE',  ( 0.000000000000000000, -0.5150380749100594846, -0.8571673007021091140 ) ) ;
#91643=AXIS2_PLACEMENT_3D ( 'NONE', #131482, #119158, #61959 ) ;
#91711=CARTESIAN_POINT ( 'NONE',  ( -19.92362232443690218, -3.158997490844367206, -35.05992480806695255 ) ) ;
#91715=CARTESIAN_POINT ( 'NONE',  ( -34.92499999999997584, 0.000000000000000000, -40.00000000000000000 ) ) ;
#91813=CARTESIAN_POINT ( 'NONE',  ( 16.45742106731621490, 0.9613713492673634509, -33.49048331797055766 ) ) ;
#91863=PRESENTATION_STYLE_ASSIGNMENT (( #70860 ) ) ;
#91928=ORIENTED_EDGE ( 'NONE', *, *, #5336, .T. ) ;
#92036=ORIENTED_EDGE ( 'NONE', *, *, #107060, .F. ) ;
#92041=CARTESIAN_POINT ( 'NONE',  ( -4.983273985306034929E-14, -39.92999999999999261, -40.00000000000000000 ) ) ;
#92081=LINE ( 'NONE', #101535, #124865 ) ;
#92097=EDGE_LOOP ( 'NONE', ( #72575, #62386, #95514, #57245 ) ) ;
#92115=ADVANCED_FACE ( 'NONE', ( #60568, #104741 ), #93862, .F. ) ;
#92141=FILL_AREA_STYLE ('',( #105172 ) ) ;
#92218=CYLINDRICAL_SURFACE ( 'NONE', #104577, 2.552699999999994418 ) ;
#92223=ADVANCED_FACE ( 'NONE', ( #43778 ), #140929, .T. ) ;
#92240=CARTESIAN_POINT ( 'NONE',  ( 34.79316404164333676, 22.27000000000000668, -10.13466756456404916 ) ) ;
#92259=CARTESIAN_POINT ( 'NONE',  ( -7.140000000000001457, -35.13237070076360169, 17.62370837922860289 ) ) ;
#92280=DIRECTION ( 'NONE',  ( -1.000000000000000000, 0.000000000000000000, 0.000000000000000000 ) ) ;
#92337=ORIENTED_EDGE ( 'NONE', *, *, #42043, .T. ) ;
#92341=VERTEX_POINT ( 'NONE', #24869 ) ;
#92369=ORIENTED_EDGE ( 'NONE', *, *, #86213, .F. ) ;
#92457=CARTESIAN_POINT ( 'NONE',  ( -13.68197150847072230, 5.985828926257079630, -31.40491832948329787 ) ) ;
#92463=VECTOR ( 'NONE', #33899, 1000.000000000000000 ) ;
#92476=EDGE_CURVE ( 'NONE', #69904, #13983, #81433, .T. ) ;
#92546=ORIENTED_EDGE ( 'NONE', *, *, #437, .T. ) ;
#92630=VERTEX_POINT ( 'NONE', #110963 ) ;
#92636=CARTESIAN_POINT ( 'NONE',  ( -7.940000000000001279, -60.26999999999998892, -10.00000000000000178 ) ) ;
#92690=ORIENTED_EDGE ( 'NONE', *, *, #6261, .F. ) ;
#92723=VERTEX_POINT ( 'NONE', #89248 ) ;
#92758=AXIS2_PLACEMENT_3D ( 'NONE', #126460, #104719, #27156 ) ;
#92861=DIRECTION ( 'NONE',  ( -1.451651444332056451E-15, -1.000000000000000000, 0.000000000000000000 ) ) ;
#92867=STYLED_ITEM ( 'NONE', ( #103041 ), #72019 ) ;
#92879=CARTESIAN_POINT ( 'NONE',  ( -15.90492180865371274, 6.766090994904859102, -28.60278292646719933 ) ) ;
#92895=DIRECTION ( 'NONE',  ( 1.000000000000000000, -0.000000000000000000, -0.000000000000000000 ) ) ;
#92922=DIRECTION ( 'NONE',  ( -1.000000000000000000, 0.000000000000000000, 0.000000000000000000 ) ) ;
#92959=EDGE_CURVE ( 'NONE', #15191, #48074, #51464, .T. ) ;
#92975=EDGE_LOOP ( 'NONE', ( #106420, #132525, #101630, #18059 ) ) ;
#93008=AXIS2_PLACEMENT_3D ( 'NONE', #91715, #136639, #102618 ) ;
#93015=ORIENTED_EDGE ( 'NONE', *, *, #12180, .T. ) ;
#93031=DIRECTION ( 'NONE',  ( 1.000000000000000000, 0.000000000000000000, 0.000000000000000000 ) ) ;
#93055=CARTESIAN_POINT ( 'NONE',  ( 12.69999999999999574, 0.000000000000000000, -39.50000000000000000 ) ) ;
#93081=STYLED_ITEM ( 'NONE', ( #3786 ), #15692 ) ;
#93097=DIRECTION ( 'NONE',  ( 0.000000000000000000, -1.000000000000000000, 0.000000000000000000 ) ) ;
#93109=CARTESIAN_POINT ( 'NONE',  ( 34.92500000000001847, -7.729999999999995097, 3.180000000000000160 ) ) ;
#93112=AXIS2_PLACEMENT_3D ( 'NONE', #53414, #130996, #30974 ) ;
#93194=( NAMED_UNIT ( * ) SI_UNIT ( $, .STERADIAN. ) SOLID_ANGLE_UNIT ( ) );
#93203=AXIS2_PLACEMENT_3D ( 'NONE', #22719, #37761, #25413 ) ;
#93243=ADVANCED_FACE ( 'NONE', ( #128664 ), #38855, .T. ) ;
#93301=DIRECTION ( 'NONE',  ( 0.000000000000000000, 0.000000000000000000, -1.000000000000000000 ) ) ;
#93311=CARTESIAN_POINT ( 'NONE',  ( 7.939999999999994174, -39.93000000000000682, -7.752100000000004876 ) ) ;
#93316=CIRCLE ( 'NONE', #128005, 0.5000000000000004441 ) ;
#93345=FILL_AREA_STYLE_COLOUR ( '', #142304 ) ;
#93352=AXIS2_PLACEMENT_3D ( 'NONE', #85179, #106937, #29372 ) ;
#93406=ADVANCED_FACE ( 'NONE', ( #34349 ), #36488, .F. ) ;
#93408=DIRECTION ( 'NONE',  ( -1.000000000000000000, -1.369518533665900312E-16, 0.000000000000000000 ) ) ;
#93437=EDGE_CURVE ( 'NONE', #28467, #84209, #20361, .T. ) ;
#93482=( GEOMETRIC_REPRESENTATION_CONTEXT ( 3 ) GLOBAL_UNCERTAINTY_ASSIGNED_CONTEXT ( ( #23146 ) ) GLOBAL_UNIT_ASSIGNED_CONTEXT ( ( #105479, #38120, #93194 ) ) REPRESENTATION_CONTEXT ( 'NONE', 'WORKASPACE' ) );
#93556=LINE ( 'NONE', #17405, #77169 ) ;
#93582=EDGE_LOOP ( 'NONE', ( #31744, #112019, #84911, #61201, #21929, #7590, #81676 ) ) ;
#93607=ORIENTED_EDGE ( 'NONE', *, *, #12180, .F. ) ;
#93619=CARTESIAN_POINT ( 'NONE',  ( 12.69999999999999574, -22.26999999999999247, -40.00000000000000000 ) ) ;
#93648=CARTESIAN_POINT ( 'NONE',  ( -6.771599798802371950, -34.64999999999999147, 17.99210858042621908 ) ) ;
#93658=AXIS2_PLACEMENT_3D ( 'NONE', #101590, #100885, #33525 ) ;
#93668=DIRECTION ( 'NONE',  ( -1.000000000000000000, 3.654646145370261567E-15, 0.000000000000000000 ) ) ;
#93678=SURFACE_STYLE_FILL_AREA ( #40040 ) ;
#93693=EDGE_LOOP ( 'NONE', ( #35456, #49968, #18698, #108105 ) ) ;
#93708=ADVANCED_FACE ( 'NONE', ( #142246 ), #9531, .F. ) ;
#93737=DIRECTION ( 'NONE',  ( -0.000000000000000000, -1.000000000000000000, -0.000000000000000000 ) ) ;
#93738=ORIENTED_EDGE ( 'NONE', *, *, #48379, .F. ) ;
#93813=CARTESIAN_POINT ( 'NONE',  ( 7.139999999999955271, -35.56014942880460694, -8.278119684037269721 ) ) ;
#93822=CARTESIAN_POINT ( 'NONE',  ( -34.92499999999999005, -3.270000000000013340, -37.00000000000000000 ) ) ;
#93827=ORIENTED_EDGE ( 'NONE', *, *, #13442, .T. ) ;
#93845=VECTOR ( 'NONE', #78367, 1000.000000000000114 ) ;
#93862=PLANE ( 'NONE',  #68793 ) ;
#93899=AXIS2_PLACEMENT_3D ( 'NONE', #121294, #109709, #55348 ) ;
#93901=CARTESIAN_POINT ( 'NONE',  ( -10.36538675573420676, 9.201169882002593781, -27.40968550208418364 ) ) ;
#93961=CARTESIAN_POINT ( 'NONE',  ( -7.140000000000002345, -35.56014942880460694, -11.72188031596274982 ) ) ;
#93998=LINE ( 'NONE', #27310, #114258 ) ;
#94090=LINE ( 'NONE', #50605, #74159 ) ;
#94112=DIRECTION ( 'NONE',  ( -1.000000000000000000, 0.000000000000000000, 0.000000000000000000 ) ) ;
#94250=( LENGTH_UNIT ( ) NAMED_UNIT ( * ) SI_UNIT ( .MILLI., .METRE. ) );
#94279=EDGE_CURVE ( 'NONE', #9868, #6439, #75946, .T. ) ;
#94291=SURFACE_STYLE_FILL_AREA ( #92141 ) ;
#94298=DIRECTION ( 'NONE',  ( 1.000000000000000000, -0.000000000000000000, 0.000000000000000000 ) ) ;
#94330=ORIENTED_EDGE ( 'NONE', *, *, #129833, .F. ) ;
#94345=SURFACE_STYLE_FILL_AREA ( #29097 ) ;
#94384=DIRECTION ( 'NONE',  ( 0.000000000000000000, 0.000000000000000000, -1.000000000000000000 ) ) ;
#94417=( NAMED_UNIT ( * ) PLANE_ANGLE_UNIT ( ) SI_UNIT ( $, .RADIAN. ) );
#94482=DIRECTION ( 'NONE',  ( 3.166071393695993333E-32, -1.016133275908817741E-16, 1.000000000000000000 ) ) ;
#94509=ORIENTED_EDGE ( 'NONE', *, *, #17255, .F. ) ;
#94531=CARTESIAN_POINT ( 'NONE',  ( -16.84537971347776875, -0.2749361969536389116, -34.34141757107727244 ) ) ;
#94551=PRESENTATION_STYLE_ASSIGNMENT (( #39497 ) ) ;
#94562=MECHANICAL_DESIGN_GEOMETRIC_PRESENTATION_REPRESENTATION('',(#83004),#62209);
#94582=AXIS2_PLACEMENT_3D ( 'NONE', #142998, #87900, #88637 ) ;
#94606=CARTESIAN_POINT ( 'NONE',  ( -7.578096315150903095, 10.89383722895850504, -26.41284878744174947 ) ) ;
#94651=VECTOR ( 'NONE', #70830, 999.9999999999998863 ) ;
#94712=CARTESIAN_POINT ( 'NONE',  ( 16.49230000000001084, 3.130000000000008331, -2.396719511207313368E-16 ) ) ;
#94768=CIRCLE ( 'NONE', #22933, 1.898649999999994842 ) ;
#94769=EDGE_CURVE ( 'NONE', #41660, #51304, #76516, .T. ) ;
#94789=DIRECTION ( 'NONE',  ( -1.000000000000000000, 0.000000000000000000, -0.000000000000000000 ) ) ;
#94824=( LENGTH_UNIT ( ) NAMED_UNIT ( * ) SI_UNIT ( .MILLI., .METRE. ) );
#94853=( NAMED_UNIT ( * ) SI_UNIT ( $, .STERADIAN. ) SOLID_ANGLE_UNIT ( ) );
#94870=EDGE_CURVE ( 'NONE', #31365, #71785, #88991, .T. ) ;
#94897=DIRECTION ( 'NONE',  ( 0.000000000000000000, 0.000000000000000000, 1.000000000000000000 ) ) ;
#94898=EDGE_CURVE ( 'NONE', #71183, #9868, #9045, .T. ) ;
#94940=EDGE_CURVE ( 'NONE', #61882, #89049, #47992, .T. ) ;
#94976=DIRECTION ( 'NONE',  ( 3.469446951953611033E-15, -1.000000000000000000, -6.938893903907222067E-15 ) ) ;
#95012=FACE_OUTER_BOUND ( 'NONE', #45321, .T. ) ;
#95027=EDGE_CURVE ( 'NONE', #116824, #34379, #29992, .T. ) ;
#95048=DIRECTION ( 'NONE',  ( 1.000000000000000000, 0.000000000000000000, 0.000000000000000000 ) ) ;
#95080=FILL_AREA_STYLE_COLOUR ( '', #17556 ) ;
#95112=CARTESIAN_POINT ( 'NONE',  ( 31.92500000000001492, 2.730000000000007088, -36.39086428169088094 ) ) ;
#95137=FILL_AREA_STYLE_COLOUR ( '', #122677 ) ;
#95173=( GEOMETRIC_REPRESENTATION_CONTEXT ( 3 ) GLOBAL_UNCERTAINTY_ASSIGNED_CONTEXT ( ( #15491 ) ) GLOBAL_UNIT_ASSIGNED_CONTEXT ( ( #83953, #49887, #117227 ) ) REPRESENTATION_CONTEXT ( 'NONE', 'WORKASPACE' ) );
#95216=EDGE_CURVE ( 'NONE', #13538, #124237, #108728, .T. ) ;
#95231=ORIENTED_EDGE ( 'NONE', *, *, #62219, .T. ) ;
#95272=DIRECTION ( 'NONE',  ( 0.000000000000000000, 0.000000000000000000, -1.000000000000000000 ) ) ;
#95348=VERTEX_POINT ( 'NONE', #67431 ) ;
#95369=ORIENTED_EDGE ( 'NONE', *, *, #36173, .F. ) ;
#95373=CARTESIAN_POINT ( 'NONE',  ( -12.20000000000000284, -40.42999999999999261, -39.50000000000000000 ) ) ;
#95388=CYLINDRICAL_SURFACE ( 'NONE', #63864, 0.5000000000000004441 ) ;
#95398=ORIENTED_EDGE ( 'NONE', *, *, #74309, .F. ) ;
#95401=COLOUR_RGB ( '', 0.40784314, 0.44705882, 0.49803922) ;
#95409=CARTESIAN_POINT ( 'NONE',  ( 12.69999999999999574, -35.15000000000000568, -39.50000000000000000 ) ) ;
#95456=( GEOMETRIC_REPRESENTATION_CONTEXT ( 3 ) GLOBAL_UNCERTAINTY_ASSIGNED_CONTEXT ( ( #77928 ) ) GLOBAL_UNIT_ASSIGNED_CONTEXT ( ( #7896, #63051, #106480 ) ) REPRESENTATION_CONTEXT ( 'NONE', 'WORKASPACE' ) );
#95467=ORIENTED_EDGE ( 'NONE', *, *, #46465, .F. ) ;
#95472=DIRECTION ( 'NONE',  ( 0.000000000000000000, 0.000000000000000000, 1.000000000000000000 ) ) ;
#95514=ORIENTED_EDGE ( 'NONE', *, *, #18717, .T. ) ;
#95561=FILL_AREA_STYLE ('',( #141961 ) ) ;
#95622=EDGE_LOOP ( 'NONE', ( #116963, #41788, #132461, #116201, #129474, #47091, #110474, #43912, #16228 ) ) ;
#95629=ORIENTED_EDGE ( 'NONE', *, *, #22518, .F. ) ;
#95634=DIRECTION ( 'NONE',  ( 0.000000000000000000, 1.000000000000000000, 0.000000000000000000 ) ) ;
#95672=DIRECTION ( 'NONE',  ( -0.000000000000000000, -0.000000000000000000, -1.000000000000000000 ) ) ;
#95680=AXIS2_PLACEMENT_3D ( 'NONE', #103193, #4530, #50266 ) ;
#95707=DIRECTION ( 'NONE',  ( 1.000000000000000000, 0.000000000000000000, 0.000000000000000000 ) ) ;
#95716=( GEOMETRIC_REPRESENTATION_CONTEXT ( 3 ) GLOBAL_UNCERTAINTY_ASSIGNED_CONTEXT ( ( #72442 ) ) GLOBAL_UNIT_ASSIGNED_CONTEXT ( ( #34641, #12855, #136082 ) ) REPRESENTATION_CONTEXT ( 'NONE', 'WORKASPACE' ) );
#95739=ORIENTED_EDGE ( 'NONE', *, *, #19743, .F. ) ;
#95743=MECHANICAL_DESIGN_GEOMETRIC_PRESENTATION_REPRESENTATION('',(#14724),#93482);
#95802=( LENGTH_UNIT ( ) NAMED_UNIT ( * ) SI_UNIT ( .MILLI., .METRE. ) );
#95834=DIRECTION ( 'NONE',  ( -0.000000000000000000, -1.000000000000000000, -0.000000000000000000 ) ) ;
#95843=EDGE_CURVE ( 'NONE', #77610, #44308, #15660, .T. ) ;
#95858=SURFACE_SIDE_STYLE ('',( #48808 ) ) ;
#95890=EDGE_CURVE ( 'NONE', #72919, #117423, #134002, .T. ) ;
#95896=CARTESIAN_POINT ( 'NONE',  ( -19.28515664589289003, 1.196650378695325090, -30.59010235425025215 ) ) ;
#95900=CARTESIAN_POINT ( 'NONE',  ( 12.19999999999999574, -40.29840020119763011, 19.55137198191483350 ) ) ;
#95961=EDGE_LOOP ( 'NONE', ( #4493, #75211, #115765, #18888 ) ) ;
#95977=FACE_OUTER_BOUND ( 'NONE', #102255, .T. ) ;
#95986=DIRECTION ( 'NONE',  ( -1.000000000000000000, 0.000000000000000000, 0.000000000000000000 ) ) ;
#96011=EDGE_LOOP ( 'NONE', ( #75704, #61003, #13262, #90275, #12529, #30260, #65386, #42866, #71835 ) ) ;
#96039=CARTESIAN_POINT ( 'NONE',  ( -3.697064227771988509, 12.20036213366778099, -27.08507981779950313 ) ) ;
#96044=DIRECTION ( 'NONE',  ( 0.000000000000000000, 0.000000000000000000, -1.000000000000000000 ) ) ;
#96070=( LENGTH_UNIT ( ) NAMED_UNIT ( * ) SI_UNIT ( .MILLI., .METRE. ) );
#96118=EDGE_CURVE ( 'NONE', #128588, #128930, #25220, .T. ) ;
#96146=FILL_AREA_STYLE ('',( #54826 ) ) ;
#96164=ORIENTED_EDGE ( 'NONE', *, *, #104839, .F. ) ;
#96257=SURFACE_STYLE_USAGE ( .BOTH. , #5689 ) ;
#96263=ORIENTED_EDGE ( 'NONE', *, *, #127006, .T. ) ;
#96271=CARTESIAN_POINT ( 'NONE',  ( -12.70000000000000462, -25.83999999999998565, 2.999999999999999112 ) ) ;
#96276=EDGE_CURVE ( 'NONE', #18833, #78237, #121201, .T. ) ;
#96315=PRESENTATION_STYLE_ASSIGNMENT (( #129685 ) ) ;
#96346=ORIENTED_EDGE ( 'NONE', *, *, #112441, .T. ) ;
#96353=FILL_AREA_STYLE_COLOUR ( '', #46089 ) ;
#96432=DIRECTION ( 'NONE',  ( -3.166071393695993333E-32, 1.016133275908817741E-16, -1.000000000000000000 ) ) ;
#96437=ORIENTED_EDGE ( 'NONE', *, *, #54934, .F. ) ;
#96452=CARTESIAN_POINT ( 'NONE',  ( 10.93876867942899622, 8.767031578203539510, -29.74760889984009182 ) ) ;
#96500=ORIENTED_EDGE ( 'NONE', *, *, #67696, .T. ) ;
#96690=DIRECTION ( 'NONE',  ( 0.000000000000000000, -1.000000000000000000, 0.000000000000000000 ) ) ;
#96700=EDGE_CURVE ( 'NONE', #89049, #143240, #47351, .T. ) ;
#96710=ORIENTED_EDGE ( 'NONE', *, *, #45748, .F. ) ;
#96723=CARTESIAN_POINT ( 'NONE',  ( 2.438206507620173102, 12.42651081890557307, -25.38545720235088154 ) ) ;
#96737=CARTESIAN_POINT ( 'NONE',  ( -7.940000000000001279, -33.26999999999999602, -11.89864999999999462 ) ) ;
#96773=PRESENTATION_STYLE_ASSIGNMENT (( #132347 ) ) ;
#96844=VERTEX_POINT ( 'NONE', #102756 ) ;
#96905=AXIS2_PLACEMENT_3D ( 'NONE', #127317, #28019, #37480 ) ;
#96919=EDGE_CURVE ( 'NONE', #97698, #88226, #64776, .T. ) ;
#96953=UNCERTAINTY_MEASURE_WITH_UNIT (LENGTH_MEASURE( 1.000000000000000082E-05 ), #67876, 'distance_accuracy_value', 'NONE');
#96972=CARTESIAN_POINT ( 'NONE',  ( -12.20000000000000462, -25.33999999999998565, 2.999999999999999112 ) ) ;
#96990=FACE_OUTER_BOUND ( 'NONE', #57557, .T. ) ;
#97015=STYLED_ITEM ( 'NONE', ( #112691 ), #58768 ) ;
#97025=LINE ( 'NONE', #107222, #138228 ) ;
#97048=CARTESIAN_POINT ( 'NONE',  ( -55.65468426143998215, -28.33999999999998565, 13.17925390838734323 ) ) ;
#97088=SURFACE_STYLE_USAGE ( .BOTH. , #64507 ) ;
#97129=FACE_OUTER_BOUND ( 'NONE', #128742, .T. ) ;
#97147=EDGE_LOOP ( 'NONE', ( #207, #54393, #70391, #116718, #87744 ) ) ;
#97163=CARTESIAN_POINT ( 'NONE',  ( 11.60152521092712341, 8.206876333263409151, -30.11676755377419568 ) ) ;
#97202=DIRECTION ( 'NONE',  ( -1.000000000000000000, 0.000000000000000000, 0.000000000000000000 ) ) ;
#97245=DIRECTION ( 'NONE',  ( 0.000000000000000000, 0.000000000000000000, 1.000000000000000000 ) ) ;
#97287=ORIENTED_EDGE ( 'NONE', *, *, #52281, .T. ) ;
#97358=VERTEX_POINT ( 'NONE', #125770 ) ;
#97375=DIRECTION ( 'NONE',  ( 0.000000000000000000, 0.000000000000000000, 1.000000000000000000 ) ) ;
#97431=VERTEX_POINT ( 'NONE', #38745 ) ;
#97457=CARTESIAN_POINT ( 'NONE',  ( -34.92499999999997584, -7.730000000000015525, 3.180000000000000160 ) ) ;
#97461=CARTESIAN_POINT ( 'NONE',  ( 5.847033781869541258, 11.58818063635165885, -27.61414687898571430 ) ) ;
#97500=EDGE_CURVE ( 'NONE', #72776, #126104, #16994, .T. ) ;
#97596=VECTOR ( 'NONE', #60515, 1000.000000000000000 ) ;
#97620=STYLED_ITEM ( 'NONE', ( #132358 ), #65904 ) ;
#97635=COLOUR_RGB ( '', 0.66274510, 0.83137255, 0.94901961) ;
#97641=FACE_OUTER_BOUND ( 'NONE', #2342, .T. ) ;
#97663=ORIENTED_EDGE ( 'NONE', *, *, #112253, .T. ) ;
#97673=AXIS2_PLACEMENT_3D ( 'NONE', #60403, #124204, #37193 ) ;
#97692=( LENGTH_UNIT ( ) NAMED_UNIT ( * ) SI_UNIT ( .MILLI., .METRE. ) );
#97698=VERTEX_POINT ( 'NONE', #101682 ) ;
#97751=DIRECTION ( 'NONE',  ( 1.248002500702736137E-15, 1.000000000000000000, 0.000000000000000000 ) ) ;
#97875=AXIS2_PLACEMENT_3D ( 'NONE', #44600, #45302, #22064 ) ;
#97895=DIRECTION ( 'NONE',  ( 3.115803279706882722E-16, -1.000000000000000000, 0.000000000000000000 ) ) ;
#97927=CARTESIAN_POINT ( 'NONE',  ( 5.913250154378581591, 11.56455435889447436, -27.63405961019482149 ) ) ;
#97946=PLANE ( 'NONE',  #30374 ) ;
#97964=LINE ( 'NONE', #76952, #3861 ) ;
#98051=EDGE_CURVE ( 'NONE', #79346, #98685, #52956, .T. ) ;
#98106=ORIENTED_EDGE ( 'NONE', *, *, #75237, .F. ) ;
#98111=COLOUR_RGB ( '', 0.31764706, 0.68627451, 0.89019608) ;
#98120=ORIENTED_EDGE ( 'NONE', *, *, #32298, .T. ) ;
#98137=VECTOR ( 'NONE', #26107, 1000.000000000000000 ) ;
#98146=DIRECTION ( 'NONE',  ( 0.000000000000000000, 1.000000000000000000, 0.000000000000000000 ) ) ;
#98159=CARTESIAN_POINT ( 'NONE',  ( -7.140000000000001457, -35.62921248010920294, -8.151379605006853879 ) ) ;
#98164=CARTESIAN_POINT ( 'NONE',  ( -31.92499999999997584, -22.26999999999999247, -39.50000000000000000 ) ) ;
#98205=CARTESIAN_POINT ( 'NONE',  ( 1.945313545083072748, 12.48888505241799152, -25.34115511373076046 ) ) ;
#98242=CARTESIAN_POINT ( 'NONE',  ( 12.19999999999999574, -40.43000000000000682, -40.00000000000000000 ) ) ;
#98243=SURFACE_SIDE_STYLE ('',( #29393 ) ) ;
#98315=CIRCLE ( 'NONE', #79825, 0.5000000000000004441 ) ;
#98323=PRESENTATION_STYLE_ASSIGNMENT (( #131662 ) ) ;
#98352=CARTESIAN_POINT ( 'NONE',  ( 19.04500000000000881, 3.130000000000007887, -22.35000000000000142 ) ) ;
#98373=DIRECTION ( 'NONE',  ( -1.000000000000000000, 0.000000000000000000, 0.000000000000000000 ) ) ;
#98429=ORIENTED_EDGE ( 'NONE', *, *, #102250, .T. ) ;
#98431=UNCERTAINTY_MEASURE_WITH_UNIT (LENGTH_MEASURE( 1.000000000000000082E-05 ), #119110, 'distance_accuracy_value', 'NONE');
#98465=EDGE_CURVE ( 'NONE', #118892, #13978, #129131, .T. ) ;
#98501=CARTESIAN_POINT ( 'NONE',  ( -34.92499999999997584, -6.270000000000012896, -36.39086428169088094 ) ) ;
#98562=STYLED_ITEM ( 'NONE', ( #139536 ), #91052 ) ;
#98576=( LENGTH_UNIT ( ) NAMED_UNIT ( * ) SI_UNIT ( .MILLI., .METRE. ) );
#98584=ORIENTED_EDGE ( 'NONE', *, *, #123443, .T. ) ;
#98593=SURFACE_SIDE_STYLE ('',( #99287 ) ) ;
#98617=CARTESIAN_POINT ( 'NONE',  ( 19.93618820137057668, -3.269999999999996021, -37.00000000000000000 ) ) ;
#98629=ADVANCED_FACE ( 'NONE', ( #114020 ), #80008, .T. ) ;
#98670=EDGE_LOOP ( 'NONE', ( #132646, #92546, #21607 ) ) ;
#98685=VERTEX_POINT ( 'NONE', #116871 ) ;
#98688=VECTOR ( 'NONE', #78523, 1000.000000000000000 ) ;
#98703=CARTESIAN_POINT ( 'NONE',  ( 7.139999999999985469, -39.92999999999999972, -39.50000000000000000 ) ) ;
#98704=LINE ( 'NONE', #108846, #44793 ) ;
#98706=ORIENTED_EDGE ( 'NONE', *, *, #133372, .T. ) ;
#98719=EDGE_CURVE ( 'NONE', #99826, #54868, #29670, .T. ) ;
#98726=CARTESIAN_POINT ( 'NONE',  ( -7.140000000000001457, -39.92999999999999261, -40.00000000000000000 ) ) ;
#98739=CARTESIAN_POINT ( 'NONE',  ( -19.72734424435373768, -1.609519425888390476, -32.19467225173904268 ) ) ;
#98753=PRESENTATION_STYLE_ASSIGNMENT (( #42985 ) ) ;
#98756=COLOUR_RGB ( '', 0.31764706, 0.68627451, 0.89019608) ;
#98761=CYLINDRICAL_SURFACE ( 'NONE', #94582, 2.247899999999996901 ) ;
#98776=MECHANICAL_DESIGN_GEOMETRIC_PRESENTATION_REPRESENTATION('',(#112663),#121951);
#98808=CYLINDRICAL_SURFACE ( 'NONE', #13211, 0.5000000000000004441 ) ;
#98823=DIRECTION ( 'NONE',  ( -0.000000000000000000, -0.000000000000000000, -1.000000000000000000 ) ) ;
#98844=EDGE_LOOP ( 'NONE', ( #131687, #6664, #38036 ) ) ;
#98862=CARTESIAN_POINT ( 'NONE',  ( 12.19999999999999574, -22.33999999999998565, -0.5000000000000004441 ) ) ;
#98890=CARTESIAN_POINT ( 'NONE',  ( -2.007830101563949921, 12.50197052871801340, -25.33253914797327866 ) ) ;
#98894=FACE_OUTER_BOUND ( 'NONE', #116525, .T. ) ;
#98910=DIRECTION ( 'NONE',  ( -0.000000000000000000, 1.000000000000000000, -0.000000000000000000 ) ) ;
#98917=EDGE_CURVE ( 'NONE', #129819, #9868, #133469, .T. ) ;
#98927=CARTESIAN_POINT ( 'NONE',  ( 21.59770000000000323, 3.130000000000007887, 0.000000000000000000 ) ) ;
#99008=SURFACE_STYLE_USAGE ( .BOTH. , #41075 ) ;
#99029=ORIENTED_EDGE ( 'NONE', *, *, #89128, .T. ) ;
#99136=EDGE_CURVE ( 'NONE', #6439, #111777, #85477, .T. ) ;
#99172=DIRECTION ( 'NONE',  ( 0.000000000000000000, -1.000000000000000000, 0.000000000000000000 ) ) ;
#99195=CARTESIAN_POINT ( 'NONE',  ( -34.42499999999997584, -21.76999999999999247, -0.5000000000000000000 ) ) ;
#99221=LINE ( 'NONE', #132637, #6264 ) ;
#99253=EDGE_LOOP ( 'NONE', ( #57223, #48747, #137642, #52314, #119945, #126096, #54507, #79211 ) ) ;
#99264=FILL_AREA_STYLE_COLOUR ( '', #85943 ) ;
#99278=ORIENTED_EDGE ( 'NONE', *, *, #110454, .F. ) ;
#99287=SURFACE_STYLE_FILL_AREA ( #110171 ) ;
#99316=VECTOR ( 'NONE', #117975, 1000.000000000000000 ) ;
#99318=LINE ( 'NONE', #120337, #60499 ) ;
#99324=DIRECTION ( 'NONE',  ( 0.000000000000000000, 1.000000000000000000, 0.000000000000000000 ) ) ;
#99385=ORIENTED_EDGE ( 'NONE', *, *, #44063, .T. ) ;
#99411=( NAMED_UNIT ( * ) PLANE_ANGLE_UNIT ( ) SI_UNIT ( $, .RADIAN. ) );
#99452=CARTESIAN_POINT ( 'NONE',  ( 8.603643696575190347, 12.00528567777757694, -25.64165571474893568 ) ) ;
#99463=SURFACE_STYLE_USAGE ( .BOTH. , #54581 ) ;
#99479=FACE_OUTER_BOUND ( 'NONE', #137062, .T. ) ;
#99516=AXIS2_PLACEMENT_3D ( 'NONE', #1423, #134127, #36241 ) ;
#99545=ADVANCED_FACE ( 'NONE', ( #32391 ), #12064, .F. ) ;
#99547=VERTEX_POINT ( 'NONE', #31673 ) ;
#99574=FILL_AREA_STYLE ('',( #90894 ) ) ;
#99604=COLOUR_RGB ( '', 0.09019608, 0.27058824, 0.51372549) ;
#99625=SURFACE_STYLE_USAGE ( .BOTH. , #64894 ) ;
#99729=( NAMED_UNIT ( * ) SI_UNIT ( $, .STERADIAN. ) SOLID_ANGLE_UNIT ( ) );
#99823=CARTESIAN_POINT ( 'NONE',  ( -32.09920400167933252, 22.26999999999998536, -14.71147562388301289 ) ) ;
#99826=VERTEX_POINT ( 'NONE', #106901 ) ;
#99831=CARTESIAN_POINT ( 'NONE',  ( 7.939999999999994174, -35.76999999999998892, -10.00000000000000178 ) ) ;
#99966=( NAMED_UNIT ( * ) PLANE_ANGLE_UNIT ( ) SI_UNIT ( $, .RADIAN. ) );
#99978=( NAMED_UNIT ( * ) PLANE_ANGLE_UNIT ( ) SI_UNIT ( $, .RADIAN. ) );
#99988=( BOUNDED_CURVE ( )  B_SPLINE_CURVE ( 3, ( #139828, #41183, #19439, #28898 ),
 .UNSPECIFIED., .F., .T. ) 
 B_SPLINE_CURVE_WITH_KNOTS ( ( 4, 4 ),
 ( 4.712388980384689674, 6.283185307179586232 ),
 .UNSPECIFIED. ) 
 CURVE ( )  GEOMETRIC_REPRESENTATION_ITEM ( )  RATIONAL_B_SPLINE_CURVE ( ( 1.000000000000000000, 0.8047378541243649375, 0.8047378541243649375, 1.000000000000000000 ) ) 
 REPRESENTATION_ITEM ( '' )  );
#99999=VECTOR ( 'NONE', #123245, 1000.000000000000000 ) ;
#100001=( NAMED_UNIT ( * ) PLANE_ANGLE_UNIT ( ) SI_UNIT ( $, .RADIAN. ) );
#100005=EDGE_CURVE ( 'NONE', #106633, #58061, #23786, .T. ) ;
#100015=CARTESIAN_POINT ( 'NONE',  ( 17.00344868374274299, -0.9023935745793740804, -35.76208109637431676 ) ) ;
#100031=( GEOMETRIC_REPRESENTATION_CONTEXT ( 3 ) GLOBAL_UNCERTAINTY_ASSIGNED_CONTEXT ( ( #66506 ) ) GLOBAL_UNIT_ASSIGNED_CONTEXT ( ( #60554, #27880, #51080 ) ) REPRESENTATION_CONTEXT ( 'NONE', 'WORKASPACE' ) );
#100097=EDGE_LOOP ( 'NONE', ( #100582, #136336, #92369, #32022 ) ) ;
#100104=ADVANCED_FACE ( 'NONE', ( #136327 ), #137054, .T. ) ;
#100116=ORIENTED_EDGE ( 'NONE', *, *, #127291, .F. ) ;
#100159=SURFACE_STYLE_USAGE ( .BOTH. , #71636 ) ;
#100170=FACE_OUTER_BOUND ( 'NONE', #55720, .T. ) ;
#100206=STYLED_ITEM ( 'NONE', ( #54286 ), #78835 ) ;
#100215=DIRECTION ( 'NONE',  ( 1.248002500702738701E-15, 1.000000000000000000, -0.000000000000000000 ) ) ;
#100285=DIRECTION ( 'NONE',  ( -1.000000000000000000, 0.000000000000000000, 0.000000000000000000 ) ) ;
#100303=CARTESIAN_POINT ( 'NONE',  ( -7.140000000000001457, -35.69931938766895740, -8.025146269613532723 ) ) ;
#100348=CARTESIAN_POINT ( 'NONE',  ( 18.92835661504068412, 2.123974822113010585, -30.34497721346233590 ) ) ;
#100358=CARTESIAN_POINT ( 'NONE',  ( -7.140000000000001457, -35.76999999999998892, -7.899272885403731514 ) ) ;
#100381=VECTOR ( 'NONE', #127212, 1000.000000000000000 ) ;
#100410=EDGE_CURVE ( 'NONE', #7925, #92630, #93316, .T. ) ;
#100453=COLOUR_RGB ( '', 0.09019608, 0.27058824, 0.51372549) ;
#100465=CARTESIAN_POINT ( 'NONE',  ( -17.47596317121671206, -2.821126053013751633, -34.02141742961515547 ) ) ;
#100517=CYLINDRICAL_SURFACE ( 'NONE', #48951, 0.5000000000000004441 ) ;
#100523=EDGE_CURVE ( 'NONE', #104775, #70234, #103512, .T. ) ;
#100572=CARTESIAN_POINT ( 'NONE',  ( 17.53166427279083806, -3.156388896525972765, -35.18412642963648551 ) ) ;
#100573=VERTEX_POINT ( 'NONE', #101392 ) ;
#100582=ORIENTED_EDGE ( 'NONE', *, *, #44682, .T. ) ;
#100681=ORIENTED_EDGE ( 'NONE', *, *, #107060, .T. ) ;
#100864=SURFACE_STYLE_USAGE ( .BOTH. , #132092 ) ;
#100885=DIRECTION ( 'NONE',  ( -1.000000000000000000, -0.000000000000000000, -0.000000000000000000 ) ) ;
#100950=EDGE_CURVE ( 'NONE', #126104, #99826, #81647, .T. ) ;
#100968=ADVANCED_FACE ( 'NONE', ( #114240 ), #59873, .T. ) ;
#100979=CARTESIAN_POINT ( 'NONE',  ( -12.20000000000000284, -40.42999999999999261, -40.00000000000000000 ) ) ;
#100982=DIRECTION ( 'NONE',  ( 1.000000000000000000, 1.369518533665900312E-16, -0.000000000000000000 ) ) ;
#100991=ORIENTED_EDGE ( 'NONE', *, *, #141914, .F. ) ;
#101018=DIRECTION ( 'NONE',  ( -0.000000000000000000, -0.000000000000000000, 1.000000000000000000 ) ) ;
#101028=ORIENTED_EDGE ( 'NONE', *, *, #15831, .T. ) ;
#101049=CARTESIAN_POINT ( 'NONE',  ( -7.940000000000007496, -60.26999999999998892, -10.00000000000000178 ) ) ;
#101059=AXIS2_PLACEMENT_3D ( 'NONE', #22152, #20733, #64260 ) ;
#101068=CIRCLE ( 'NONE', #10712, 0.5000000000000004441 ) ;
#101104=FACE_BOUND ( 'NONE', #136267, .T. ) ;
#101154=ORIENTED_EDGE ( 'NONE', *, *, #103224, .F. ) ;
#101157=( NAMED_UNIT ( * ) PLANE_ANGLE_UNIT ( ) SI_UNIT ( $, .RADIAN. ) );
#101160=PLANE ( 'NONE',  #93008 ) ;
#101207=CARTESIAN_POINT ( 'NONE',  ( -12.20000000000000284, -34.64999999999999147, -40.00000000000000000 ) ) ;
#101219=CARTESIAN_POINT ( 'NONE',  ( 12.69999999999999751, -34.51840020119763608, 17.97447928118983640 ) ) ;
#101247=CARTESIAN_POINT ( 'NONE',  ( -31.92499999999997584, 22.26999999999998181, -14.71147562388301822 ) ) ;
#101253=UNCERTAINTY_MEASURE_WITH_UNIT (LENGTH_MEASURE( 1.000000000000000082E-05 ), #49543, 'distance_accuracy_value', 'NONE');
#101262=CARTESIAN_POINT ( 'NONE',  ( -12.70000000000000284, -25.33999999999998565, 2.999999999999999112 ) ) ;
#101301=B_SPLINE_CURVE_WITH_KNOTS ( 'NONE', 3,
 ( #49656, #39478, #52462, #63392, #117692, #94531, #27146, #6069, #62651, #17677 ),
 .UNSPECIFIED., .F., .F.,
 ( 4, 2, 2, 2, 4 ),
 ( 0.000000000000000000, 0.0009391669472699282553, 0.001878333894539856511, 0.002817500841809784766, 0.003756667789079713021 ),
 .UNSPECIFIED. ) ;
#101314=PLANE ( 'NONE',  #109583 ) ;
#101392=CARTESIAN_POINT ( 'NONE',  ( -12.20000000000000107, -40.29840020119761590, 19.55137198191482995 ) ) ;
#101422=FACE_OUTER_BOUND ( 'NONE', #20149, .T. ) ;
#101429=ORIENTED_EDGE ( 'NONE', *, *, #65791, .T. ) ;
#101432=( NAMED_UNIT ( * ) PLANE_ANGLE_UNIT ( ) SI_UNIT ( $, .RADIAN. ) );
#101490=ORIENTED_EDGE ( 'NONE', *, *, #114101, .F. ) ;
#101535=CARTESIAN_POINT ( 'NONE',  ( -12.70000000000000462, -22.26999999999999247, -40.00000000000000000 ) ) ;
#101552=FACE_OUTER_BOUND ( 'NONE', #69298, .T. ) ;
#101567=FILL_AREA_STYLE ('',( #89974 ) ) ;
#101582=DIRECTION ( 'NONE',  ( -0.000000000000000000, -0.9647414015272163246, 0.2631995976047502017 ) ) ;
#101590=CARTESIAN_POINT ( 'NONE',  ( -12.20000000000000284, -34.64999999999999147, -39.50000000000000000 ) ) ;
#101613=CARTESIAN_POINT ( 'NONE',  ( 9.990891321718962104, 11.37382169669887055, -26.06733581495564422 ) ) ;
#101630=ORIENTED_EDGE ( 'NONE', *, *, #98051, .F. ) ;
#101682=CARTESIAN_POINT ( 'NONE',  ( -7.940000000000007496, -39.92999999999999261, -7.752100000000004876 ) ) ;
#101714=CARTESIAN_POINT ( 'NONE',  ( 1.953608656376216022E-15, -6.270000000000002238, -37.00000000000000000 ) ) ;
#101739=CARTESIAN_POINT ( 'NONE',  ( 12.19999999999999574, -59.76999999999998892, -40.00000000000000000 ) ) ;
#101758=CARTESIAN_POINT ( 'NONE',  ( 16.45742106731621490, 0.9613713492673662264, -33.49048331797056477 ) ) ;
#101806=CARTESIAN_POINT ( 'NONE',  ( -7.140000000000001457, -35.14999999999999147, -39.50000000000000000 ) ) ;
#101821=DIRECTION ( 'NONE',  ( 1.000000000000000000, -0.000000000000000000, -0.000000000000000000 ) ) ;
#101873=DIRECTION ( 'NONE',  ( 0.000000000000000000, 0.000000000000000000, 1.000000000000000000 ) ) ;
#101874=DIRECTION ( 'NONE',  ( 0.000000000000000000, 1.000000000000000000, 0.000000000000000000 ) ) ;
#101901=EDGE_CURVE ( 'NONE', #38919, #85630, #132664, .T. ) ;
#101930=AXIS2_PLACEMENT_3D ( 'NONE', #128648, #96690, #29320 ) ;
#101940=DIRECTION ( 'NONE',  ( 1.321231229586337907E-16, -0.9647414015272156584, 0.2631995976047526442 ) ) ;
#101989=CARTESIAN_POINT ( 'NONE',  ( 17.42520222878246372, -2.544454608235909188, -33.49760814689099675 ) ) ;
#102020=CIRCLE ( 'NONE', #30192, 0.5000000000000004441 ) ;
#102041=SURFACE_STYLE_FILL_AREA ( #37515 ) ;
#102051=DIRECTION ( 'NONE',  ( 1.321231229586337907E-16, -0.9647414015272156584, 0.2631995976047526442 ) ) ;
#102162=CARTESIAN_POINT ( 'NONE',  ( -12.20000000000000462, -22.33999999999998565, 3.000000000000000000 ) ) ;
#102250=EDGE_CURVE ( 'NONE', #22506, #117264, #58361, .T. ) ;
#102255=EDGE_LOOP ( 'NONE', ( #80927, #56346, #30445, #38850, #9298 ) ) ;
#102276=CARTESIAN_POINT ( 'NONE',  ( -19.93618820137057668, -6.270000000050818478, -40.00000000000000000 ) ) ;
#102326=DIRECTION ( 'NONE',  ( 3.166071393695993333E-32, -1.016133275908817741E-16, 1.000000000000000000 ) ) ;
#102358=ORIENTED_EDGE ( 'NONE', *, *, #112441, .F. ) ;
#102367=SURFACE_SIDE_STYLE ('',( #90023 ) ) ;
#102424=COLOUR_RGB ( '', 0.08235294, 0.09019608, 0.10196078) ;
#102432=FILL_AREA_STYLE ('',( #48045 ) ) ;
#102447=ORIENTED_EDGE ( 'NONE', *, *, #141914, .T. ) ;
#102450=ORIENTED_EDGE ( 'NONE', *, *, #44544, .F. ) ;
#102453=CARTESIAN_POINT ( 'NONE',  ( 32.09873525369289382, 22.27000000000000668, -14.71147562388300045 ) ) ;
#102469=ORIENTED_EDGE ( 'NONE', *, *, #140396, .F. ) ;
#102555=STYLED_ITEM ( 'NONE', ( #91863 ), #62426 ) ;
#102563=EDGE_CURVE ( 'NONE', #43110, #9868, #54008, .T. ) ;
#102567=UNCERTAINTY_MEASURE_WITH_UNIT (LENGTH_MEASURE( 1.000000000000000082E-05 ), #21150, 'distance_accuracy_value', 'NONE');
#102603=EDGE_CURVE ( 'NONE', #23998, #59778, #67613, .T. ) ;
#102613=CARTESIAN_POINT ( 'NONE',  ( -19.39435030839552709, 0.5803129815428644811, -30.75302245446138727 ) ) ;
#102618=DIRECTION ( 'NONE',  ( 0.000000000000000000, 0.000000000000000000, 1.000000000000000000 ) ) ;
#102660=EDGE_CURVE ( 'NONE', #132295, #84209, #25481, .T. ) ;
#102715=CYLINDRICAL_SURFACE ( 'NONE', #88133, 0.5000000000000001110 ) ;
#102756=CARTESIAN_POINT ( 'NONE',  ( -34.42499999999997584, 22.27000000000000668, 0.000000000000000000 ) ) ;
#102788=DIRECTION ( 'NONE',  ( 1.000000000000000000, 0.000000000000000000, 0.000000000000000000 ) ) ;
#102819=CARTESIAN_POINT ( 'NONE',  ( 7.139999999999956160, -60.26999999999998892, -12.10072711459626227 ) ) ;
#102840=FACE_BOUND ( 'NONE', #119968, .T. ) ;
#102847=AXIS2_PLACEMENT_3D ( 'NONE', #90078, #23395, #24131 ) ;
#102853=DIRECTION ( 'NONE',  ( 0.000000000000000000, 0.000000000000000000, -1.000000000000000000 ) ) ;
#102882=CARTESIAN_POINT ( 'NONE',  ( 0.000000000000000000, -34.64999999999999147, 17.49210858042621908 ) ) ;
#102885=EDGE_LOOP ( 'NONE', ( #42330, #40247, #126539, #3497 ) ) ;
#102963=CIRCLE ( 'NONE', #40469, 0.5000000000000004441 ) ;
#102966=ORIENTED_EDGE ( 'NONE', *, *, #24635, .T. ) ;
#102987=ORIENTED_EDGE ( 'NONE', *, *, #131135, .T. ) ;
#103016=DIRECTION ( 'NONE',  ( 0.000000000000000000, 0.000000000000000000, -1.000000000000000000 ) ) ;
#103034=PLANE ( 'NONE',  #23095 ) ;
#103041=PRESENTATION_STYLE_ASSIGNMENT (( #138529 ) ) ;
#103141=SURFACE_SIDE_STYLE ('',( #58986 ) ) ;
#103145=FACE_OUTER_BOUND ( 'NONE', #63518, .T. ) ;
#103193=CARTESIAN_POINT ( 'NONE',  ( -12.20000000000000284, -40.42999999999999261, -39.50000000000000000 ) ) ;
#103201=CARTESIAN_POINT ( 'NONE',  ( 7.940000000000001279, -33.26999999999999602, -11.89864999999999462 ) ) ;
#103219=AXIS2_PLACEMENT_3D ( 'NONE', #100979, #43754, #100285 ) ;
#103224=EDGE_CURVE ( 'NONE', #48074, #21068, #26352, .T. ) ;
#103236=ADVANCED_FACE ( 'NONE', ( #105021 ), #47208, .T. ) ;
#103250=CARTESIAN_POINT ( 'NONE',  ( 7.139999999999991687, -35.62921248010918873, -8.151379605006875195 ) ) ;
#103256=DIRECTION ( 'NONE',  ( 2.173158128376833625E-16, -1.000000000000000000, 0.000000000000000000 ) ) ;
#103257=VECTOR ( 'NONE', #96432, 1000.000000000000000 ) ;
#103281=ADVANCED_FACE ( 'NONE', ( #141970 ), #45026, .F. ) ;
#103303=AXIS2_PLACEMENT_3D ( 'NONE', #51116, #37378, #127216 ) ;
#103336=CARTESIAN_POINT ( 'NONE',  ( -14.16207406425801807, 5.380563507462931661, -29.22689065742943981 ) ) ;
#103342=CARTESIAN_POINT ( 'NONE',  ( 34.92500000000001847, -3.269999999999991580, -36.39086428169088094 ) ) ;
#103351=DIRECTION ( 'NONE',  ( -0.000000000000000000, -1.000000000000000000, -0.000000000000000000 ) ) ;
#103352=VERTEX_POINT ( 'NONE', #56412 ) ;
#103354=ORIENTED_EDGE ( 'NONE', *, *, #85080, .T. ) ;
#103367=CARTESIAN_POINT ( 'NONE',  ( -34.92499999999996874, 22.27000000000001023, -8.436850734044138989 ) ) ;
#103385=DIRECTION ( 'NONE',  ( 1.000000000000000000, 0.000000000000000000, 0.000000000000000000 ) ) ;
#103388=CARTESIAN_POINT ( 'NONE',  ( 16.82833281552586868, -0.2148806029953220509, -34.28722974112268673 ) ) ;
#103389=ORIENTED_EDGE ( 'NONE', *, *, #98917, .F. ) ;
#103401=CARTESIAN_POINT ( 'NONE',  ( -12.20000000000000462, -22.33999999999998565, 3.000000000000000000 ) ) ;
#103410=( GEOMETRIC_REPRESENTATION_CONTEXT ( 3 ) GLOBAL_UNCERTAINTY_ASSIGNED_CONTEXT ( ( #112703 ) ) GLOBAL_UNIT_ASSIGNED_CONTEXT ( ( #30024, #86583, #118466 ) ) REPRESENTATION_CONTEXT ( 'NONE', 'WORKASPACE' ) );
#103411=CARTESIAN_POINT ( 'NONE',  ( -7.940000000000007496, -60.26999999999998892, -12.24789999999999957 ) ) ;
#103434=CARTESIAN_POINT ( 'NONE',  ( -12.69999999999999929, -59.76999999999998892, -39.50000000000000000 ) ) ;
#103440=VECTOR ( 'NONE', #75862, 1000.000000000000000 ) ;
#103441=( NAMED_UNIT ( * ) PLANE_ANGLE_UNIT ( ) SI_UNIT ( $, .RADIAN. ) );
#103454=AXIS2_PLACEMENT_3D ( 'NONE', #74799, #84249, #116839 ) ;
#103475=( BOUNDED_SURFACE ( )  B_SPLINE_SURFACE ( 3, 2, ( 
 ( #40280, #37395, #3983 ),
 ( #48262, #117071, #17748 ),
 ( #59865, #17071, #104784 ),
 ( #26517, #6143, #39555 ),
 ( #81640, #51135, #38825 ),
 ( #92457, #103336, #6856 ),
 ( #27939, #4697, #115614 ),
 ( #136691, #48995, #114908 ),
 ( #15586, #27212, #138139 ),
 ( #137431, #28677, #82341 ),
 ( #16318, #50420, #84486 ),
 ( #71455, #93901, #70068 ),
 ( #60611, #126525, #5444 ),
 ( #49726, #62023, #83041 ),
 ( #127239, #61334, #106179 ),
 ( #114233, #94606, #59183 ),
 ( #138861, #83782, #54010 ),
 ( #64870, #108312, #19900 ),
 ( #8291, #109051, #32230 ),
 ( #96039, #40965, #107629 ),
 ( #63465, #9741, #42418 ),
 ( #120634, #98890, #143124 ),
 ( #65614, #30823, #43819 ),
 ( #88037, #8984, #119218 ),
 ( #52541, #64151, #31517 ),
 ( #74318, #98205, #109782 ),
 ( #142432, #96723, #75049 ),
 ( #53244, #140276, #85884 ),
 ( #75741, #43118, #41671 ),
 ( #97461, #29351, #141713 ),
 ( #140966, #87328, #130122 ),
 ( #131541, #86630, #130853 ),
 ( #129379, #76465, #119911 ),
 ( #20615, #85163, #21351 ),
 ( #10450, #54710, #73596 ),
 ( #30067, #117763, #18453 ),
 ( #106915, #62736, #7594 ),
 ( #51854, #118508, #19207 ),
 ( #66298, #111188, #110471 ),
 ( #33679, #89454, #56878 ),
 ( #11875, #46732, #11141 ),
 ( #3150, #113333, #133689 ),
 ( #34372, #12603, #132287 ),
 ( #78592, #88771, #56164 ),
 ( #122801, #135143, #100348 ),
 ( #101758, #13301, #23483 ) ),
 .UNSPECIFIED., .F., .F., .F. ) 
 B_SPLINE_SURFACE_WITH_KNOTS ( ( 4, 2, 2, 2, 2, 2, 2, 2, 2, 2, 2, 2, 2, 2, 2, 2, 2, 2, 2, 2, 2, 2, 4 ),
 ( 3, 3 ),
 ( 2.602085213965210642E-18, 0.003250134860695850971, 0.006500269721391699340, 0.008125337151739624175, 0.009750404582087547276, 0.01300053944278339521, 0.01462560687313131831, 0.01625067430347924141, 0.01950080916417509108, 0.02112587659452301592, 0.02275094402487094075, 0.02600107888556678695, 0.02762614631591470832, 0.02925121374626263315, 0.03250134860695848282, 0.03412641603730640766, 0.03575148346765433249, 0.03900161832835018216, 0.04225175318904603183, 0.04550188804974188150, 0.04712695548008980634, 0.04875202291043773117, 0.05200215777113357390 ),
 ( 0.000000000000000000, 1.000000000000000000 ),
 .UNSPECIFIED. ) 
 GEOMETRIC_REPRESENTATION_ITEM ( )  RATIONAL_B_SPLINE_SURFACE ( (
 ( 1.000000000000000000, 0.7366656399173064917, 1.000000000000000000),
 ( 1.000000000000000000, 0.7439429771432026772, 1.000000000000000000),
 ( 1.000000000000000000, 0.7520594078564465379, 1.000000000000000000),
 ( 1.000000000000000000, 0.7692526947351095989, 1.000000000000000000),
 ( 1.000000000000000000, 0.7783293130759435519, 1.000000000000000000),
 ( 1.000000000000000000, 0.7922221006548060274, 1.000000000000000000),
 ( 1.000000000000000000, 0.7969161081511108025, 1.000000000000000000),
 ( 1.000000000000000000, 0.8061991495951973397, 1.000000000000000000),
 ( 1.000000000000000000, 0.8107995347775716066, 1.000000000000000000),
 ( 1.000000000000000000, 0.8243916883358404224, 1.000000000000000000),
 ( 1.000000000000000000, 0.8331742881454423655, 1.000000000000000000),
 ( 1.000000000000000000, 0.8456175635000574564, 1.000000000000000000),
 ( 1.000000000000000000, 0.8496437749331391398, 1.000000000000000000),
 ( 1.000000000000000000, 0.8573989149376710639, 1.000000000000000000),
 ( 1.000000000000000000, 0.8610920168694898846, 1.000000000000000000),
 ( 1.000000000000000000, 0.8715094877776208282, 1.000000000000000000),
 ( 1.000000000000000000, 0.8775986680032793474, 1.000000000000000000),
 ( 1.000000000000000000, 0.8851898980576022868, 1.000000000000000000),
 ( 1.000000000000000000, 0.8874625043875524755, 1.000000000000000000),
 ( 1.000000000000000000, 0.8914353813151855155, 1.000000000000000000),
 ( 1.000000000000000000, 0.8931046208065658298, 1.000000000000000000),
 ( 1.000000000000000000, 0.8971318440585478449, 1.000000000000000000),
 ( 1.000000000000000000, 0.8985209499677152545, 1.000000000000000000),
 ( 1.000000000000000000, 0.8985769579961769837, 1.000000000000000000),
 ( 1.000000000000000000, 0.8982569968411678873, 1.000000000000000000),
 ( 1.000000000000000000, 0.8969164612184702401, 1.000000000000000000),
 ( 1.000000000000000000, 0.8959054417035888784, 1.000000000000000000),
 ( 1.000000000000000000, 0.8919262031741450603, 1.000000000000000000),
 ( 1.000000000000000000, 0.8880110869415998032, 1.000000000000000000),
 ( 1.000000000000000000, 0.8804381194099686336, 1.000000000000000000),
 ( 1.000000000000000000, 0.8776206763866101213, 1.000000000000000000),
 ( 1.000000000000000000, 0.8715502808905819521, 1.000000000000000000),
 ( 1.000000000000000000, 0.8682884511766901792, 1.000000000000000000),
 ( 1.000000000000000000, 0.8578980603305481623, 1.000000000000000000),
 ( 1.000000000000000000, 0.8501653997698138676, 1.000000000000000000),
 ( 1.000000000000000000, 0.8334322383353173214, 1.000000000000000000),
 ( 1.000000000000000000, 0.8246054523620813814, 1.000000000000000000),
 ( 1.000000000000000000, 0.8064801979543902988, 1.000000000000000000),
 ( 1.000000000000000000, 0.7971768814008325377, 1.000000000000000000),
 ( 1.000000000000000000, 0.7832300806951568717, 1.000000000000000000),
 ( 1.000000000000000000, 0.7785857309249303304, 1.000000000000000000),
 ( 1.000000000000000000, 0.7695076527920222675, 1.000000000000000000),
 ( 1.000000000000000000, 0.7650571017203612323, 1.000000000000000000),
 ( 1.000000000000000000, 0.7520869309904180122, 1.000000000000000000),
 ( 1.000000000000000000, 0.7439459459532327124, 1.000000000000000000),
 ( 1.000000000000000000, 0.7366656399173067138, 1.000000000000000000) ) ) 
 REPRESENTATION_ITEM ( '' )  SURFACE ( )  );
#103484=CARTESIAN_POINT ( 'NONE',  ( 7.139999999999992575, -35.13237070076360169, 17.62370837922859934 ) ) ;
#103511=CARTESIAN_POINT ( 'NONE',  ( 0.000000000000000000, 0.000000000000000000, 0.000000000000000000 ) ) ;
#103512=LINE ( 'NONE', #69509, #44726 ) ;
#103542=CARTESIAN_POINT ( 'NONE',  ( -7.940000000000001279, -35.14999999999999147, -8.101350000000007157 ) ) ;
#103629=STYLED_ITEM ( 'NONE', ( #56889 ), #125580 ) ;
#103681=EDGE_LOOP ( 'NONE', ( #65998, #6912, #662, #114881, #77544, #122191, #125424, #111586 ) ) ;
#103692=ORIENTED_EDGE ( 'NONE', *, *, #43017, .F. ) ;
#103720=CARTESIAN_POINT ( 'NONE',  ( 12.69999999999999574, -59.76999999999998892, 24.34531699603382293 ) ) ;
#103744=DIRECTION ( 'NONE',  ( -1.000000000000000000, 1.248002500702738701E-15, -3.404785525682857987E-16 ) ) ;
#103756=VERTEX_POINT ( 'NONE', #34267 ) ;
#103768=CARTESIAN_POINT ( 'NONE',  ( -5.098242758349162962, 11.83526629088845361, -27.40386350861210119 ) ) ;
#103831=VECTOR ( 'NONE', #38692, 1000.000000000000000 ) ;
#103870=STYLED_ITEM ( 'NONE', ( #63786 ), #56651 ) ;
#103912=ADVANCED_FACE ( 'NONE', ( #58931 ), #37111, .T. ) ;
#103937=UNCERTAINTY_MEASURE_WITH_UNIT (LENGTH_MEASURE( 1.000000000000000082E-05 ), #48620, 'distance_accuracy_value', 'NONE');
#104065=CARTESIAN_POINT ( 'NONE',  ( 12.19999999999999574, -21.76999999999999247, -40.00000000000000000 ) ) ;
#104108=DIRECTION ( 'NONE',  ( -0.8571673007021110013, 1.049727191138617093E-16, 0.5150380749100563760 ) ) ;
#104149=CARTESIAN_POINT ( 'NONE',  ( -7.940000000000001279, -33.26999999999999602, -10.00000000000000178 ) ) ;
#104164=ORIENTED_EDGE ( 'NONE', *, *, #62862, .T. ) ;
#104276=DIRECTION ( 'NONE',  ( -1.369518533665900312E-16, 1.000000000000000000, -0.000000000000000000 ) ) ;
#104316=CARTESIAN_POINT ( 'NONE',  ( 34.92500000000001847, 1.088194295437629318E-14, -37.00000000000000000 ) ) ;
#104352=CARTESIAN_POINT ( 'NONE',  ( 0.000000000000000000, -35.14999999999999147, 17.49210858042621908 ) ) ;
#104402=CARTESIAN_POINT ( 'NONE',  ( 31.92500000000002203, -21.76999999999999247, -37.00000000000000000 ) ) ;
#104404=CIRCLE ( 'NONE', #136812, 3.000000000000002665 ) ;
#104443=CIRCLE ( 'NONE', #132223, 2.999999999999999112 ) ;
#104464=FACE_OUTER_BOUND ( 'NONE', #46455, .T. ) ;
#104537=PRESENTATION_STYLE_ASSIGNMENT (( #80670 ) ) ;
#104575=FILL_AREA_STYLE ('',( #125634 ) ) ;
#104577=AXIS2_PLACEMENT_3D ( 'NONE', #26280, #37886, #70542 ) ;
#104579=DIRECTION ( 'NONE',  ( -0.9425785261922232650, 0.3339846133601012124, 0.000000000000000000 ) ) ;
#104606=FACE_OUTER_BOUND ( 'NONE', #102885, .T. ) ;
#104610=COLOUR_RGB ( '', 0.66274510, 0.83137255, 0.94901961) ;
#104623=CIRCLE ( 'NONE', #81481, 2.247899999999996901 ) ;
#104627=FACE_OUTER_BOUND ( 'NONE', #121072, .T. ) ;
#104680=EDGE_CURVE ( 'NONE', #34178, #119435, #86790, .T. ) ;
#104695=VECTOR ( 'NONE', #86400, 1000.000000000000000 ) ;
#104719=DIRECTION ( 'NONE',  ( 0.000000000000000000, -0.000000000000000000, -1.000000000000000000 ) ) ;
#104741=FACE_BOUND ( 'NONE', #38470, .T. ) ;
#104775=VERTEX_POINT ( 'NONE', #103434 ) ;
#104784=CARTESIAN_POINT ( 'NONE',  ( -18.50179702988272012, 3.003944652846646690, -30.07174397188686399 ) ) ;
#104792=EDGE_LOOP ( 'NONE', ( #61634, #35779, #95467, #135023 ) ) ;
#104797=EDGE_CURVE ( 'NONE', #61905, #92723, #35901, .T. ) ;
#104839=EDGE_CURVE ( 'NONE', #34178, #99547, #54416, .T. ) ;
#104847=AXIS2_PLACEMENT_3D ( 'NONE', #8547, #76743, #143393 ) ;
#104849=ORIENTED_EDGE ( 'NONE', *, *, #22505, .F. ) ;
#104914=CARTESIAN_POINT ( 'NONE',  ( -7.940000000000001279, -33.26999999999999602, -10.00000000000000178 ) ) ;
#104927=( LENGTH_UNIT ( ) NAMED_UNIT ( * ) SI_UNIT ( .MILLI., .METRE. ) );
#104972=DIRECTION ( 'NONE',  ( 0.000000000000000000, -1.000000000000000000, 0.000000000000000000 ) ) ;
#104983=ORIENTED_EDGE ( 'NONE', *, *, #76417, .F. ) ;
#105007=ORIENTED_EDGE ( 'NONE', *, *, #122212, .T. ) ;
#105021=FACE_OUTER_BOUND ( 'NONE', #43620, .T. ) ;
#105031=ORIENTED_EDGE ( 'NONE', *, *, #74636, .F. ) ;
#105035=FILL_AREA_STYLE ('',( #60874 ) ) ;
#105090=ORIENTED_EDGE ( 'NONE', *, *, #70339, .F. ) ;
#105120=ORIENTED_EDGE ( 'NONE', *, *, #73593, .T. ) ;
#105132=PRESENTATION_STYLE_ASSIGNMENT (( #6482 ) ) ;
#105149=FACE_OUTER_BOUND ( 'NONE', #93693, .T. ) ;
#105172=FILL_AREA_STYLE_COLOUR ( '', #83702 ) ;
#105200=CARTESIAN_POINT ( 'NONE',  ( 31.92500000000001492, -3.269999999999992024, -40.00000000000000000 ) ) ;
#105227=( BOUNDED_CURVE ( )  B_SPLINE_CURVE ( 3, ( #93648, #105911, #8029, #84901 ),
 .UNSPECIFIED., .F., .T. ) 
 B_SPLINE_CURVE_WITH_KNOTS ( ( 4, 4 ),
 ( 4.446051736530363563, 4.712388980384695003 ),
 .UNSPECIFIED. ) 
 CURVE ( )  GEOMETRIC_REPRESENTATION_ITEM ( )  RATIONAL_B_SPLINE_CURVE ( ( 1.000000000000000000, 0.9940974367313476501, 0.9940974367313476501, 1.000000000000000000 ) ) 
 REPRESENTATION_ITEM ( '' )  );
#105257=ORIENTED_EDGE ( 'NONE', *, *, #94279, .F. ) ;
#105266=EDGE_CURVE ( 'NONE', #67375, #132883, #101301, .T. ) ;
#105273=CARTESIAN_POINT ( 'NONE',  ( 14.08979869950237251, -1.618973607074033705, -40.00000000000000000 ) ) ;
#105300=PRESENTATION_STYLE_ASSIGNMENT (( #114037 ) ) ;
#105357=ORIENTED_EDGE ( 'NONE', *, *, #24427, .T. ) ;
#105365=EDGE_CURVE ( 'NONE', #119435, #118785, #131474, .T. ) ;
#105388=VECTOR ( 'NONE', #75667, 1000.000000000000000 ) ;
#105393=EDGE_CURVE ( 'NONE', #85630, #68517, #11075, .T. ) ;
#105404=EDGE_LOOP ( 'NONE', ( #33919, #110626, #99385, #120478, #20823, #77200, #88973, #96500 ) ) ;
#105411=ORIENTED_EDGE ( 'NONE', *, *, #130115, .T. ) ;
#105415=EDGE_CURVE ( 'NONE', #27902, #131125, #13759, .T. ) ;
#105432=ADVANCED_FACE ( 'NONE', ( #86549 ), #108971, .T. ) ;
#105440=PRESENTATION_STYLE_ASSIGNMENT (( #116335 ) ) ;
#105442=CARTESIAN_POINT ( 'NONE',  ( 12.19999999999999574, -27.68200100598810565, 15.59110741220538188 ) ) ;
#105479=( LENGTH_UNIT ( ) NAMED_UNIT ( * ) SI_UNIT ( .MILLI., .METRE. ) );
#105501=DIRECTION ( 'NONE',  ( 0.000000000000000000, 1.000000000000000000, 0.000000000000000000 ) ) ;
#105603=CARTESIAN_POINT ( 'NONE',  ( 7.139999999999956160, -35.56014942880460694, -11.72188031596273206 ) ) ;
#105610=MECHANICAL_DESIGN_GEOMETRIC_PRESENTATION_REPRESENTATION('',(#135656),#80213);
#105620=CARTESIAN_POINT ( 'NONE',  ( 12.19999999999999574, -60.26999999999998892, 25.00000000000000000 ) ) ;
#105632=CYLINDRICAL_SURFACE ( 'NONE', #133880, 0.5000000000000004441 ) ;
#105692=ORIENTED_EDGE ( 'NONE', *, *, #135087, .T. ) ;
#105723=CARTESIAN_POINT ( 'NONE',  ( -31.92499999999997584, -6.270000000000012896, -40.00000000000000000 ) ) ;
#105726=CARTESIAN_POINT ( 'NONE',  ( -7.140000000000001457, -35.14999999999999147, -8.278119684037250181 ) ) ;
#105738=LINE ( 'NONE', #104316, #42949 ) ;
#105753=CARTESIAN_POINT ( 'NONE',  ( -12.20000000000000284, -40.42999999999999261, -40.00000000000000000 ) ) ;
#105787=ADVANCED_FACE ( 'NONE', ( #116424 ), #17111, .F. ) ;
#105810=CARTESIAN_POINT ( 'NONE',  ( 7.139999999999985469, -39.92999999999999972, -39.50000000000000000 ) ) ;
#105825=ORIENTED_EDGE ( 'NONE', *, *, #116835, .F. ) ;
#105876=UNCERTAINTY_MEASURE_WITH_UNIT (LENGTH_MEASURE( 1.000000000000000082E-05 ), #104927, 'distance_accuracy_value', 'NONE');
#105885=CARTESIAN_POINT ( 'NONE',  ( 7.940000000000001279, -60.26999999999998892, -8.101350000000007157 ) ) ;
#105894=ORIENTED_EDGE ( 'NONE', *, *, #35327, .T. ) ;
#105904=VECTOR ( 'NONE', #72889, 1000.000000000000000 ) ;
#105910=CARTESIAN_POINT ( 'NONE',  ( -6.391038532768485325, 11.40365449930913222, -27.77063147129241116 ) ) ;
#105911=CARTESIAN_POINT ( 'NONE',  ( -6.728648308968876890, -34.60547875340945723, 17.99210858042622263 ) ) ;
#105967=AXIS2_PLACEMENT_3D ( 'NONE', #10598, #55575, #63611 ) ;
#106082=CARTESIAN_POINT ( 'NONE',  ( 31.92500000000001492, 2.730000000000007088, -36.39086428169088094 ) ) ;
#106085=ADVANCED_FACE ( 'NONE', ( #69300 ), #122959, .F. ) ;
#106087=DIRECTION ( 'NONE',  ( -1.000000000000000000, -3.115803279706882722E-16, -0.000000000000000000 ) ) ;
#106088=AXIS2_PLACEMENT_3D ( 'NONE', #39214, #92861, #50098 ) ;
#106112=DIRECTION ( 'NONE',  ( 0.000000000000000000, -0.5150380749100594846, -0.8571673007021091140 ) ) ;
#106126=ORIENTED_EDGE ( 'NONE', *, *, #137656, .T. ) ;
#106138=LINE ( 'NONE', #85132, #105904 ) ;
#106156=EDGE_CURVE ( 'NONE', #13538, #40966, #15333, .T. ) ;
#106179=CARTESIAN_POINT ( 'NONE',  ( -9.771348248178298945, 11.46486773387262126, -26.00442996100349546 ) ) ;
#106189=ORIENTED_EDGE ( 'NONE', *, *, #89128, .F. ) ;
#106369=VERTEX_POINT ( 'NONE', #101739 ) ;
#106386=FILL_AREA_STYLE ('',( #108530 ) ) ;
#106409=DIRECTION ( 'NONE',  ( -1.000000000000000000, 0.000000000000000000, 0.000000000000000000 ) ) ;
#106410=PRESENTATION_STYLE_ASSIGNMENT (( #96257 ) ) ;
#106420=ORIENTED_EDGE ( 'NONE', *, *, #50412, .T. ) ;
#106480=( NAMED_UNIT ( * ) SI_UNIT ( $, .STERADIAN. ) SOLID_ANGLE_UNIT ( ) );
#106493=ADVANCED_FACE ( 'NONE', ( #39362 ), #126343, .T. ) ;
#106501=DIRECTION ( 'NONE',  ( -1.000000000000000000, 0.000000000000000000, -0.000000000000000000 ) ) ;
#106551=CARTESIAN_POINT ( 'NONE',  ( 7.139999999999985469, -39.93000000000000682, 18.97874025153853239 ) ) ;
#106557=CARTESIAN_POINT ( 'NONE',  ( -12.20000000000000107, -40.42999999999999261, 19.06900128115122328 ) ) ;
#106564=CARTESIAN_POINT ( 'NONE',  ( 12.69999999999999574, -60.40159979880236563, 24.51762929923639334 ) ) ;
#106611=( GEOMETRIC_REPRESENTATION_CONTEXT ( 3 ) GLOBAL_UNCERTAINTY_ASSIGNED_CONTEXT ( ( #111406 ) ) GLOBAL_UNIT_ASSIGNED_CONTEXT ( ( #8051, #85616, #5190 ) ) REPRESENTATION_CONTEXT ( 'NONE', 'WORKASPACE' ) );
#106621=CARTESIAN_POINT ( 'NONE',  ( -15.78802419517198352, 2.637730036045195625, -32.92692751918610128 ) ) ;
#106633=VERTEX_POINT ( 'NONE', #107440 ) ;
#106680=CARTESIAN_POINT ( 'NONE',  ( -12.20000000000000284, -39.92999999999999261, 19.06900128115122328 ) ) ;
#106683=CARTESIAN_POINT ( 'NONE',  ( 34.92500000000002558, -22.06289321881344634, -2.893915774544653381E-16 ) ) ;
#106755=EDGE_CURVE ( 'NONE', #61841, #126832, #15423, .T. ) ;
#106832=( GEOMETRIC_REPRESENTATION_CONTEXT ( 3 ) GLOBAL_UNCERTAINTY_ASSIGNED_CONTEXT ( ( #1205 ) ) GLOBAL_UNIT_ASSIGNED_CONTEXT ( ( #112057, #101157, #99729 ) ) REPRESENTATION_CONTEXT ( 'NONE', 'WORKASPACE' ) );
#106837=EDGE_CURVE ( 'NONE', #59938, #237, #121924, .T. ) ;
#106840=ADVANCED_FACE ( 'NONE', ( #101552 ), #47252, .T. ) ;
#106875=DIRECTION ( 'NONE',  ( 0.000000000000000000, -0.2631995976047557528, -0.9647414015272147703 ) ) ;
#106878=( NAMED_UNIT ( * ) SI_UNIT ( $, .STERADIAN. ) SOLID_ANGLE_UNIT ( ) );
#106895=CARTESIAN_POINT ( 'NONE',  ( 12.19999999999999574, -22.33999999999998565, 3.000000000000000000 ) ) ;
#106901=CARTESIAN_POINT ( 'NONE',  ( 34.92500000000002558, -21.76999999999999247, 0.000000000000000000 ) ) ;
#106904=DIRECTION ( 'NONE',  ( 0.8571673007021110013, 0.000000000000000000, 0.5150380749100563760 ) ) ;
#106915=CARTESIAN_POINT ( 'NONE',  ( 11.57112785411878519, 8.234238653253980189, -30.09936050942188857 ) ) ;
#106917=ADVANCED_FACE ( 'NONE', ( #136328 ), #27551, .F. ) ;
#106930=ORIENTED_EDGE ( 'NONE', *, *, #108652, .T. ) ;
#106937=DIRECTION ( 'NONE',  ( 1.000000000000000000, 3.115803279706882722E-16, 0.000000000000000000 ) ) ;
#106940=CARTESIAN_POINT ( 'NONE',  ( -12.20000000000000284, -40.42999999999999261, -39.50000000000000000 ) ) ;
#106954=ORIENTED_EDGE ( 'NONE', *, *, #102603, .F. ) ;
#107034=( GEOMETRIC_REPRESENTATION_CONTEXT ( 3 ) GLOBAL_UNCERTAINTY_ASSIGNED_CONTEXT ( ( #12803 ) ) GLOBAL_UNIT_ASSIGNED_CONTEXT ( ( #9369, #100001, #76847 ) ) REPRESENTATION_CONTEXT ( 'NONE', 'WORKASPACE' ) );
#107060=EDGE_CURVE ( 'NONE', #9707, #64319, #51486, .T. ) ;
#107067=CARTESIAN_POINT ( 'NONE',  ( -0.000000000000000000, -22.33999999999998565, 3.000000000000000000 ) ) ;
#107071=AXIS2_PLACEMENT_3D ( 'NONE', #106940, #105501, #83063 ) ;
#107130=ADVANCED_FACE ( 'NONE', ( #24546 ), #52847, .F. ) ;
#107147=PRESENTATION_STYLE_ASSIGNMENT (( #129612 ) ) ;
#107167=ADVANCED_FACE ( 'NONE', ( #1342 ), #68800, .T. ) ;
#107222=CARTESIAN_POINT ( 'NONE',  ( -7.140000000000001457, -60.26999999999998892, -8.278119684037250181 ) ) ;
#107247=CARTESIAN_POINT ( 'NONE',  ( 19.93618820135885272, -3.269999999999997353, -36.05817462077273916 ) ) ;
#107279=EDGE_CURVE ( 'NONE', #23962, #71803, #80389, .T. ) ;
#107343=VECTOR ( 'NONE', #78240, 1000.000000000000000 ) ;
#107362=CARTESIAN_POINT ( 'NONE',  ( 15.78699708688048631, 2.640433550745856728, -32.92603572637591469 ) ) ;
#107440=CARTESIAN_POINT ( 'NONE',  ( -17.01299345043647548, -0.9444868035624306435, -36.99999999997771738 ) ) ;
#107500=CARTESIAN_POINT ( 'NONE',  ( 7.940000000000001279, -60.26999999999998892, -11.89864999999999640 ) ) ;
#107519=DIRECTION ( 'NONE',  ( 0.000000000000000000, 0.000000000000000000, -1.000000000000000000 ) ) ;
#107522=DIRECTION ( 'NONE',  ( 0.000000000000000000, -1.000000000000000000, 0.000000000000000000 ) ) ;
#107584=CARTESIAN_POINT ( 'NONE',  ( -19.05499999999999261, 3.130000000000007887, -22.35000000000000142 ) ) ;
#107597=SURFACE_SIDE_STYLE ('',( #51819 ) ) ;
#107629=CARTESIAN_POINT ( 'NONE',  ( -4.332298631122367460, 13.32507652626317096, -24.69132185691248438 ) ) ;
#107679=CARTESIAN_POINT ( 'NONE',  ( -6.874395825605905230, -40.07226884389044841, 19.48967909493512352 ) ) ;
#107686=SURFACE_STYLE_FILL_AREA ( #19961 ) ;
#107808=DIRECTION ( 'NONE',  ( 0.000000000000000000, 0.9647414015272155474, -0.2631995976047525887 ) ) ;
#107817=FILL_AREA_STYLE_COLOUR ( '', #129499 ) ;
#107878=CYLINDRICAL_SURFACE ( 'NONE', #123407, 0.5000000000000004441 ) ;
#107998=CARTESIAN_POINT ( 'NONE',  ( 19.04500000000000881, 3.130000000000007887, 0.000000000000000000 ) ) ;
#108023=DIRECTION ( 'NONE',  ( -0.000000000000000000, -1.000000000000000000, -0.000000000000000000 ) ) ;
#108054=CARTESIAN_POINT ( 'NONE',  ( -9.524999999999998579, -4.870000000000014317, -40.00000000000000000 ) ) ;
#108105=ORIENTED_EDGE ( 'NONE', *, *, #30345, .F. ) ;
#108151=ADVANCED_FACE ( 'NONE', ( #91005 ), #89546, .T. ) ;
#108200=( NAMED_UNIT ( * ) SI_UNIT ( $, .STERADIAN. ) SOLID_ANGLE_UNIT ( ) );
#108300=DIRECTION ( 'NONE',  ( 0.000000000000000000, 1.000000000000000000, 0.000000000000000000 ) ) ;
#108303=EDGE_CURVE ( 'NONE', #85621, #58156, #29281, .T. ) ;
#108312=CARTESIAN_POINT ( 'NONE',  ( -5.349701230251782569, 11.76033174582461527, -25.84502411307383696 ) ) ;
#108328=PRODUCT_DEFINITION_SHAPE ( 'NONE', 'NONE',  #12014 ) ;
#108401=( GEOMETRIC_REPRESENTATION_CONTEXT ( 3 ) GLOBAL_UNCERTAINTY_ASSIGNED_CONTEXT ( ( #52074 ) ) GLOBAL_UNIT_ASSIGNED_CONTEXT ( ( #53104, #140827, #141576 ) ) REPRESENTATION_CONTEXT ( 'NONE', 'WORKASPACE' ) );
#108427=DIRECTION ( 'NONE',  ( 0.000000000000000000, 0.000000000000000000, 1.000000000000000000 ) ) ;
#108514=SPHERICAL_SURFACE ( 'NONE', #78714, 3.000000000000000000 ) ;
#108517=VERTEX_POINT ( 'NONE', #24836 ) ;
#108530=FILL_AREA_STYLE_COLOUR ( '', #34842 ) ;
#108547=EDGE_LOOP ( 'NONE', ( #92337, #142035, #34154, #33705, #91409 ) ) ;
#108634=ORIENTED_EDGE ( 'NONE', *, *, #38078, .T. ) ;
#108646=DIRECTION ( 'NONE',  ( 0.000000000000000000, 0.000000000000000000, -1.000000000000000000 ) ) ;
#108652=EDGE_CURVE ( 'NONE', #22073, #87140, #58963, .T. ) ;
#108708=ORIENTED_EDGE ( 'NONE', *, *, #35649, .F. ) ;
#108712=STYLED_ITEM ( 'NONE', ( #120502 ), #58892 ) ;
#108724=ORIENTED_EDGE ( 'NONE', *, *, #71272, .F. ) ;
#108726=UNCERTAINTY_MEASURE_WITH_UNIT (LENGTH_MEASURE( 1.000000000000000082E-05 ), #90147, 'distance_accuracy_value', 'NONE');
#108728=LINE ( 'NONE', #142135, #85554 ) ;
#108756=CARTESIAN_POINT ( 'NONE',  ( 4.609452035336649267, 11.99542526557792321, -27.26742746539979834 ) ) ;
#108771=CYLINDRICAL_SURFACE ( 'NONE', #85037, 0.5000000000000001110 ) ;
#108783=VECTOR ( 'NONE', #9397, 1000.000000000000114 ) ;
#108794=ADVANCED_FACE ( 'NONE', ( #5201 ), #18206, .F. ) ;
#108827=ORIENTED_EDGE ( 'NONE', *, *, #54979, .T. ) ;
#108844=( NAMED_UNIT ( * ) SI_UNIT ( $, .STERADIAN. ) SOLID_ANGLE_UNIT ( ) );
#108846=CARTESIAN_POINT ( 'NONE',  ( 7.140000000000044089, -1.036479131253094653E-14, -39.50000000000000000 ) ) ;
#108850=AXIS2_PLACEMENT_3D ( 'NONE', #34038, #122438, #23103 ) ;
#108897=DIRECTION ( 'NONE',  ( 1.000000000000000000, -1.248002500702738701E-15, 0.000000000000000000 ) ) ;
#108915=ORIENTED_EDGE ( 'NONE', *, *, #98719, .F. ) ;
#108959=DIRECTION ( 'NONE',  ( 0.000000000000000000, 0.000000000000000000, 1.000000000000000000 ) ) ;
#108971=CYLINDRICAL_SURFACE ( 'NONE', #93899, 0.5000000000000004441 ) ;
#109001=CIRCLE ( 'NONE', #136849, 2.552699999999997971 ) ;
#109003=STYLED_ITEM ( 'NONE', ( #20620 ), #115617 ) ;
#109013=FACE_OUTER_BOUND ( 'NONE', #74511, .T. ) ;
#109026=COLOUR_RGB ( '', 0.09019608, 0.27058824, 0.51372549) ;
#109038=CIRCLE ( 'NONE', #141458, 34.92999999999999261 ) ;
#109041=ORIENTED_EDGE ( 'NONE', *, *, #96118, .F. ) ;
#109051=CARTESIAN_POINT ( 'NONE',  ( -4.885316295235775819, 11.90249068597260873, -25.74872977259890305 ) ) ;
#109072=CARTESIAN_POINT ( 'NONE',  ( -7.140000000000001457, -39.92999999999999261, -39.50000000000000000 ) ) ;
#109089=CARTESIAN_POINT ( 'NONE',  ( 7.939999999999994174, -39.93000000000000682, -10.00000000000000178 ) ) ;
#109149=ORIENTED_EDGE ( 'NONE', *, *, #89457, .F. ) ;
#109179=SURFACE_SIDE_STYLE ('',( #76585 ) ) ;
#109211=COLOUR_RGB ( '', 0.08235294, 0.09019608, 0.10196078) ;
#109315=VECTOR ( 'NONE', #28251, 1000.000000000000000 ) ;
#109341=( NAMED_UNIT ( * ) PLANE_ANGLE_UNIT ( ) SI_UNIT ( $, .RADIAN. ) );
#109349=VERTEX_POINT ( 'NONE', #96271 ) ;
#109457=VECTOR ( 'NONE', #22753, 1000.000000000000000 ) ;
#109492=ORIENTED_EDGE ( 'NONE', *, *, #67754, .T. ) ;
#109493=EDGE_LOOP ( 'NONE', ( #11637, #47614, #87526, #53862 ) ) ;
#109507=DIRECTION ( 'NONE',  ( 0.000000000000000000, -1.000000000000000000, 0.000000000000000000 ) ) ;
#109509=CARTESIAN_POINT ( 'NONE',  ( 14.45613577907006331, 4.931321518839284046, -31.93570391306389666 ) ) ;
#109511=( GEOMETRIC_REPRESENTATION_CONTEXT ( 3 ) GLOBAL_UNCERTAINTY_ASSIGNED_CONTEXT ( ( #34434 ) ) GLOBAL_UNIT_ASSIGNED_CONTEXT ( ( #86886, #109341, #142686 ) ) REPRESENTATION_CONTEXT ( 'NONE', 'WORKASPACE' ) );
#109514=LINE ( 'NONE', #32691, #38487 ) ;
#109529=( LENGTH_UNIT ( ) NAMED_UNIT ( * ) SI_UNIT ( .MILLI., .METRE. ) );
#109581=FACE_OUTER_BOUND ( 'NONE', #109938, .T. ) ;
#109583=AXIS2_PLACEMENT_3D ( 'NONE', #115715, #70169, #125215 ) ;
#109586=DIRECTION ( 'NONE',  ( -1.000000000000000000, 0.000000000000000000, 0.000000000000000000 ) ) ;
#109600=LINE ( 'NONE', #79163, #20838 ) ;
#109666=CARTESIAN_POINT ( 'NONE',  ( -31.92499999999997584, -21.76999999999999247, -37.00000000000000000 ) ) ;
#109709=DIRECTION ( 'NONE',  ( 0.000000000000000000, -1.000000000000000000, 0.000000000000000000 ) ) ;
#109727=CARTESIAN_POINT ( 'NONE',  ( -31.92499999999997584, -7.730000000000015525, 3.180000000000000160 ) ) ;
#109782=CARTESIAN_POINT ( 'NONE',  ( 2.139883101372844543, 13.64905519538773859, -24.44323996371117147 ) ) ;
#109806=SPHERICAL_SURFACE ( 'NONE', #97875, 3.000000000000000000 ) ;
#109867=VERTEX_POINT ( 'NONE', #135058 ) ;
#109914=EDGE_CURVE ( 'NONE', #112461, #128588, #68723, .T. ) ;
#109938=EDGE_LOOP ( 'NONE', ( #9690, #11547, #140621 ) ) ;
#109962=VERTEX_POINT ( 'NONE', #48737 ) ;
#109985=UNCERTAINTY_MEASURE_WITH_UNIT (LENGTH_MEASURE( 1.000000000000000082E-05 ), #65078, 'distance_accuracy_value', 'NONE');
#110034=CARTESIAN_POINT ( 'NONE',  ( -12.20000000000000284, -28.33999999999998565, 13.17925390838734323 ) ) ;
#110120=EDGE_LOOP ( 'NONE', ( #118136, #79639, #106189, #98106 ) ) ;
#110153=CARTESIAN_POINT ( 'NONE',  ( 0.000000000000000000, -4.870000000000014317, -40.00000000000000000 ) ) ;
#110171=FILL_AREA_STYLE ('',( #120311 ) ) ;
#110180=FACE_OUTER_BOUND ( 'NONE', #79925, .T. ) ;
#110201=ADVANCED_FACE ( 'NONE', ( #53743 ), #108771, .T. ) ;
#110241=ADVANCED_FACE ( 'NONE', ( #10893 ), #13752, .T. ) ;
#110264=AXIS2_PLACEMENT_3D ( 'NONE', #66934, #98823, #143055 ) ;
#110277=CARTESIAN_POINT ( 'NONE',  ( -31.92499999999997584, 2.729999999999987104, -36.39086428169088094 ) ) ;
#110290=CARTESIAN_POINT ( 'NONE',  ( 7.939999999999994174, -35.76999999999998892, -10.00000000000000178 ) ) ;
#110330=ORIENTED_EDGE ( 'NONE', *, *, #94940, .T. ) ;
#110439=ORIENTED_EDGE ( 'NONE', *, *, #22890, .T. ) ;
#110454=EDGE_CURVE ( 'NONE', #40966, #92630, #18750, .T. ) ;
#110471=CARTESIAN_POINT ( 'NONE',  ( 15.69968023028021520, 7.023557150533521920, -28.49217588184342986 ) ) ;
#110474=ORIENTED_EDGE ( 'NONE', *, *, #84570, .T. ) ;
#110479=ORIENTED_EDGE ( 'NONE', *, *, #26066, .F. ) ;
#110490=LINE ( 'NONE', #11161, #110984 ) ;
#110491=SURFACE_STYLE_FILL_AREA ( #66322 ) ;
#110502=DIRECTION ( 'NONE',  ( 1.248002500702738701E-15, 1.000000000000000000, -0.000000000000000000 ) ) ;
#110613=DIRECTION ( 'NONE',  ( 0.000000000000000000, -1.000000000000000000, -2.242629915582281933E-16 ) ) ;
#110626=ORIENTED_EDGE ( 'NONE', *, *, #88359, .T. ) ;
#110635=MECHANICAL_DESIGN_GEOMETRIC_PRESENTATION_REPRESENTATION('',(#115276),#136121);
#110656=ORIENTED_EDGE ( 'NONE', *, *, #81922, .T. ) ;
#110663=( BOUNDED_CURVE ( )  B_SPLINE_CURVE ( 3, ( #17397, #62360, #61654, #105810 ),
 .UNSPECIFIED., .F., .T. ) 
 B_SPLINE_CURVE_WITH_KNOTS ( ( 4, 4 ),
 ( 4.712388980384689674, 6.283185307179586232 ),
 .UNSPECIFIED. ) 
 CURVE ( )  GEOMETRIC_REPRESENTATION_ITEM ( )  RATIONAL_B_SPLINE_CURVE ( ( 1.000000000000000000, 0.8047378541243649375, 0.8047378541243649375, 1.000000000000000000 ) ) 
 REPRESENTATION_ITEM ( '' )  );
#110681=CARTESIAN_POINT ( 'NONE',  ( -7.940000000000001279, -60.26999999999998892, -11.89864999999999640 ) ) ;
#110713=ADVANCED_FACE ( 'NONE', ( #34662 ), #136814, .T. ) ;
#110726=FILL_AREA_STYLE_COLOUR ( '', #98111 ) ;
#110733=DIRECTION ( 'NONE',  ( 1.049727191138614875E-16, -0.5150380749100594846, 0.8571673007021091140 ) ) ;
#110858=CARTESIAN_POINT ( 'NONE',  ( -6.639999999999999680, -25.33999999999998920, 15.47043909406156281 ) ) ;
#110869=EDGE_CURVE ( 'NONE', #55041, #56871, #36204, .T. ) ;
#110922=FILL_AREA_STYLE_COLOUR ( '', #115926 ) ;
#110939=ADVANCED_FACE ( 'NONE', ( #87448 ), #82554, .T. ) ;
#110963=CARTESIAN_POINT ( 'NONE',  ( 12.69999999999999574, -40.43000000000000682, 19.06900128115122683 ) ) ;
#110984=VECTOR ( 'NONE', #98910, 1000.000000000000000 ) ;
#110992=FILL_AREA_STYLE_COLOUR ( '', #14 ) ;
#111031=DIRECTION ( 'NONE',  ( 1.000000000000000000, 0.000000000000000000, 0.000000000000000000 ) ) ;
#111047=DIRECTION ( 'NONE',  ( -0.000000000000000000, 0.000000000000000000, -1.000000000000000000 ) ) ;
#111065=SURFACE_STYLE_FILL_AREA ( #22620 ) ;
#111098=FACE_OUTER_BOUND ( 'NONE', #122856, .T. ) ;
#111157=STYLED_ITEM ( 'NONE', ( #6350 ), #72546 ) ;
#111165=PRESENTATION_STYLE_ASSIGNMENT (( #67728 ) ) ;
#111173=COLOUR_RGB ( '', 0.31764706, 0.68627451, 0.89019608) ;
#111188=CARTESIAN_POINT ( 'NONE',  ( 13.89686957642768306, 5.764391331494414850, -29.07691927642787633 ) ) ;
#111202=CARTESIAN_POINT ( 'NONE',  ( -12.70000000000000284, -35.14999999999999147, -39.50000000000000000 ) ) ;
#111294=DIRECTION ( 'NONE',  ( -1.000000000000000000, 0.000000000000000000, 0.000000000000000000 ) ) ;
#111312=FILL_AREA_STYLE ('',( #79471 ) ) ;
#111336=PLANE ( 'NONE',  #141541 ) ;
#111374=DIRECTION ( 'NONE',  ( 1.000000000000000000, -2.496005001405478586E-15, 6.809571051365719919E-16 ) ) ;
#111406=UNCERTAINTY_MEASURE_WITH_UNIT (LENGTH_MEASURE( 1.000000000000000082E-05 ), #8051, 'distance_accuracy_value', 'NONE');
#111422=CARTESIAN_POINT ( 'NONE',  ( 19.88391014386735023, -2.827406561154159448, -34.10461866340826731 ) ) ;
#111523=COLOUR_RGB ( '', 0.72549020, 0.75294118, 0.79215686) ;
#111557=FILL_AREA_STYLE_COLOUR ( '', #55269 ) ;
#111586=ORIENTED_EDGE ( 'NONE', *, *, #96118, .T. ) ;
#111668=EDGE_CURVE ( 'NONE', #13978, #12164, #97025, .T. ) ;
#111682=ORIENTED_EDGE ( 'NONE', *, *, #27767, .T. ) ;
#111704=DIRECTION ( 'NONE',  ( 1.000000000000000000, 0.000000000000000000, 0.000000000000000000 ) ) ;
#111715=ORIENTED_EDGE ( 'NONE', *, *, #3238, .T. ) ;
#111777=VERTEX_POINT ( 'NONE', #20195 ) ;
#111784=CIRCLE ( 'NONE', #63181, 0.5000000000000004441 ) ;
#111796=PRESENTATION_STYLE_ASSIGNMENT (( #45150 ) ) ;
#111802=CARTESIAN_POINT ( 'NONE',  ( 12.19999999999999574, -22.26999999999999247, 0.000000000000000000 ) ) ;
#111883=CARTESIAN_POINT ( 'NONE',  ( 33.03650004940865870, 22.27000000000000668, -14.29932321514968763 ) ) ;
#111884=B_SPLINE_CURVE_WITH_KNOTS ( 'NONE', 3,
 ( #44159, #107247, #88382, #43433, #63775, #86235, #20947, #18805, #120228, #10768, #33313, #20221, #7921, #52161, #55036, #10072 ),
 .UNSPECIFIED., .F., .F.,
 ( 4, 2, 2, 2, 2, 2, 2, 4 ),
 ( 2.034069612461835805E-16, 0.0009871449549440356516, 0.001974289909887867907, 0.002961434864831699945, 0.003948579819775532851, 0.004935724774719364889, 0.005922869729663196928, 0.007897159639550867943 ),
 .UNSPECIFIED. ) ;
#111921=( NAMED_UNIT ( * ) SI_UNIT ( $, .STERADIAN. ) SOLID_ANGLE_UNIT ( ) );
#111966=CARTESIAN_POINT ( 'NONE',  ( -12.20000000000000107, -34.64999999999999147, 17.99210858042621908 ) ) ;
#111990=STYLED_ITEM ( 'NONE', ( #67275 ), #32540 ) ;
#112019=ORIENTED_EDGE ( 'NONE', *, *, #122457, .T. ) ;
#112051=CARTESIAN_POINT ( 'NONE',  ( -31.92499999999997584, -3.270000000000012452, -36.39086428169088094 ) ) ;
#112057=( LENGTH_UNIT ( ) NAMED_UNIT ( * ) SI_UNIT ( .MILLI., .METRE. ) );
#112093=FACE_OUTER_BOUND ( 'NONE', #9194, .T. ) ;
#112094=PRESENTATION_STYLE_ASSIGNMENT (( #67908 ) ) ;
#112100=TOROIDAL_SURFACE ( 'NONE', #119007, 3.500000000000000000, 0.5000000000000000000 ) ;
#112113=CYLINDRICAL_SURFACE ( 'NONE', #35090, 0.5000000000000004441 ) ;
#112123=CARTESIAN_POINT ( 'NONE',  ( -6.640000000000001457, -34.64999999999999147, -40.00000000000000000 ) ) ;
#112135=DIRECTION ( 'NONE',  ( 1.000000000000000000, 0.000000000000000000, 0.000000000000000000 ) ) ;
#112166=SURFACE_STYLE_FILL_AREA ( #35336 ) ;
#112238=CARTESIAN_POINT ( 'NONE',  ( 12.19999999999999574, 0.000000000000000000, -40.00000000000000000 ) ) ;
#112253=EDGE_CURVE ( 'NONE', #129025, #18833, #106138, .T. ) ;
#112264=ORIENTED_EDGE ( 'NONE', *, *, #18426, .F. ) ;
#112267=ORIENTED_EDGE ( 'NONE', *, *, #120626, .F. ) ;
#112286=AXIS2_PLACEMENT_3D ( 'NONE', #107067, #128134, #95472 ) ;
#112291=DIRECTION ( 'NONE',  ( 0.000000000000000000, -1.000000000000000000, 0.000000000000000000 ) ) ;
#112341=DIRECTION ( 'NONE',  ( 0.000000000000000000, -0.000000000000000000, 1.000000000000000000 ) ) ;
#112375=EDGE_CURVE ( 'NONE', #131250, #109962, #55137, .T. ) ;
#112392=( NAMED_UNIT ( * ) PLANE_ANGLE_UNIT ( ) SI_UNIT ( $, .RADIAN. ) );
#112438=VERTEX_POINT ( 'NONE', #98164 ) ;
#112441=EDGE_CURVE ( 'NONE', #36808, #118785, #133778, .T. ) ;
#112448=DIRECTION ( 'NONE',  ( -0.000000000000000000, 1.000000000000000000, -0.000000000000000000 ) ) ;
#112461=VERTEX_POINT ( 'NONE', #75703 ) ;
#112622=CARTESIAN_POINT ( 'NONE',  ( 17.01299345043647193, -0.9444868035624202074, -36.99999999997771738 ) ) ;
#112656=CARTESIAN_POINT ( 'NONE',  ( -12.70000000000000462, -27.68200100598810565, 15.59110741220538188 ) ) ;
#112663=STYLED_ITEM ( 'NONE', ( #98323 ), #110939 ) ;
#112676=DIRECTION ( 'NONE',  ( -0.000000000000000000, -0.000000000000000000, 1.000000000000000000 ) ) ;
#112691=PRESENTATION_STYLE_ASSIGNMENT (( #68510 ) ) ;
#112692=CARTESIAN_POINT ( 'NONE',  ( -7.940000000000007496, -32.12917598568331101, -10.00000000000000178 ) ) ;
#112703=UNCERTAINTY_MEASURE_WITH_UNIT (LENGTH_MEASURE( 1.000000000000000082E-05 ), #30024, 'distance_accuracy_value', 'NONE');
#112710=VECTOR ( 'NONE', #33094, 1000.000000000000000 ) ;
#112711=DIRECTION ( 'NONE',  ( -1.000000000000000000, 3.654646145370261567E-15, 0.000000000000000000 ) ) ;
#112721=EDGE_CURVE ( 'NONE', #25013, #132883, #62171, .T. ) ;
#112753=CARTESIAN_POINT ( 'NONE',  ( -34.92499999999997584, 22.27000000000000668, -40.00000000000000000 ) ) ;
#112754=CARTESIAN_POINT ( 'NONE',  ( -17.20366202404553135, -1.503341788956612968, -32.09416967367160112 ) ) ;
#112840=UNCERTAINTY_MEASURE_WITH_UNIT (LENGTH_MEASURE( 1.000000000000000082E-05 ), #37146, 'distance_accuracy_value', 'NONE');
#112850=CARTESIAN_POINT ( 'NONE',  ( 17.15336191800343002, -1.295666265796720840, -31.89410451029661075 ) ) ;
#112863=UNCERTAINTY_MEASURE_WITH_UNIT (LENGTH_MEASURE( 1.000000000000000082E-05 ), #130384, 'distance_accuracy_value', 'NONE');
#113056=CARTESIAN_POINT ( 'NONE',  ( 7.139999999999991687, -35.76999999999998892, -12.10072711459627293 ) ) ;
#113089=CARTESIAN_POINT ( 'NONE',  ( -12.20000000000000284, -25.33999999999998209, 15.47043909406156104 ) ) ;
#113095=MECHANICAL_DESIGN_GEOMETRIC_PRESENTATION_REPRESENTATION('',(#126957),#25122);
#113150=VECTOR ( 'NONE', #86226, 1000.000000000000000 ) ;
#113156=VERTEX_POINT ( 'NONE', #76229 ) ;
#113193=CARTESIAN_POINT ( 'NONE',  ( 5.178098103386369111, 13.15750331121097716, -24.81904025722317897 ) ) ;
#113252=ORIENTED_EDGE ( 'NONE', *, *, #49728, .T. ) ;
#113313=( NAMED_UNIT ( * ) PLANE_ANGLE_UNIT ( ) SI_UNIT ( $, .RADIAN. ) );
#113320=DIRECTION ( 'NONE',  ( -0.000000000000000000, -0.000000000000000000, -1.000000000000000000 ) ) ;
#113333=CARTESIAN_POINT ( 'NONE',  ( 15.33107836643582900, 3.532353787238777798, -29.90988538521246909 ) ) ;
#113347=SURFACE_STYLE_USAGE ( .BOTH. , #23497 ) ;
#113392=CARTESIAN_POINT ( 'NONE',  ( 7.139999999999992575, -35.14999999999999858, -40.00000000000000000 ) ) ;
#113451=CARTESIAN_POINT ( 'NONE',  ( -16.55061209249478082, 0.6983656428564303242, -33.57195050579999673 ) ) ;
#113458=VECTOR ( 'NONE', #104972, 1000.000000000000000 ) ;
#113460=MECHANICAL_DESIGN_GEOMETRIC_PRESENTATION_REPRESENTATION('',(#53231),#48592);
#113462=TOROIDAL_SURFACE ( 'NONE', #32461, 14.46000000000000085, 3.000000000000000000 ) ;
#113493=EDGE_CURVE ( 'NONE', #129328, #34178, #63067, .T. ) ;
#113508=VERTEX_POINT ( 'NONE', #63767 ) ;
#113513=DIRECTION ( 'NONE',  ( 3.115803279706882722E-16, -1.000000000000000000, 0.000000000000000000 ) ) ;
#113561=CARTESIAN_POINT ( 'NONE',  ( 16.67979525387081807, 0.3337821591035643465, -30.81818940114110461 ) ) ;
#113650=ORIENTED_EDGE ( 'NONE', *, *, #70559, .F. ) ;
#113651=( BOUNDED_CURVE ( )  B_SPLINE_CURVE ( 3, ( #129909, #19005, #50936, #139398 ),
 .UNSPECIFIED., .F., .T. ) 
 B_SPLINE_CURVE_WITH_KNOTS ( ( 4, 4 ),
 ( 1.570796326794896558, 3.141592653589793116 ),
 .UNSPECIFIED. ) 
 CURVE ( )  GEOMETRIC_REPRESENTATION_ITEM ( )  RATIONAL_B_SPLINE_CURVE ( ( 1.000000000000000000, 0.8047378541243649375, 0.8047378541243649375, 1.000000000000000000 ) ) 
 REPRESENTATION_ITEM ( '' )  );
#113673=EDGE_LOOP ( 'NONE', ( #71544, #114886, #39545, #58142 ) ) ;
#113698=DIRECTION ( 'NONE',  ( 0.000000000000000000, 0.000000000000000000, 1.000000000000000000 ) ) ;
#113699=STYLED_ITEM ( 'NONE', ( #36467 ), #98629 ) ;
#113746=EDGE_LOOP ( 'NONE', ( #134740, #21304, #111682 ) ) ;
#113779=ORIENTED_EDGE ( 'NONE', *, *, #134000, .T. ) ;
#113784=COLOUR_RGB ( '', 0.66274510, 0.83137255, 0.94901961) ;
#113802=ORIENTED_EDGE ( 'NONE', *, *, #18720, .T. ) ;
#113845=DIRECTION ( 'NONE',  ( 0.000000000000000000, 0.000000000000000000, 1.000000000000000000 ) ) ;
#113855=ORIENTED_EDGE ( 'NONE', *, *, #134132, .F. ) ;
#113866=FILL_AREA_STYLE ('',( #82000 ) ) ;
#113921=VERTEX_POINT ( 'NONE', #49868 ) ;
#113922=EDGE_LOOP ( 'NONE', ( #125223, #99278, #30426, #104849 ) ) ;
#113923=CARTESIAN_POINT ( 'NONE',  ( -10.01929040585510933, 11.35911882391357430, -26.07695017617128741 ) ) ;
#113957=ADVANCED_FACE ( 'NONE', ( #129528 ), #61478, .T. ) ;
#113996=DIRECTION ( 'NONE',  ( -1.000000000000000000, 0.000000000000000000, 0.000000000000000000 ) ) ;
#114014=CARTESIAN_POINT ( 'NONE',  ( 32.59678851739267458, 22.26999999999999957, -14.57149272626654302 ) ) ;
#114020=FACE_OUTER_BOUND ( 'NONE', #82460, .T. ) ;
#114037=SURFACE_STYLE_USAGE ( .BOTH. , #82164 ) ;
#114041=CARTESIAN_POINT ( 'NONE',  ( -6.640000000000001457, 12.19802518668052649, 4.711086268963014412 ) ) ;
#114056=CARTESIAN_POINT ( 'NONE',  ( -12.69999999999999929, -59.76999999999998892, 24.34531699603381938 ) ) ;
#114080=( NAMED_UNIT ( * ) SI_UNIT ( $, .STERADIAN. ) SOLID_ANGLE_UNIT ( ) );
#114101=EDGE_CURVE ( 'NONE', #100573, #9707, #26502, .T. ) ;
#114118=LINE ( 'NONE', #14801, #62215 ) ;
#114121=FACE_OUTER_BOUND ( 'NONE', #95622, .T. ) ;
#114149=ORIENTED_EDGE ( 'NONE', *, *, #65628, .T. ) ;
#114223=ORIENTED_EDGE ( 'NONE', *, *, #94279, .T. ) ;
#114233=CARTESIAN_POINT ( 'NONE',  ( -7.150129580834428289, 11.08364541797794800, -28.03538095272935848 ) ) ;
#114240=FACE_OUTER_BOUND ( 'NONE', #104792, .T. ) ;
#114258=VECTOR ( 'NONE', #7698, 1000.000000000000000 ) ;
#114273=UNCERTAINTY_MEASURE_WITH_UNIT (LENGTH_MEASURE( 1.000000000000000082E-05 ), #50834, 'distance_accuracy_value', 'NONE');
#114335=SURFACE_SIDE_STYLE ('',( #102041 ) ) ;
#114507=LINE ( 'NONE', #61600, #20074 ) ;
#114622=ORIENTED_EDGE ( 'NONE', *, *, #500, .F. ) ;
#114719=ADVANCED_FACE ( 'NONE', ( #138674 ), #113462, .T. ) ;
#114796=ORIENTED_EDGE ( 'NONE', *, *, #51613, .F. ) ;
#114800=DIRECTION ( 'NONE',  ( -0.000000000000000000, 0.9647414015272155474, -0.2631995976047525887 ) ) ;
#114881=ORIENTED_EDGE ( 'NONE', *, *, #9300, .T. ) ;
#114886=ORIENTED_EDGE ( 'NONE', *, *, #83980, .F. ) ;
#114908=CARTESIAN_POINT ( 'NONE',  ( -15.02522766578277746, 7.701385942161060427, -28.15899997092440898 ) ) ;
#114939=ADVANCED_FACE ( 'NONE', ( #59353, #102840, #66809 ), #26692, .T. ) ;
#114952=CARTESIAN_POINT ( 'NONE',  ( 12.19999999999999574, -21.76999999999999247, 0.000000000000000000 ) ) ;
#114960=EDGE_LOOP ( 'NONE', ( #3264, #91121, #136853, #45899 ) ) ;
#115007=ORIENTED_EDGE ( 'NONE', *, *, #4280, .T. ) ;
#115091=DIRECTION ( 'NONE',  ( 0.000000000000000000, -1.000000000000000000, 0.000000000000000000 ) ) ;
#115108=MECHANICAL_DESIGN_GEOMETRIC_PRESENTATION_REPRESENTATION('',(#133687),#29461);
#115158=DIRECTION ( 'NONE',  ( -1.000000000000000000, 0.000000000000000000, 0.000000000000000000 ) ) ;
#115244=CARTESIAN_POINT ( 'NONE',  ( 19.93618820137057668, -0.2700000000508058218, 500000.0000000000582 ) ) ;
#115276=STYLED_ITEM ( 'NONE', ( #111165 ), #93406 ) ;
#115280=ORIENTED_EDGE ( 'NONE', *, *, #85715, .F. ) ;
#115301=CARTESIAN_POINT ( 'NONE',  ( -14.86926710130653717, 7.855190979727734835, -28.08282898950776385 ) ) ;
#115328=VERTEX_POINT ( 'NONE', #3312 ) ;
#115342=CARTESIAN_POINT ( 'NONE',  ( -13.41477511890566454, 6.314159094412498341, -31.22869265677382344 ) ) ;
#115366=STYLED_ITEM ( 'NONE', ( #65472 ), #38349 ) ;
#115371=ORIENTED_EDGE ( 'NONE', *, *, #40855, .T. ) ;
#115374=DIRECTION ( 'NONE',  ( -0.000000000000000000, -0.000000000000000000, -1.000000000000000000 ) ) ;
#115434=DIRECTION ( 'NONE',  ( 0.000000000000000000, 0.000000000000000000, -1.000000000000000000 ) ) ;
#115503=FILL_AREA_STYLE_COLOUR ( '', #73888 ) ;
#115563=FILL_AREA_STYLE ('',( #126468 ) ) ;
#115594=AXIS2_PLACEMENT_3D ( 'NONE', #104914, #5582, #62143 ) ;
#115604=AXIS2_PLACEMENT_3D ( 'NONE', #83939, #139742, #40420 ) ;
#115614=CARTESIAN_POINT ( 'NONE',  ( -15.70492293426981334, 6.989513400225817463, -28.49959148306838230 ) ) ;
#115617=ADVANCED_FACE ( 'NONE', ( #98894 ), #16478, .T. ) ;
#115685=ORIENTED_EDGE ( 'NONE', *, *, #23055, .F. ) ;
#115715=CARTESIAN_POINT ( 'NONE',  ( 12.69999999999999574, 0.000000000000000000, -40.00000000000000000 ) ) ;
#115721=CARTESIAN_POINT ( 'NONE',  ( 7.939999999999994174, -60.26999999999998892, -10.00000000000000178 ) ) ;
#115764=( NAMED_UNIT ( * ) PLANE_ANGLE_UNIT ( ) SI_UNIT ( $, .RADIAN. ) );
#115765=ORIENTED_EDGE ( 'NONE', *, *, #136290, .F. ) ;
#115785=( BOUNDED_CURVE ( )  B_SPLINE_CURVE ( 3, ( #64199, #139647, #107679, #117819 ),
 .UNSPECIFIED., .F., .F. ) 
 B_SPLINE_CURVE_WITH_KNOTS ( ( 4, 4 ),
 ( 0.2663372438543387677, 1.570796326794899667 ),
 .UNSPECIFIED. ) 
 CURVE ( )  GEOMETRIC_REPRESENTATION_ITEM ( )  RATIONAL_B_SPLINE_CURVE ( ( 1.000000000000000000, 0.8631550219135049051, 0.8631550219135049051, 1.000000000000000000 ) ) 
 REPRESENTATION_ITEM ( '' )  );
#115811=STYLED_ITEM ( 'NONE', ( #77805 ), #141893 ) ;
#115926=COLOUR_RGB ( '', 0.72549020, 0.75294118, 0.79215686) ;
#115944=AXIS2_PLACEMENT_3D ( 'NONE', #123318, #23982, #68246 ) ;
#115955=EDGE_LOOP ( 'NONE', ( #16484, #118998, #2737, #49126 ) ) ;
#116024=DIRECTION ( 'NONE',  ( -1.000000000000000000, 1.451651444332056451E-15, 0.000000000000000000 ) ) ;
#116027=AXIS2_PLACEMENT_3D ( 'NONE', #141357, #10818, #88429 ) ;
#116040=AXIS2_PLACEMENT_3D ( 'NONE', #110153, #55819, #94112 ) ;
#116086=DIRECTION ( 'NONE',  ( 0.000000000000000000, 0.000000000000000000, 1.000000000000000000 ) ) ;
#116090=CARTESIAN_POINT ( 'NONE',  ( -16.15228161756845893, 1.822542437158885642, -33.22373175091470188 ) ) ;
#116201=ORIENTED_EDGE ( 'NONE', *, *, #118976, .T. ) ;
#116224=CARTESIAN_POINT ( 'NONE',  ( -12.19999999999999929, -59.76999999999998892, -40.00000000000000000 ) ) ;
#116256=TOROIDAL_SURFACE ( 'NONE', #56071, 9.000000000000001776, 3.000000000000000000 ) ;
#116282=DIRECTION ( 'NONE',  ( 0.000000000000000000, -1.000000000000000000, -2.312964634635742661E-15 ) ) ;
#116317=VECTOR ( 'NONE', #101873, 1000.000000000000000 ) ;
#116335=SURFACE_STYLE_USAGE ( .BOTH. , #127946 ) ;
#116377=VECTOR ( 'NONE', #94482, 1000.000000000000000 ) ;
#116382=ORIENTED_EDGE ( 'NONE', *, *, #64691, .T. ) ;
#116412=AXIS2_PLACEMENT_3D ( 'NONE', #44985, #46403, #79756 ) ;
#116424=FACE_OUTER_BOUND ( 'NONE', #114960, .T. ) ;
#116478=DIRECTION ( 'NONE',  ( 1.000000000000000000, 0.000000000000000000, 0.000000000000000000 ) ) ;
#116525=EDGE_LOOP ( 'NONE', ( #97287, #4300, #47591, #79891 ) ) ;
#116540=DIRECTION ( 'NONE',  ( 0.000000000000000000, 0.000000000000000000, -1.000000000000000000 ) ) ;
#116717=CIRCLE ( 'NONE', #14881, 0.5000000000000004441 ) ;
#116718=ORIENTED_EDGE ( 'NONE', *, *, #8938, .F. ) ;
#116726=FILL_AREA_STYLE ('',( #60973 ) ) ;
#116763=CARTESIAN_POINT ( 'NONE',  ( 12.49289321881344605, -60.26999999999998892, 25.00000000000000000 ) ) ;
#116773=CARTESIAN_POINT ( 'NONE',  ( -3.684382248798170334, 13.44380610198669324, -24.60099495244268653 ) ) ;
#116824=VERTEX_POINT ( 'NONE', #34705 ) ;
#116835=EDGE_CURVE ( 'NONE', #25909, #92341, #129813, .T. ) ;
#116839=DIRECTION ( 'NONE',  ( 1.000000000000000000, 0.000000000000000000, 0.000000000000000000 ) ) ;
#116843=DIRECTION ( 'NONE',  ( 0.000000000000000000, -2.242629915582283412E-16, 1.000000000000000000 ) ) ;
#116860=CYLINDRICAL_SURFACE ( 'NONE', #87223, 0.5000000000000000000 ) ;
#116871=CARTESIAN_POINT ( 'NONE',  ( 7.139999999999992575, -35.14999999999999858, -39.50000000000000000 ) ) ;
#116894=DIRECTION ( 'NONE',  ( 0.000000000000000000, 0.9647414015272156584, -0.2631995976047526442 ) ) ;
#116939=ADVANCED_FACE ( 'NONE', ( #72366 ), #50565, .T. ) ;
#116962=EDGE_CURVE ( 'NONE', #36342, #97431, #138295, .T. ) ;
#116963=ORIENTED_EDGE ( 'NONE', *, *, #33306, .F. ) ;
#117029=COLOUR_RGB ( '', 0.31764706, 0.68627451, 0.89019608) ;
#117056=( NAMED_UNIT ( * ) SI_UNIT ( $, .STERADIAN. ) SOLID_ANGLE_UNIT ( ) );
#117060=ORIENTED_EDGE ( 'NONE', *, *, #55753, .F. ) ;
#117071=CARTESIAN_POINT ( 'NONE',  ( -16.42533615676552117, 1.154938085476876264, -30.62621587217987340 ) ) ;
#117109=CARTESIAN_POINT ( 'NONE',  ( -34.89799234656373983, 22.27000000000001023, -9.122257832017591994 ) ) ;
#117118=MECHANICAL_DESIGN_GEOMETRIC_PRESENTATION_REPRESENTATION('',(#121772),#84747);
#117171=( GEOMETRIC_REPRESENTATION_CONTEXT ( 3 ) GLOBAL_UNCERTAINTY_ASSIGNED_CONTEXT ( ( #56237 ) ) GLOBAL_UNIT_ASSIGNED_CONTEXT ( ( #14893, #25771, #117056 ) ) REPRESENTATION_CONTEXT ( 'NONE', 'WORKASPACE' ) );
#117207=FACE_OUTER_BOUND ( 'NONE', #73589, .T. ) ;
#117227=( NAMED_UNIT ( * ) SI_UNIT ( $, .STERADIAN. ) SOLID_ANGLE_UNIT ( ) );
#117228=AXIS2_PLACEMENT_3D ( 'NONE', #117955, #118702, #141160 ) ;
#117248=FACE_OUTER_BOUND ( 'NONE', #32908, .T. ) ;
#117264=VERTEX_POINT ( 'NONE', #80201 ) ;
#117287=CARTESIAN_POINT ( 'NONE',  ( -7.140000000000001457, -35.76999999999998892, -12.10072711459627293 ) ) ;
#117318=FACE_OUTER_BOUND ( 'NONE', #31038, .T. ) ;
#117423=VERTEX_POINT ( 'NONE', #25778 ) ;
#117471=VECTOR ( 'NONE', #61641, 1000.000000000000000 ) ;
#117477=EDGE_CURVE ( 'NONE', #30341, #40406, #85154, .T. ) ;
#117481=DIRECTION ( 'NONE',  ( 1.000000000000000000, 0.000000000000000000, 0.000000000000000000 ) ) ;
#117511=DIRECTION ( 'NONE',  ( 1.000000000000000000, 0.000000000000000000, 6.938893903907222067E-15 ) ) ;
#117639=EDGE_CURVE ( 'NONE', #38181, #22073, #90609, .T. ) ;
#117692=CARTESIAN_POINT ( 'NONE',  ( -16.93298150401930258, -0.6090650756136195554, -34.87030803381578181 ) ) ;
#117712=ORIENTED_EDGE ( 'NONE', *, *, #54703, .T. ) ;
#117725=CARTESIAN_POINT ( 'NONE',  ( 0.000000000000000000, 0.000000000000000000, -40.00000000000000000 ) ) ;
#117763=CARTESIAN_POINT ( 'NONE',  ( 11.43556760655506821, 8.373926597364643953, -27.85776518686094860 ) ) ;
#117793=ADVANCED_FACE ( 'NONE', ( #126351 ), #4964, .F. ) ;
#117803=SURFACE_STYLE_USAGE ( .BOTH. , #98243 ) ;
#117819=CARTESIAN_POINT ( 'NONE',  ( -6.640000000000001457, -40.29840020119761590, 19.55137198191482995 ) ) ;
#117910=SURFACE_STYLE_USAGE ( .BOTH. , #73727 ) ;
#117955=CARTESIAN_POINT ( 'NONE',  ( 0.000000000000000000, -21.76999999999999247, -39.50000000000000000 ) ) ;
#117967=EDGE_LOOP ( 'NONE', ( #51615, #72738, #77417, #69329, #106126, #92690, #50440, #126519 ) ) ;
#117975=DIRECTION ( 'NONE',  ( 3.115803279706882722E-16, -1.000000000000000000, 0.000000000000000000 ) ) ;
#118029=DIRECTION ( 'NONE',  ( 3.469446951953611033E-15, 0.000000000000000000, 1.000000000000000000 ) ) ;
#118044=VECTOR ( 'NONE', #11033, 1000.000000000000000 ) ;
#118080=LINE ( 'NONE', #18790, #72687 ) ;
#118136=ORIENTED_EDGE ( 'NONE', *, *, #95890, .T. ) ;
#118165=VECTOR ( 'NONE', #102326, 1000.000000000000000 ) ;
#118192=DIRECTION ( 'NONE',  ( -0.000000000000000000, 0.000000000000000000, 1.000000000000000000 ) ) ;
#118205=DIRECTION ( 'NONE',  ( -0.8571673007021118895, 0.000000000000000000, -0.5150380749100549327 ) ) ;
#118219=CARTESIAN_POINT ( 'NONE',  ( -11.61648642849997337, 8.193565109092823207, -30.12529094710442124 ) ) ;
#118347=EDGE_CURVE ( 'NONE', #89560, #71785, #135315, .T. ) ;
#118356=CARTESIAN_POINT ( 'NONE',  ( 31.92500000000001492, -6.269999999999992468, -40.00000000000000000 ) ) ;
#118365=LINE ( 'NONE', #107500, #80630 ) ;
#118369=ORIENTED_EDGE ( 'NONE', *, *, #9084, .T. ) ;
#118398=VECTOR ( 'NONE', #49434, 1000.000000000000000 ) ;
#118457=VERTEX_POINT ( 'NONE', #112123 ) ;
#118458=COLOUR_RGB ( '', 0.09019608, 0.27058824, 0.51372549) ;
#118466=( NAMED_UNIT ( * ) SI_UNIT ( $, .STERADIAN. ) SOLID_ANGLE_UNIT ( ) );
#118508=CARTESIAN_POINT ( 'NONE',  ( 13.33798170103910685, 6.458498716420526975, -28.77788784152867052 ) ) ;
#118530=COLOUR_RGB ( '', 0.40784314, 0.44705882, 0.49803922) ;
#118531=COLOUR_RGB ( '', 0.66274510, 0.83137255, 0.94901961) ;
#118539=DIRECTION ( 'NONE',  ( 0.000000000000000000, -0.2631995976047483699, -0.9647414015272167687 ) ) ;
#118551=DIRECTION ( 'NONE',  ( 1.000000000000000000, 0.000000000000000000, -0.000000000000000000 ) ) ;
#118556=CIRCLE ( 'NONE', #115944, 0.5000000000000013323 ) ;
#118565=AXIS2_PLACEMENT_3D ( 'NONE', #50859, #29801, #117511 ) ;
#118671=VERTEX_POINT ( 'NONE', #40976 ) ;
#118682=DIRECTION ( 'NONE',  ( -3.166071393695993333E-32, 1.016133275908817741E-16, -1.000000000000000000 ) ) ;
#118702=DIRECTION ( 'NONE',  ( -1.000000000000000000, 0.000000000000000000, 0.000000000000000000 ) ) ;
#118732=ORIENTED_EDGE ( 'NONE', *, *, #67255, .F. ) ;
#118767=DIRECTION ( 'NONE',  ( -1.000000000000000000, 0.000000000000000000, 0.000000000000000000 ) ) ;
#118782=CARTESIAN_POINT ( 'NONE',  ( 12.19999999999999574, -25.33999999999998565, 3.000000000000002665 ) ) ;
#118785=VERTEX_POINT ( 'NONE', #77202 ) ;
#118843=PRESENTATION_STYLE_ASSIGNMENT (( #86237 ) ) ;
#118892=VERTEX_POINT ( 'NONE', #100358 ) ;
#118941=DIRECTION ( 'NONE',  ( 1.000000000000000000, -0.000000000000000000, -0.000000000000000000 ) ) ;
#118970=SURFACE_STYLE_FILL_AREA ( #18199 ) ;
#118975=VECTOR ( 'NONE', #14681, 1000.000000000000000 ) ;
#118976=EDGE_CURVE ( 'NONE', #68517, #131359, #91615, .T. ) ;
#118995=EDGE_LOOP ( 'NONE', ( #96164, #24908, #60577, #32986 ) ) ;
#118998=ORIENTED_EDGE ( 'NONE', *, *, #40600, .F. ) ;
#119007=AXIS2_PLACEMENT_3D ( 'NONE', #102162, #93408, #38322 ) ;
#119035=DIRECTION ( 'NONE',  ( 1.451651444332056451E-15, 1.000000000000000000, -0.000000000000000000 ) ) ;
#119043=ORIENTED_EDGE ( 'NONE', *, *, #56233, .F. ) ;
#119110=( LENGTH_UNIT ( ) NAMED_UNIT ( * ) SI_UNIT ( .MILLI., .METRE. ) );
#119133=VECTOR ( 'NONE', #95672, 1000.000000000000000 ) ;
#119158=DIRECTION ( 'NONE',  ( 0.000000000000000000, -1.000000000000000000, 0.000000000000000000 ) ) ;
#119218=CARTESIAN_POINT ( 'NONE',  ( 0.4979396410360854008, 13.74659983411467756, -24.36742386311884090 ) ) ;
#119262=CARTESIAN_POINT ( 'NONE',  ( -31.92499999999997584, -3.270000000000012452, -36.39086428169088094 ) ) ;
#119304=DIRECTION ( 'NONE',  ( 0.000000000000000000, 1.016133275908817741E-16, -1.000000000000000000 ) ) ;
#119373=DIRECTION ( 'NONE',  ( 0.000000000000000000, 0.000000000000000000, -1.000000000000000000 ) ) ;
#119417=CARTESIAN_POINT ( 'NONE',  ( 31.92500000000001492, 9.947201970464227326E-15, -40.00000000000000000 ) ) ;
#119435=VERTEX_POINT ( 'NONE', #25453 ) ;
#119458=LINE ( 'NONE', #131801, #62504 ) ;
#119459=FILL_AREA_STYLE ('',( #85409 ) ) ;
#119471=CARTESIAN_POINT ( 'NONE',  ( -7.056846916127231314E-14, -40.42999999999999261, 19.06900128115122328 ) ) ;
#119484=CIRCLE ( 'NONE', #52346, 0.5000000000000000000 ) ;
#119592=DIRECTION ( 'NONE',  ( 1.000000000000000000, 0.000000000000000000, 0.000000000000000000 ) ) ;
#119677=DIRECTION ( 'NONE',  ( -0.000000000000000000, -1.000000000000000000, -0.000000000000000000 ) ) ;
#119771=ORIENTED_EDGE ( 'NONE', *, *, #96276, .F. ) ;
#119772=EDGE_LOOP ( 'NONE', ( #30585, #106954, #117060, #39203 ) ) ;
#119847=FILL_AREA_STYLE ('',( #141650 ) ) ;
#119855=DIRECTION ( 'NONE',  ( 0.000000000000000000, 0.000000000000000000, 1.000000000000000000 ) ) ;
#119866=AXIS2_PLACEMENT_3D ( 'NONE', #141674, #120592, #54671 ) ;
#119890=EDGE_CURVE ( 'NONE', #115328, #125503, #47440, .T. ) ;
#119903=ORIENTED_EDGE ( 'NONE', *, *, #102563, .T. ) ;
#119911=CARTESIAN_POINT ( 'NONE',  ( 8.807295529226077946, 11.91728907476091237, -25.70178564786368725 ) ) ;
#119945=ORIENTED_EDGE ( 'NONE', *, *, #31078, .T. ) ;
#119957=CARTESIAN_POINT ( 'NONE',  ( 31.92500000000001492, -6.269999999999992468, -36.39086428169088094 ) ) ;
#119968=EDGE_LOOP ( 'NONE', ( #83068, #4502 ) ) ;
#120002=COLOUR_RGB ( '', 0.08235294, 0.09019608, 0.10196078) ;
#120019=( LENGTH_UNIT ( ) NAMED_UNIT ( * ) SI_UNIT ( .MILLI., .METRE. ) );
#120041=ORIENTED_EDGE ( 'NONE', *, *, #129034, .T. ) ;
#120108=SURFACE_STYLE_FILL_AREA ( #75934 ) ;
#120132=ORIENTED_EDGE ( 'NONE', *, *, #34003, .T. ) ;
#120146=DIRECTION ( 'NONE',  ( 0.000000000000000000, 0.000000000000000000, -1.000000000000000000 ) ) ;
#120206=CIRCLE ( 'NONE', #78560, 3.000000000000000444 ) ;
#120221=ORIENTED_EDGE ( 'NONE', *, *, #61881, .F. ) ;
#120228=CARTESIAN_POINT ( 'NONE',  ( 19.80737797471735107, -2.215184370838247929, -32.97705054010764769 ) ) ;
#120240=SURFACE_STYLE_FILL_AREA ( #140597 ) ;
#120311=FILL_AREA_STYLE_COLOUR ( '', #13698 ) ;
#120322=CARTESIAN_POINT ( 'NONE',  ( -7.140000000000001457, -35.76999999999998892, -12.10072711459627293 ) ) ;
#120337=CARTESIAN_POINT ( 'NONE',  ( 12.69999999999999574, -22.33999999999998565, -0.5000000000000004441 ) ) ;
#120338=EDGE_CURVE ( 'NONE', #34379, #72776, #79923, .T. ) ;
#120455=CIRCLE ( 'NONE', #136731, 0.5000000000000013323 ) ;
#120478=ORIENTED_EDGE ( 'NONE', *, *, #28653, .F. ) ;
#120502=PRESENTATION_STYLE_ASSIGNMENT (( #121248 ) ) ;
#120503=FACE_OUTER_BOUND ( 'NONE', #100097, .T. ) ;
#120535=EDGE_CURVE ( 'NONE', #95348, #118892, #65330, .T. ) ;
#120537=VERTEX_POINT ( 'NONE', #87763 ) ;
#120547=CARTESIAN_POINT ( 'NONE',  ( 12.69999999999999574, -35.15000000000000568, 17.49210858042622618 ) ) ;
#120553=DIRECTION ( 'NONE',  ( 0.000000000000000000, -0.9647414015272155474, 0.2631995976047525887 ) ) ;
#120555=LINE ( 'NONE', #88701, #2290 ) ;
#120582=AXIS2_PLACEMENT_3D ( 'NONE', #76508, #66345, #37075 ) ;
#120592=DIRECTION ( 'NONE',  ( -1.000000000000000000, 0.000000000000000000, 3.596245529072721644E-15 ) ) ;
#120626=EDGE_CURVE ( 'NONE', #64363, #97358, #55875, .T. ) ;
#120634=CARTESIAN_POINT ( 'NONE',  ( -1.881878777429229599, 12.51266495272427193, -26.80546393447896847 ) ) ;
#120694=COLOUR_RGB ( '', 0.72549020, 0.75294118, 0.79215686) ;
#120783=ORIENTED_EDGE ( 'NONE', *, *, #44063, .F. ) ;
#120810=EDGE_CURVE ( 'NONE', #86478, #71183, #105738, .T. ) ;
#120815=DIRECTION ( 'NONE',  ( 1.000000000000000000, 0.000000000000000000, 0.000000000000000000 ) ) ;
#120867=EDGE_LOOP ( 'NONE', ( #90130, #30893, #65315, #101490 ) ) ;
#120910=AXIS2_PLACEMENT_3D ( 'NONE', #61237, #93097, #126421 ) ;
#120935=ORIENTED_EDGE ( 'NONE', *, *, #6099, .T. ) ;
#120971=AXIS2_PLACEMENT_3D ( 'NONE', #17193, #73036, #4829 ) ;
#121021=DIRECTION ( 'NONE',  ( 1.000000000000000000, 3.115803279706882722E-16, -0.000000000000000000 ) ) ;
#121072=EDGE_LOOP ( 'NONE', ( #59248, #10749, #23883, #92036 ) ) ;
#121103=DIRECTION ( 'NONE',  ( -1.000000000000000000, 0.000000000000000000, 0.000000000000000000 ) ) ;
#121166=( NAMED_UNIT ( * ) PLANE_ANGLE_UNIT ( ) SI_UNIT ( $, .RADIAN. ) );
#121180=PLANE ( 'NONE',  #139306 ) ;
#121201=B_SPLINE_CURVE_WITH_KNOTS ( 'NONE', 3,
 ( #81544, #6049, #103250, #93813 ),
 .UNSPECIFIED., .F., .F.,
 ( 4, 4 ),
 ( 0.001201692628195026894, 0.001634763834691506899 ),
 .UNSPECIFIED. ) ;
#121248=SURFACE_STYLE_USAGE ( .BOTH. , #10339 ) ;
#121260=TOROIDAL_SURFACE ( 'NONE', #139825, 2.500000000000000000, 0.5000000000000000000 ) ;
#121276=DIRECTION ( 'NONE',  ( -1.321231229586337907E-16, 0.9647414015272155474, -0.2631995976047525887 ) ) ;
#121294=CARTESIAN_POINT ( 'NONE',  ( 12.19999999999999574, 0.000000000000000000, -39.50000000000000000 ) ) ;
#121304=CYLINDRICAL_SURFACE ( 'NONE', #103219, 0.5000000000000004441 ) ;
#121310=ORIENTED_EDGE ( 'NONE', *, *, #108652, .F. ) ;
#121385=FILL_AREA_STYLE_COLOUR ( '', #35413 ) ;
#121393=DIRECTION ( 'NONE',  ( 0.000000000000000000, -0.9647414015272164356, 0.2631995976047502017 ) ) ;
#121427=DIRECTION ( 'NONE',  ( 0.000000000000000000, 0.000000000000000000, 1.000000000000000000 ) ) ;
#121431=SURFACE_STYLE_USAGE ( .BOTH. , #34433 ) ;
#121503=CARTESIAN_POINT ( 'NONE',  ( -12.20000000000000284, -25.83999999999998565, -1.121314957791154772E-16 ) ) ;
#121504=VERTEX_POINT ( 'NONE', #56270 ) ;
#121535=ORIENTED_EDGE ( 'NONE', *, *, #127854, .F. ) ;
#121574=FACE_OUTER_BOUND ( 'NONE', #81959, .T. ) ;
#121607=ORIENTED_EDGE ( 'NONE', *, *, #75237, .T. ) ;
#121669=EDGE_LOOP ( 'NONE', ( #142034, #14989, #102450, #5383 ) ) ;
#121697=DIRECTION ( 'NONE',  ( -1.369518533665900312E-16, 1.000000000000000000, -0.000000000000000000 ) ) ;
#121706=ORIENTED_EDGE ( 'NONE', *, *, #70559, .T. ) ;
#121716=CARTESIAN_POINT ( 'NONE',  ( -12.70000000000000284, -40.29840020119761590, 19.55137198191482995 ) ) ;
#121723=SURFACE_STYLE_FILL_AREA ( #55798 ) ;
#121736=CARTESIAN_POINT ( 'NONE',  ( 16.64450715494396604, 0.4096876026223312262, -33.72258372513044122 ) ) ;
#121772=STYLED_ITEM ( 'NONE', ( #30515 ), #133817 ) ;
#121789=EDGE_CURVE ( 'NONE', #98685, #113921, #32904, .T. ) ;
#121803=EDGE_CURVE ( 'NONE', #92723, #61905, #17650, .T. ) ;
#121880=SURFACE_STYLE_FILL_AREA ( #101567 ) ;
#121924=CIRCLE ( 'NONE', #87291, 5.999999999999998224 ) ;
#121925=DIRECTION ( 'NONE',  ( -1.000000000000000000, -1.369518533665900312E-16, 0.000000000000000000 ) ) ;
#121951=( GEOMETRIC_REPRESENTATION_CONTEXT ( 3 ) GLOBAL_UNCERTAINTY_ASSIGNED_CONTEXT ( ( #12664 ) ) GLOBAL_UNIT_ASSIGNED_CONTEXT ( ( #120019, #132408, #65731 ) ) REPRESENTATION_CONTEXT ( 'NONE', 'WORKASPACE' ) );
#121974=VECTOR ( 'NONE', #110733, 999.9999999999998863 ) ;
#122014=CARTESIAN_POINT ( 'NONE',  ( 34.92500000000001137, 22.27000000000001023, -8.436784469852378621 ) ) ;
#122040=EDGE_CURVE ( 'NONE', #64319, #104775, #142780, .T. ) ;
#122086=CYLINDRICAL_SURFACE ( 'NONE', #117228, 0.5000000000000004441 ) ;
#122111=DIRECTION ( 'NONE',  ( -3.973028287378889149E-16, 1.000000000000000000, 0.000000000000000000 ) ) ;
#122121=CARTESIAN_POINT ( 'NONE',  ( 12.49289321881344783, -34.80096641561354431, 18.05156865852269732 ) ) ;
#122182=ORIENTED_EDGE ( 'NONE', *, *, #62862, .F. ) ;
#122184=CARTESIAN_POINT ( 'NONE',  ( -19.83193850628799737, -2.400066657216377575, -33.20899412005067575 ) ) ;
#122191=ORIENTED_EDGE ( 'NONE', *, *, #43480, .T. ) ;
#122206=( NAMED_UNIT ( * ) SI_UNIT ( $, .STERADIAN. ) SOLID_ANGLE_UNIT ( ) );
#122212=EDGE_CURVE ( 'NONE', #34178, #78214, #97964, .T. ) ;
#122255=AXIS2_PLACEMENT_3D ( 'NONE', #105442, #6100, #106875 ) ;
#122266=CARTESIAN_POINT ( 'NONE',  ( -32.26821726222483733, 22.27000000000000313, -14.68217205629616018 ) ) ;
#122284=CARTESIAN_POINT ( 'NONE',  ( 16.90050536373548340, -0.4844931144635390985, -34.66719912185458696 ) ) ;
#122300=FACE_OUTER_BOUND ( 'NONE', #109493, .T. ) ;
#122313=VERTEX_POINT ( 'NONE', #133453 ) ;
#122356=CARTESIAN_POINT ( 'NONE',  ( -12.19999999999999929, -59.76999999999998892, -39.50000000000000000 ) ) ;
#122391=CIRCLE ( 'NONE', #22822, 2.999999999999999112 ) ;
#122438=DIRECTION ( 'NONE',  ( -0.000000000000000000, -0.000000000000000000, 1.000000000000000000 ) ) ;
#122457=EDGE_CURVE ( 'NONE', #63324, #64204, #130966, .T. ) ;
#122458=PLANE ( 'NONE',  #69841 ) ;
#122487=VECTOR ( 'NONE', #121276, 1000.000000000000114 ) ;
#122490=EDGE_LOOP ( 'NONE', ( #78891, #24363, #18564 ) ) ;
#122515=CARTESIAN_POINT ( 'NONE',  ( -34.92499999999999716, 22.26999999999998181, -14.71147562388301822 ) ) ;
#122541=VERTEX_POINT ( 'NONE', #9871 ) ;
#122554=CARTESIAN_POINT ( 'NONE',  ( 7.139999999999985469, -40.06159979880239064, 18.96849477799998596 ) ) ;
#122593=DIRECTION ( 'NONE',  ( 0.000000000000000000, 0.000000000000000000, 1.000000000000000000 ) ) ;
#122607=AXIS2_PLACEMENT_3D ( 'NONE', #5131, #38519, #7283 ) ;
#122649=CARTESIAN_POINT ( 'NONE',  ( 10.87659042482644800, 10.89112078991403898, -26.37954615677881520 ) ) ;
#122658=CARTESIAN_POINT ( 'NONE',  ( 31.92500000000001492, -6.269999999999992468, -37.00000000000000000 ) ) ;
#122677=COLOUR_RGB ( '', 0.08235294, 0.09019608, 0.10196078) ;
#122744=CARTESIAN_POINT ( 'NONE',  ( 34.74723349734966149, 22.27000000000000313, -10.47243126915188860 ) ) ;
#122775=DIRECTION ( 'NONE',  ( -0.000000000000000000, -0.000000000000000000, -1.000000000000000000 ) ) ;
#122777=( NAMED_UNIT ( * ) PLANE_ANGLE_UNIT ( ) SI_UNIT ( $, .RADIAN. ) );
#122801=CARTESIAN_POINT ( 'NONE',  ( 16.15294014157827718, 1.820683936599848396, -33.22430742917087088 ) ) ;
#122832=ORIENTED_EDGE ( 'NONE', *, *, #102603, .T. ) ;
#122856=EDGE_LOOP ( 'NONE', ( #105120, #95739, #74219, #59357 ) ) ;
#122917=LINE ( 'NONE', #112051, #112710 ) ;
#122925=CARTESIAN_POINT ( 'NONE',  ( -19.87087987052762372, -2.718579257641874580, -33.78996532117428586 ) ) ;
#122959=PLANE ( 'NONE',  #103303 ) ;
#122974=ORIENTED_EDGE ( 'NONE', *, *, #44682, .F. ) ;
#122997=( GEOMETRIC_REPRESENTATION_CONTEXT ( 3 ) GLOBAL_UNCERTAINTY_ASSIGNED_CONTEXT ( ( #63533 ) ) GLOBAL_UNIT_ASSIGNED_CONTEXT ( ( #98576, #101432, #142802 ) ) REPRESENTATION_CONTEXT ( 'NONE', 'WORKASPACE' ) );
#123035=CARTESIAN_POINT ( 'NONE',  ( 16.92059731686079971, -0.5630473312367980654, -34.80677428804649765 ) ) ;
#123093=ORIENTED_EDGE ( 'NONE', *, *, #31923, .F. ) ;
#123120=VECTOR ( 'NONE', #7667, 1000.000000000000000 ) ;
#123138=ORIENTED_EDGE ( 'NONE', *, *, #40430, .T. ) ;
#123189=ORIENTED_EDGE ( 'NONE', *, *, #49320, .T. ) ;
#123218=DIRECTION ( 'NONE',  ( -1.451651444332056451E-15, -1.000000000000000000, 0.000000000000000000 ) ) ;
#123235=CARTESIAN_POINT ( 'NONE',  ( -31.92499999999997584, -6.270000000000012008, -37.00000000000000000 ) ) ;
#123245=DIRECTION ( 'NONE',  ( -1.000000000000000000, -0.000000000000000000, -0.000000000000000000 ) ) ;
#123318=CARTESIAN_POINT ( 'NONE',  ( -12.20000000000000284, -40.42999999999999261, 19.06900128115121973 ) ) ;
#123347=DIRECTION ( 'NONE',  ( -1.000000000000000000, 0.000000000000000000, 0.000000000000000000 ) ) ;
#123386=VECTOR ( 'NONE', #137504, 1000.000000000000000 ) ;
#123390=CARTESIAN_POINT ( 'NONE',  ( 17.01299345042646749, -0.9444868035190615574, -36.07446264259789359 ) ) ;
#123407=AXIS2_PLACEMENT_3D ( 'NONE', #119471, #64407, #97751 ) ;
#123413=CARTESIAN_POINT ( 'NONE',  ( -34.92499999999999005, -3.270000000000012896, -40.00000000000000000 ) ) ;
#123443=EDGE_CURVE ( 'NONE', #117264, #79752, #111884, .T. ) ;
#123474=CARTESIAN_POINT ( 'NONE',  ( 17.01299345043647193, -0.9444868035624202074, 500000.0000000000582 ) ) ;
#123529=CARTESIAN_POINT ( 'NONE',  ( 7.060677813783885703, -39.92999999999999261, 19.30339710675712794 ) ) ;
#123538=DIRECTION ( 'NONE',  ( 0.000000000000000000, 0.000000000000000000, 1.000000000000000000 ) ) ;
#123568=( LENGTH_UNIT ( ) NAMED_UNIT ( * ) SI_UNIT ( .MILLI., .METRE. ) );
#123609=PLANE ( 'NONE',  #9044 ) ;
#123669=PRESENTATION_STYLE_ASSIGNMENT (( #59140 ) ) ;
#123689=CARTESIAN_POINT ( 'NONE',  ( 31.92500000000002203, -21.76999999999999247, -37.00000000000000000 ) ) ;
#123749=EDGE_LOOP ( 'NONE', ( #134249, #77460, #90454, #129545 ) ) ;
#123763=CARTESIAN_POINT ( 'NONE',  ( 17.20358538138344429, -1.503029704422955248, -32.09388084135276387 ) ) ;
#123781=AXIS2_PLACEMENT_3D ( 'NONE', #40480, #41161, #126727 ) ;
#123811=DIRECTION ( 'NONE',  ( -0.000000000000000000, -0.000000000000000000, -1.000000000000000000 ) ) ;
#123891=DIRECTION ( 'NONE',  ( 1.000000000000000000, 0.000000000000000000, 0.000000000000000000 ) ) ;
#123916=EDGE_LOOP ( 'NONE', ( #76272, #27431, #65394 ) ) ;
#123987=( GEOMETRIC_REPRESENTATION_CONTEXT ( 3 ) GLOBAL_UNCERTAINTY_ASSIGNED_CONTEXT ( ( #137470 ) ) GLOBAL_UNIT_ASSIGNED_CONTEXT ( ( #57085, #2651, #1905 ) ) REPRESENTATION_CONTEXT ( 'NONE', 'WORKASPACE' ) );
#124009=ORIENTED_EDGE ( 'NONE', *, *, #1223, .T. ) ;
#124056=ORIENTED_EDGE ( 'NONE', *, *, #44980, .F. ) ;
#124101=CARTESIAN_POINT ( 'NONE',  ( -55.65468426144000347, -40.29840020119755195, 19.55137198191481218 ) ) ;
#124119=CARTESIAN_POINT ( 'NONE',  ( 12.19999999999999574, -60.26999999999998892, -39.50000000000000000 ) ) ;
#124182=CARTESIAN_POINT ( 'NONE',  ( 34.36534788329977630, 22.27000000000001378, -12.13892467737981740 ) ) ;
#124195=CARTESIAN_POINT ( 'NONE',  ( -7.140000000000000568, -35.07067781378390237, 17.84983973653577749 ) ) ;
#124204=DIRECTION ( 'NONE',  ( 1.000000000000000000, 3.115803279706882722E-16, -0.000000000000000000 ) ) ;
#124237=VERTEX_POINT ( 'NONE', #98703 ) ;
#124243=( NAMED_UNIT ( * ) SI_UNIT ( $, .STERADIAN. ) SOLID_ANGLE_UNIT ( ) );
#124322=EDGE_CURVE ( 'NONE', #92341, #54868, #21151, .T. ) ;
#124348=CARTESIAN_POINT ( 'NONE',  ( -16.73819859380873609, 0.09982356673932113456, -33.96774470396684364 ) ) ;
#124449=CARTESIAN_POINT ( 'NONE',  ( 19.82791644288525390, -2.376042199413920475, -33.22268429432537573 ) ) ;
#124501=LINE ( 'NONE', #12161, #121974 ) ;
#124576=DIRECTION ( 'NONE',  ( -0.000000000000000000, -1.000000000000000000, -0.000000000000000000 ) ) ;
#124578=DIRECTION ( 'NONE',  ( -0.000000000000000000, 0.000000000000000000, 1.000000000000000000 ) ) ;
#124647=ORIENTED_EDGE ( 'NONE', *, *, #3341, .F. ) ;
#124684=VECTOR ( 'NONE', #62588, 1000.000000000000000 ) ;
#124745=( NAMED_UNIT ( * ) PLANE_ANGLE_UNIT ( ) SI_UNIT ( $, .RADIAN. ) );
#124760=DIRECTION ( 'NONE',  ( -1.000000000000000000, -0.000000000000000000, -0.000000000000000000 ) ) ;
#124770=ORIENTED_EDGE ( 'NONE', *, *, #8257, .F. ) ;
#124787=CYLINDRICAL_SURFACE ( 'NONE', #48917, 2.552699999999994418 ) ;
#124801=CARTESIAN_POINT ( 'NONE',  ( -4.199658430161101741, 13.35074831326553024, -24.67186739689545050 ) ) ;
#124809=CARTESIAN_POINT ( 'NONE',  ( 12.69999999999999574, -35.13237070076361590, 17.62370837922860645 ) ) ;
#124865=VECTOR ( 'NONE', #113845, 1000.000000000000000 ) ;
#125126=CARTESIAN_POINT ( 'NONE',  ( 12.49289321881344605, -22.06289321881344634, -40.00000000000000000 ) ) ;
#125132=CIRCLE ( 'NONE', #134476, 0.5000000000000004441 ) ;
#125137=DIRECTION ( 'NONE',  ( -1.000000000000000000, 0.000000000000000000, 0.000000000000000000 ) ) ;
#125167=PRESENTATION_STYLE_ASSIGNMENT (( #67982 ) ) ;
#125193=CIRCLE ( 'NONE', #64988, 0.5000000000000004441 ) ;
#125215=DIRECTION ( 'NONE',  ( 0.000000000000000000, 0.000000000000000000, 1.000000000000000000 ) ) ;
#125223=ORIENTED_EDGE ( 'NONE', *, *, #100410, .T. ) ;
#125244=ADVANCED_FACE ( 'NONE', ( #81655 ), #137444, .F. ) ;
#125305=MECHANICAL_DESIGN_GEOMETRIC_PRESENTATION_REPRESENTATION('',(#72049),#95173);
#125339=ADVANCED_FACE ( 'NONE', ( #83801 ), #126817, .F. ) ;
#125406=AXIS2_PLACEMENT_3D ( 'NONE', #98862, #22705, #77849 ) ;
#125418=VECTOR ( 'NONE', #124760, 1000.000000000000000 ) ;
#125424=ORIENTED_EDGE ( 'NONE', *, *, #109914, .T. ) ;
#125430=SURFACE_STYLE_FILL_AREA ( #136285 ) ;
#125502=CARTESIAN_POINT ( 'NONE',  ( 12.19999999999999574, -40.43000000000000682, 19.06900128115122683 ) ) ;
#125503=VERTEX_POINT ( 'NONE', #96737 ) ;
#125507=SURFACE_STYLE_FILL_AREA ( #60265 ) ;
#125525=EDGE_LOOP ( 'NONE', ( #120783, #126312, #77631, #133297, #71906, #9949 ) ) ;
#125564=CARTESIAN_POINT ( 'NONE',  ( 12.19999999999999574, -59.76999999999998892, -39.50000000000000000 ) ) ;
#125580=ADVANCED_FACE ( 'NONE', ( #11155 ), #46746, .F. ) ;
#125634=FILL_AREA_STYLE_COLOUR ( '', #109211 ) ;
#125643=ADVANCED_FACE ( 'NONE', ( #12615 ), #136241, .F. ) ;
#125692=FILL_AREA_STYLE ('',( #41317 ) ) ;
#125770=CARTESIAN_POINT ( 'NONE',  ( 31.92500000000000782, 22.27000000000000313, -14.71147562388301822 ) ) ;
#125778=DIRECTION ( 'NONE',  ( -1.734723475976805517E-15, -1.000000000000000000, 0.000000000000000000 ) ) ;
#125810=VECTOR ( 'NONE', #66874, 1000.000000000000000 ) ;
#125819=LINE ( 'NONE', #6828, #100381 ) ;
#125823=CIRCLE ( 'NONE', #95680, 0.5000000000000004441 ) ;
#125841=AXIS2_PLACEMENT_3D ( 'NONE', #121503, #22184, #110613 ) ;
#125845=SURFACE_STYLE_USAGE ( .BOTH. , #45447 ) ;
#125997=CARTESIAN_POINT ( 'NONE',  ( -7.140000000000001457, -39.92999999999999261, -39.50000000000000000 ) ) ;
#126011=FACE_OUTER_BOUND ( 'NONE', #126509, .T. ) ;
#126022=CARTESIAN_POINT ( 'NONE',  ( 0.000000000000000000, -40.42999999999999261, -40.00000000000000000 ) ) ;
#126035=CARTESIAN_POINT ( 'NONE',  ( 7.939999999999994174, -60.26999999999998892, -10.00000000000000178 ) ) ;
#126095=EDGE_CURVE ( 'NONE', #25013, #237, #33183, .T. ) ;
#126096=ORIENTED_EDGE ( 'NONE', *, *, #116962, .F. ) ;
#126104=VERTEX_POINT ( 'NONE', #44781 ) ;
#126167=ORIENTED_EDGE ( 'NONE', *, *, #31923, .T. ) ;
#126200=CYLINDRICAL_SURFACE ( 'NONE', #25919, 0.5000000000000004441 ) ;
#126239=AXIS2_PLACEMENT_3D ( 'NONE', #75055, #142436, #96044 ) ;
#126312=ORIENTED_EDGE ( 'NONE', *, *, #71326, .T. ) ;
#126315=ORIENTED_EDGE ( 'NONE', *, *, #14087, .T. ) ;
#126333=VECTOR ( 'NONE', #116843, 1000.000000000000000 ) ;
#126343=CYLINDRICAL_SURFACE ( 'NONE', #66402, 0.5000000000000001110 ) ;
#126351=FACE_OUTER_BOUND ( 'NONE', #98844, .T. ) ;
#126355=DIRECTION ( 'NONE',  ( 0.000000000000000000, 0.000000000000000000, 1.000000000000000000 ) ) ;
#126369=CARTESIAN_POINT ( 'NONE',  ( -31.92499999999997584, -3.270000000000012452, -37.00000000000000000 ) ) ;
#126375=PRESENTATION_STYLE_ASSIGNMENT (( #63119 ) ) ;
#126384=DIRECTION ( 'NONE',  ( -0.000000000000000000, 1.000000000000000000, -0.000000000000000000 ) ) ;
#126404=CARTESIAN_POINT ( 'NONE',  ( -6.640000000000001457, -34.51840020119762187, 17.97447928118982929 ) ) ;
#126421=DIRECTION ( 'NONE',  ( 0.000000000000000000, -0.000000000000000000, -1.000000000000000000 ) ) ;
#126435=CONICAL_SURFACE ( 'NONE', #43161, 2.552699999999994418, 1.029744258676651869 ) ;
#126460=CARTESIAN_POINT ( 'NONE',  ( 19.93618820137057668, -0.2700000000508058218, -36.99999999997771738 ) ) ;
#126468=FILL_AREA_STYLE_COLOUR ( '', #118531 ) ;
#126509=EDGE_LOOP ( 'NONE', ( #72651, #61759, #80128, #62549 ) ) ;
#126519=ORIENTED_EDGE ( 'NONE', *, *, #47975, .T. ) ;
#126525=CARTESIAN_POINT ( 'NONE',  ( -9.989884667592379586, 9.469783904273665343, -27.25938507612927708 ) ) ;
#126539=ORIENTED_EDGE ( 'NONE', *, *, #51734, .F. ) ;
#126572=CARTESIAN_POINT ( 'NONE',  ( 17.54957349175731451, -3.269999995228190848, -36.08445893746787903 ) ) ;
#126576=VERTEX_POINT ( 'NONE', #54746 ) ;
#126592=AXIS2_PLACEMENT_3D ( 'NONE', #43080, #128643, #76420 ) ;
#126677=ORIENTED_EDGE ( 'NONE', *, *, #105415, .T. ) ;
#126687=SURFACE_STYLE_FILL_AREA ( #15748 ) ;
#126703=ORIENTED_EDGE ( 'NONE', *, *, #8418, .F. ) ;
#126723=ORIENTED_EDGE ( 'NONE', *, *, #18720, .F. ) ;
#126727=DIRECTION ( 'NONE',  ( 0.000000000000000000, 0.000000000000000000, -1.000000000000000000 ) ) ;
#126817=CONICAL_SURFACE ( 'NONE', #24986, 1.898649999999993065, 1.029744258676648316 ) ;
#126832=VERTEX_POINT ( 'NONE', #136553 ) ;
#126860=SURFACE_STYLE_USAGE ( .BOTH. , #68966 ) ;
#126863=SURFACE_STYLE_FILL_AREA ( #113866 ) ;
#126896=PRESENTATION_STYLE_ASSIGNMENT (( #48658 ) ) ;
#126957=STYLED_ITEM ( 'NONE', ( #32591 ), #107130 ) ;
#126962=CARTESIAN_POINT ( 'NONE',  ( -16.45742106731621845, 0.9613713492673547911, -33.49048331797055766 ) ) ;
#126992=SURFACE_STYLE_USAGE ( .BOTH. , #82811 ) ;
#127006=EDGE_CURVE ( 'NONE', #89438, #131559, #92081, .T. ) ;
#127027=EDGE_LOOP ( 'NONE', ( #59608, #69293, #91532 ) ) ;
#127087=ORIENTED_EDGE ( 'NONE', *, *, #76752, .T. ) ;
#127095=LINE ( 'NONE', #93055, #58816 ) ;
#127102=CARTESIAN_POINT ( 'NONE',  ( 21.59770000000000323, 3.130000000000007887, -22.35000000000000142 ) ) ;
#127113=ADVANCED_FACE ( 'NONE', ( #141169 ), #108514, .T. ) ;
#127124=CIRCLE ( 'NONE', #18335, 3.000000000000002665 ) ;
#127212=DIRECTION ( 'NONE',  ( 1.000000000000000000, 0.000000000000000000, -0.000000000000000000 ) ) ;
#127216=DIRECTION ( 'NONE',  ( 1.000000000000000000, 3.115803279706882722E-16, 0.000000000000000000 ) ) ;
#127239=CARTESIAN_POINT ( 'NONE',  ( -8.338599238176856332, 10.47657132819572645, -28.51096560023557558 ) ) ;
#127244=VECTOR ( 'NONE', #118205, 1000.000000000000000 ) ;
#127248=ORIENTED_EDGE ( 'NONE', *, *, #96276, .T. ) ;
#127255=DIRECTION ( 'NONE',  ( 0.000000000000000000, 0.000000000000000000, -1.000000000000000000 ) ) ;
#127291=EDGE_CURVE ( 'NONE', #109962, #78214, #48591, .T. ) ;
#127317=CARTESIAN_POINT ( 'NONE',  ( -12.20000000000000284, -34.64999999999999147, -39.50000000000000000 ) ) ;
#127328=AXIS2_PLACEMENT_3D ( 'NONE', #73783, #28857, #129573 ) ;
#127554=MECHANICAL_DESIGN_GEOMETRIC_PRESENTATION_REPRESENTATION('',(#109003),#25715);
#127583=EDGE_CURVE ( 'NONE', #82818, #131125, #69416, .T. ) ;
#127614=DIRECTION ( 'NONE',  ( -1.000000000000000000, 0.000000000000000000, 0.000000000000000000 ) ) ;
#127634=CARTESIAN_POINT ( 'NONE',  ( -12.70000000000000462, -22.26999999999999247, -0.5000000000000004441 ) ) ;
#127656=( LENGTH_UNIT ( ) NAMED_UNIT ( * ) SI_UNIT ( .MILLI., .METRE. ) );
#127671=CARTESIAN_POINT ( 'NONE',  ( -17.44530448566515446, 4.797056265612570591, -29.43923607413351462 ) ) ;
#127706=CARTESIAN_POINT ( 'NONE',  ( 12.19999999999999574, -25.83999999999998565, 13.17925390838734323 ) ) ;
#127725=ORIENTED_EDGE ( 'NONE', *, *, #134132, .T. ) ;
#127801=CARTESIAN_POINT ( 'NONE',  ( 0.000000000000000000, -4.870000000000014317, -36.99999999997771738 ) ) ;
#127821=ORIENTED_EDGE ( 'NONE', *, *, #114101, .T. ) ;
#127852=CARTESIAN_POINT ( 'NONE',  ( -12.20000000000000284, -34.64999999999999147, 17.49210858042622263 ) ) ;
#127854=EDGE_CURVE ( 'NONE', #51304, #23998, #62417, .T. ) ;
#127864=CARTESIAN_POINT ( 'NONE',  ( 19.93618820137057668, -3.269999999999996021, -36.39086428165683174 ) ) ;
#127880=AXIS2_PLACEMENT_3D ( 'NONE', #8925, #141658, #53195 ) ;
#127915=DIRECTION ( 'NONE',  ( 0.000000000000000000, 0.000000000000000000, 1.000000000000000000 ) ) ;
#127946=SURFACE_SIDE_STYLE ('',( #83006 ) ) ;
#127952=( LENGTH_UNIT ( ) NAMED_UNIT ( * ) SI_UNIT ( .MILLI., .METRE. ) );
#127996=ORIENTED_EDGE ( 'NONE', *, *, #65791, .F. ) ;
#128005=AXIS2_PLACEMENT_3D ( 'NONE', #65955, #78234, #23082 ) ;
#128010=ORIENTED_EDGE ( 'NONE', *, *, #108303, .T. ) ;
#128025=EDGE_CURVE ( 'NONE', #60140, #133539, #142122, .T. ) ;
#128034=ORIENTED_EDGE ( 'NONE', *, *, #76417, .T. ) ;
#128044=DIRECTION ( 'NONE',  ( 1.369518533665900312E-16, -1.000000000000000000, 0.000000000000000000 ) ) ;
#128107=AXIS2_PLACEMENT_3D ( 'NONE', #89633, #101940, #78776 ) ;
#128111=CARTESIAN_POINT ( 'NONE',  ( 7.139999999999992575, -35.14999999999999858, 17.49210858042621908 ) ) ;
#128134=DIRECTION ( 'NONE',  ( -1.000000000000000000, 0.000000000000000000, 0.000000000000000000 ) ) ;
#128140=CIRCLE ( 'NONE', #93352, 3.000000000000000000 ) ;
#128182=LINE ( 'NONE', #109072, #113458 ) ;
#128188=AXIS2_PLACEMENT_3D ( 'NONE', #52769, #77436, #75975 ) ;
#128219=CIRCLE ( 'NONE', #19438, 3.000000000000001776 ) ;
#128393=ADVANCED_FACE ( 'NONE', ( #70816 ), #102715, .T. ) ;
#128466=FACE_OUTER_BOUND ( 'NONE', #25569, .T. ) ;
#128478=CARTESIAN_POINT ( 'NONE',  ( 34.71789321881347945, -22.26999999999999247, -0.2071067811865477115 ) ) ;
#128533=EDGE_LOOP ( 'NONE', ( #130597, #16328, #105007, #95231 ) ) ;
#128568=DIRECTION ( 'NONE',  ( 0.000000000000000000, 0.000000000000000000, -1.000000000000000000 ) ) ;
#128588=VERTEX_POINT ( 'NONE', #27267 ) ;
#128632=STYLED_ITEM ( 'NONE', ( #96773 ), #133701 ) ;
#128643=DIRECTION ( 'NONE',  ( 0.000000000000000000, 0.000000000000000000, -1.000000000000000000 ) ) ;
#128648=CARTESIAN_POINT ( 'NONE',  ( 0.000000000000000000, 22.27000000000000668, -40.00000000000000000 ) ) ;
#128664=FACE_OUTER_BOUND ( 'NONE', #131488, .T. ) ;
#128682=PRESENTATION_STYLE_ASSIGNMENT (( #125845 ) ) ;
#128699=VECTOR ( 'NONE', #121427, 1000.000000000000000 ) ;
#128702=SPHERICAL_SURFACE ( 'NONE', #107071, 0.5000000000000000000 ) ;
#128716=FILL_AREA_STYLE_COLOUR ( '', #14205 ) ;
#128742=EDGE_LOOP ( 'NONE', ( #89097, #113802, #105257, #80624 ) ) ;
#128769=CARTESIAN_POINT ( 'NONE',  ( -31.92499999999997584, -6.270000000000012008, -37.00000000000000000 ) ) ;
#128814=VERTEX_POINT ( 'NONE', #112692 ) ;
#128832=EDGE_CURVE ( 'NONE', #23962, #85630, #55862, .T. ) ;
#128924=CARTESIAN_POINT ( 'NONE',  ( -7.140000000000001457, -39.92999999999999261, -12.10072711459627293 ) ) ;
#128930=VERTEX_POINT ( 'NONE', #50307 ) ;
#128950=( BOUNDED_CURVE ( )  B_SPLINE_CURVE ( 3, ( #33775, #80842, #133780, #36589 ),
 .UNSPECIFIED., .F., .T. ) 
 B_SPLINE_CURVE_WITH_KNOTS ( ( 4, 4 ),
 ( -7.105427357601001859E-15, 1.570796326794900111 ),
 .UNSPECIFIED. ) 
 CURVE ( )  GEOMETRIC_REPRESENTATION_ITEM ( )  RATIONAL_B_SPLINE_CURVE ( ( 1.000000000000000000, 0.8047378541243626060, 0.8047378541243626060, 1.000000000000000000 ) ) 
 REPRESENTATION_ITEM ( '' )  );
#128972=CARTESIAN_POINT ( 'NONE',  ( -34.92499999999997584, -21.76999999999999247, -37.00000000000000000 ) ) ;
#129020=CARTESIAN_POINT ( 'NONE',  ( -12.19999999999999929, -60.26999999999998892, -40.00000000000000000 ) ) ;
#129025=VERTEX_POINT ( 'NONE', #16955 ) ;
#129034=EDGE_CURVE ( 'NONE', #108517, #143240, #109001, .T. ) ;
#129041=CARTESIAN_POINT ( 'NONE',  ( 0.000000000000000000, -59.76999999999998892, -39.50000000000000000 ) ) ;
#129068=CIRCLE ( 'NONE', #105967, 0.4999999999999996669 ) ;
#129090=SURFACE_STYLE_USAGE ( .BOTH. , #41365 ) ;
#129092=ORIENTED_EDGE ( 'NONE', *, *, #129833, .T. ) ;
#129114=FILL_AREA_STYLE_COLOUR ( '', #79480 ) ;
#129131=B_SPLINE_CURVE_WITH_KNOTS ( 'NONE', 3,
 ( #22001, #100303, #98159, #66960 ),
 .UNSPECIFIED., .F., .F.,
 ( 4, 4 ),
 ( 0.001201692628197130247, 0.001634763834693580111 ),
 .UNSPECIFIED. ) ;
#129136=PRESENTATION_STYLE_ASSIGNMENT (( #140041 ) ) ;
#129181=ADVANCED_FACE ( 'NONE', ( #120503 ), #132343, .T. ) ;
#129191=CARTESIAN_POINT ( 'NONE',  ( 7.940000000000001279, -35.14999999999999858, -10.00000000000000178 ) ) ;
#129249=CIRCLE ( 'NONE', #66772, 31.92999999999999261 ) ;
#129305=CIRCLE ( 'NONE', #15851, 2.247899999999995568 ) ;
#129328=VERTEX_POINT ( 'NONE', #96972 ) ;
#129367=CARTESIAN_POINT ( 'NONE',  ( -16.50229999999999819, 3.130000000000007887, -22.35000000000000142 ) ) ;
#129368=ADVANCED_FACE ( 'NONE', ( #117318 ), #41199, .T. ) ;
#129379=CARTESIAN_POINT ( 'NONE',  ( 7.515903222916713311, 10.89581445352136946, -28.18232836037424605 ) ) ;
#129396=ORIENTED_EDGE ( 'NONE', *, *, #14352, .T. ) ;
#129441=ORIENTED_EDGE ( 'NONE', *, *, #57587, .F. ) ;
#129474=ORIENTED_EDGE ( 'NONE', *, *, #20401, .T. ) ;
#129497=CARTESIAN_POINT ( 'NONE',  ( -34.92499999999997584, -21.76999999999999247, -40.00000000000000000 ) ) ;
#129499=COLOUR_RGB ( '', 0.66274510, 0.83137255, 0.94901961) ;
#129520=DIRECTION ( 'NONE',  ( 1.000000000000000000, 0.000000000000000000, 0.000000000000000000 ) ) ;
#129528=FACE_OUTER_BOUND ( 'NONE', #127027, .T. ) ;
#129535=AXIS2_PLACEMENT_3D ( 'NONE', #69754, #3698, #327 ) ;
#129545=ORIENTED_EDGE ( 'NONE', *, *, #106837, .F. ) ;
#129573=DIRECTION ( 'NONE',  ( 0.000000000000000000, 0.000000000000000000, 1.000000000000000000 ) ) ;
#129579=CARTESIAN_POINT ( 'NONE',  ( 31.92500000000001492, -6.269999999999992468, -37.00000000000000000 ) ) ;
#129593=CYLINDRICAL_SURFACE ( 'NONE', #90722, 2.247899999999996901 ) ;
#129597=DIRECTION ( 'NONE',  ( 0.000000000000000000, 0.000000000000000000, -1.000000000000000000 ) ) ;
#129612=SURFACE_STYLE_USAGE ( .BOTH. , #63685 ) ;
#129641=CIRCLE ( 'NONE', #99516, 6.000000000000001776 ) ;
#129660=MECHANICAL_DESIGN_GEOMETRIC_PRESENTATION_REPRESENTATION('',(#27840),#55593);
#129685=SURFACE_STYLE_USAGE ( .BOTH. , #137012 ) ;
#129698=DIRECTION ( 'NONE',  ( 0.000000000000000000, 1.000000000000000000, 0.000000000000000000 ) ) ;
#129712=FACE_OUTER_BOUND ( 'NONE', #17785, .T. ) ;
#129722=SURFACE_SIDE_STYLE ('',( #120240 ) ) ;
#129813=CIRCLE ( 'NONE', #25591, 2.500000000000002220 ) ;
#129819=VERTEX_POINT ( 'NONE', #33069 ) ;
#129833=EDGE_CURVE ( 'NONE', #96844, #126104, #11228, .T. ) ;
#129855=MECHANICAL_DESIGN_GEOMETRIC_PRESENTATION_REPRESENTATION('',(#113699),#51220);
#129909=CARTESIAN_POINT ( 'NONE',  ( -6.640000000000001457, -34.64999999999999147, -40.00000000000000000 ) ) ;
#129971=CARTESIAN_POINT ( 'NONE',  ( 7.939999999999994174, -60.26999999999998892, -7.752100000000003099 ) ) ;
#129981=CARTESIAN_POINT ( 'NONE',  ( 0.000000000000000000, -39.92999999999999261, -39.50000000000000000 ) ) ;
#129999=DIRECTION ( 'NONE',  ( -0.000000000000000000, -0.000000000000000000, 1.000000000000000000 ) ) ;
#130019=CARTESIAN_POINT ( 'NONE',  ( 7.139999999999991687, -35.76999999999998892, -12.10072711459627293 ) ) ;
#130052=( GEOMETRIC_REPRESENTATION_CONTEXT ( 3 ) GLOBAL_UNCERTAINTY_ASSIGNED_CONTEXT ( ( #82381 ) ) GLOBAL_UNIT_ASSIGNED_CONTEXT ( ( #24133, #35031, #90083 ) ) REPRESENTATION_CONTEXT ( 'NONE', 'WORKASPACE' ) );
#130056=( NAMED_UNIT ( * ) PLANE_ANGLE_UNIT ( ) SI_UNIT ( $, .RADIAN. ) );
#130078=DIRECTION ( 'NONE',  ( -0.000000000000000000, 0.000000000000000000, 1.000000000000000000 ) ) ;
#130115=EDGE_CURVE ( 'NONE', #58061, #66948, #56950, .T. ) ;
#130122=CARTESIAN_POINT ( 'NONE',  ( 7.354306473674146361, 12.49300487098931001, -25.30134302938294155 ) ) ;
#130154=ORIENTED_EDGE ( 'NONE', *, *, #60631, .F. ) ;
#130165=ORIENTED_EDGE ( 'NONE', *, *, #118347, .F. ) ;
#130177=DIRECTION ( 'NONE',  ( -0.000000000000000000, -1.000000000000000000, -0.000000000000000000 ) ) ;
#130196=UNCERTAINTY_MEASURE_WITH_UNIT (LENGTH_MEASURE( 1.000000000000000082E-05 ), #96070, 'distance_accuracy_value', 'NONE');
#130197=AXIS2_PLACEMENT_3D ( 'NONE', #115244, #49363, #37015 ) ;
#130249=( GEOMETRIC_REPRESENTATION_CONTEXT ( 3 ) GLOBAL_UNCERTAINTY_ASSIGNED_CONTEXT ( ( #137840 ) ) GLOBAL_UNIT_ASSIGNED_CONTEXT ( ( #139915, #131154, #31147 ) ) REPRESENTATION_CONTEXT ( 'NONE', 'WORKASPACE' ) );
#130282=VECTOR ( 'NONE', #107808, 1000.000000000000114 ) ;
#130286=COLOUR_RGB ( '', 0.31764706, 0.68627451, 0.89019608) ;
#130301=CARTESIAN_POINT ( 'NONE',  ( 31.92500000000001492, -6.269999999999992468, -40.00000000000000000 ) ) ;
#130343=SURFACE_STYLE_FILL_AREA ( #106386 ) ;
#130357=CARTESIAN_POINT ( 'NONE',  ( 34.92500000000001847, 1.088194295437629318E-14, -40.00000000000000000 ) ) ;
#130361=UNCERTAINTY_MEASURE_WITH_UNIT (LENGTH_MEASURE( 1.000000000000000082E-05 ), #90232, 'distance_accuracy_value', 'NONE');
#130384=( LENGTH_UNIT ( ) NAMED_UNIT ( * ) SI_UNIT ( .MILLI., .METRE. ) );
#130398=DIRECTION ( 'NONE',  ( -0.000000000000000000, 2.242629915582283412E-16, -1.000000000000000000 ) ) ;
#130538=CYLINDRICAL_SURFACE ( 'NONE', #41554, 3.000000000000002665 ) ;
#130561=EDGE_CURVE ( 'NONE', #73050, #112438, #86263, .T. ) ;
#130563=DIRECTION ( 'NONE',  ( -0.9743982503113671756, -0.2248289345038712306, 0.000000000000000000 ) ) ;
#130569=CARTESIAN_POINT ( 'NONE',  ( 12.83744844559187293, 6.995917548256143981, -30.85333074290490529 ) ) ;
#130597=ORIENTED_EDGE ( 'NONE', *, *, #72661, .T. ) ;
#130712=CARTESIAN_POINT ( 'NONE',  ( 31.92500000000001492, -6.269999999999992468, -37.00000000000000000 ) ) ;
#130764=CIRCLE ( 'NONE', #35878, 3.000000000000002665 ) ;
#130834=DIRECTION ( 'NONE',  ( -1.000000000000000000, 0.000000000000000000, 0.000000000000000000 ) ) ;
#130853=CARTESIAN_POINT ( 'NONE',  ( 8.331076807256511785, 12.11968929156625308, -25.56276712144670427 ) ) ;
#130857=FILL_AREA_STYLE_COLOUR ( '', #28004 ) ;
#130966=LINE ( 'NONE', #129497, #103440 ) ;
#130983=ORIENTED_EDGE ( 'NONE', *, *, #73754, .F. ) ;
#130989=FACE_OUTER_BOUND ( 'NONE', #118995, .T. ) ;
#130996=DIRECTION ( 'NONE',  ( -0.000000000000000000, -0.000000000000000000, -1.000000000000000000 ) ) ;
#131003=EDGE_LOOP ( 'NONE', ( #48139, #105825, #140, #126723 ) ) ;
#131041=DIRECTION ( 'NONE',  ( -0.000000000000000000, -1.000000000000000000, -0.000000000000000000 ) ) ;
#131052=DIRECTION ( 'NONE',  ( -0.000000000000000000, -1.000000000000000000, -0.000000000000000000 ) ) ;
#131125=VERTEX_POINT ( 'NONE', #41490 ) ;
#131133=CARTESIAN_POINT ( 'NONE',  ( 7.139999999999992575, -35.14999999999999858, -39.50000000000000000 ) ) ;
#131135=EDGE_CURVE ( 'NONE', #22146, #1800, #74136, .T. ) ;
#131154=( NAMED_UNIT ( * ) PLANE_ANGLE_UNIT ( ) SI_UNIT ( $, .RADIAN. ) );
#131162=PLANE ( 'NONE',  #143319 ) ;
#131163=CARTESIAN_POINT ( 'NONE',  ( 19.28515664589288292, 1.963325189347669086, -33.49048331797055766 ) ) ;
#131177=CARTESIAN_POINT ( 'NONE',  ( -7.940000000000001279, -60.26999999999998892, -8.101350000000007157 ) ) ;
#131218=DIRECTION ( 'NONE',  ( 1.000000000000000000, 1.369518533665899572E-16, 0.000000000000000000 ) ) ;
#131250=VERTEX_POINT ( 'NONE', #66131 ) ;
#131271=AXIS2_PLACEMENT_3D ( 'NONE', #78396, #132078, #122593 ) ;
#131285=SURFACE_STYLE_USAGE ( .BOTH. , #87069 ) ;
#131359=VERTEX_POINT ( 'NONE', #11687 ) ;
#131384=ORIENTED_EDGE ( 'NONE', *, *, #98051, .T. ) ;
#131435=CARTESIAN_POINT ( 'NONE',  ( 12.69999999999999574, -25.83999999999998565, 2.999999999999999112 ) ) ;
#131452=( BOUNDED_CURVE ( )  B_SPLINE_CURVE ( 3, ( #103720, #82041, #116763, #137827 ),
 .UNSPECIFIED., .F., .T. ) 
 B_SPLINE_CURVE_WITH_KNOTS ( ( 4, 4 ),
 ( 1.570796326794896558, 3.141592653589793116 ),
 .UNSPECIFIED. ) 
 CURVE ( )  GEOMETRIC_REPRESENTATION_ITEM ( )  RATIONAL_B_SPLINE_CURVE ( ( 1.000000000000000000, 0.8047378541243649375, 0.8047378541243649375, 1.000000000000000000 ) ) 
 REPRESENTATION_ITEM ( '' )  );
#131474=LINE ( 'NONE', #113089, #15135 ) ;
#131482=CARTESIAN_POINT ( 'NONE',  ( 0.000000000000000000, -22.26999999999999247, -40.00000000000000000 ) ) ;
#131488=EDGE_LOOP ( 'NONE', ( #30811, #26119, #47984, #75646 ) ) ;
#131500=MECHANICAL_DESIGN_GEOMETRIC_PRESENTATION_REPRESENTATION('',(#103629),#138433);
#131531=MECHANICAL_DESIGN_GEOMETRIC_PRESENTATION_REPRESENTATION('',(#8833),#108401);
#131539=ADVANCED_FACE ( 'NONE', ( #7960 ), #126200, .T. ) ;
#131541=CARTESIAN_POINT ( 'NONE',  ( 7.109511292951834704, 11.08337169632131669, -28.03137008052015133 ) ) ;
#131559=VERTEX_POINT ( 'NONE', #127634 ) ;
#131601=( NAMED_UNIT ( * ) PLANE_ANGLE_UNIT ( ) SI_UNIT ( $, .RADIAN. ) );
#131604=COLOUR_RGB ( '', 0.08235294, 0.09019608, 0.10196078) ;
#131616=UNCERTAINTY_MEASURE_WITH_UNIT (LENGTH_MEASURE( 1.000000000000000082E-05 ), #85109, 'distance_accuracy_value', 'NONE');
#131662=SURFACE_STYLE_USAGE ( .BOTH. , #109179 ) ;
#131674=ORIENTED_EDGE ( 'NONE', *, *, #44004, .F. ) ;
#131675=ADVANCED_FACE ( 'NONE', ( #8646 ), #42065, .F. ) ;
#131687=ORIENTED_EDGE ( 'NONE', *, *, #36918, .F. ) ;
#131738=MECHANICAL_DESIGN_GEOMETRIC_PRESENTATION_REPRESENTATION('',(#97015),#6669);
#131801=CARTESIAN_POINT ( 'NONE',  ( 0.000000000000000000, -22.26999999999999247, -0.5000000000000004441 ) ) ;
#131817=FACE_OUTER_BOUND ( 'NONE', #128533, .T. ) ;
#131890=FACE_OUTER_BOUND ( 'NONE', #119772, .T. ) ;
#131896=FILL_AREA_STYLE ('',( #111557 ) ) ;
#131944=FACE_OUTER_BOUND ( 'NONE', #26710, .T. ) ;
#131993=CARTESIAN_POINT ( 'NONE',  ( 9.512856086559503765, 9.797339893906631403, -29.02678346616960425 ) ) ;
#132003=ORIENTED_EDGE ( 'NONE', *, *, #64691, .F. ) ;
#132011=( NAMED_UNIT ( * ) SI_UNIT ( $, .STERADIAN. ) SOLID_ANGLE_UNIT ( ) );
#132078=DIRECTION ( 'NONE',  ( 1.000000000000000000, -0.000000000000000000, -0.000000000000000000 ) ) ;
#132086=ORIENTED_EDGE ( 'NONE', *, *, #94870, .F. ) ;
#132092=SURFACE_SIDE_STYLE ('',( #121880 ) ) ;
#132124=MECHANICAL_DESIGN_GEOMETRIC_PRESENTATION_REPRESENTATION('',(#65069),#106611);
#132172=CYLINDRICAL_SURFACE ( 'NONE', #36579, 0.5000000000000004441 ) ;
#132181=CARTESIAN_POINT ( 'NONE',  ( -12.70000000000000995, 12.19802518668052294, 4.711086268963008195 ) ) ;
#132223=AXIS2_PLACEMENT_3D ( 'NONE', #16531, #49920, #4913 ) ;
#132276=DIRECTION ( 'NONE',  ( -1.000000000000000000, 0.000000000000000000, 0.000000000000000000 ) ) ;
#132287=CARTESIAN_POINT ( 'NONE',  ( 17.75907150484199448, 4.272537658411479811, -29.62615593856758167 ) ) ;
#132295=VERTEX_POINT ( 'NONE', #95900 ) ;
#132309=( NAMED_UNIT ( * ) PLANE_ANGLE_UNIT ( ) SI_UNIT ( $, .RADIAN. ) );
#132343=TOROIDAL_SURFACE ( 'NONE', #49020, 2.500000000000000000, 0.5000000000000000000 ) ;
#132347=SURFACE_STYLE_USAGE ( .BOTH. , #9804 ) ;
#132358=PRESENTATION_STYLE_ASSIGNMENT (( #121431 ) ) ;
#132408=( NAMED_UNIT ( * ) PLANE_ANGLE_UNIT ( ) SI_UNIT ( $, .RADIAN. ) );
#132411=VECTOR ( 'NONE', #111047, 1000.000000000000000 ) ;
#132461=ORIENTED_EDGE ( 'NONE', *, *, #105393, .T. ) ;
#132463=EDGE_LOOP ( 'NONE', ( #88986, #58682, #51873, #53210 ) ) ;
#132496=DIRECTION ( 'NONE',  ( 0.000000000000000000, -1.000000000000000000, 0.000000000000000000 ) ) ;
#132504=CARTESIAN_POINT ( 'NONE',  ( -31.92499999999997584, 22.26999999999998181, -14.71147562388301822 ) ) ;
#132525=ORIENTED_EDGE ( 'NONE', *, *, #121789, .F. ) ;
#132557=DIRECTION ( 'NONE',  ( 3.973028287378889149E-16, -1.000000000000000000, 0.000000000000000000 ) ) ;
#132580=MECHANICAL_DESIGN_GEOMETRIC_PRESENTATION_REPRESENTATION('',(#51527),#63131);
#132610=DIRECTION ( 'NONE',  ( 1.000000000000000000, 0.000000000000000000, 0.000000000000000000 ) ) ;
#132637=CARTESIAN_POINT ( 'NONE',  ( -12.20000000000000284, -39.92999999999999261, -40.00000000000000000 ) ) ;
#132642=DIRECTION ( 'NONE',  ( 0.000000000000000000, 0.000000000000000000, -1.000000000000000000 ) ) ;
#132646=ORIENTED_EDGE ( 'NONE', *, *, #40430, .F. ) ;
#132664=CIRCLE ( 'NONE', #19205, 0.5000000000000004441 ) ;
#132677=CARTESIAN_POINT ( 'NONE',  ( 16.45742106731621135, 0.9613713492673626737, -33.49048331797055766 ) ) ;
#132706=AXIS2_PLACEMENT_3D ( 'NONE', #123689, #55565, #78035 ) ;
#132725=ORIENTED_EDGE ( 'NONE', *, *, #117639, .T. ) ;
#132731=CARTESIAN_POINT ( 'NONE',  ( 16.15220243791050336, 1.822765899684732238, -33.22366253240541312 ) ) ;
#132796=ORIENTED_EDGE ( 'NONE', *, *, #80182, .T. ) ;
#132806=ORIENTED_EDGE ( 'NONE', *, *, #86213, .T. ) ;
#132807=DIRECTION ( 'NONE',  ( 1.000000000000000000, 0.000000000000000000, 0.000000000000000000 ) ) ;
#132812=DIRECTION ( 'NONE',  ( 1.000000000000000000, 0.000000000000000000, 0.000000000000000000 ) ) ;
#132846=PRODUCT_DEFINITION_FORMATION_WITH_SPECIFIED_SOURCE ( 'ANY', '', #7609, .NOT_KNOWN. ) ;
#132859=CARTESIAN_POINT ( 'NONE',  ( -12.70000000000000817, -1.739288537755694446E-15, -40.00000000000000000 ) ) ;
#132868=FILL_AREA_STYLE_COLOUR ( '', #45994 ) ;
#132883=VERTEX_POINT ( 'NONE', #61020 ) ;
#132888=CIRCLE ( 'NONE', #49589, 0.5000000000000000000 ) ;
#132896=CIRCLE ( 'NONE', #84264, 14.46000000000000085 ) ;
#132926=FACE_OUTER_BOUND ( 'NONE', #125525, .T. ) ;
#132947=CYLINDRICAL_SURFACE ( 'NONE', #81678, 0.5000000000000004441 ) ;
#132975=EDGE_LOOP ( 'NONE', ( #137087, #16548, #48775, #120041 ) ) ;
#133084=DIRECTION ( 'NONE',  ( 0.000000000000000000, 1.000000000000000000, 0.000000000000000000 ) ) ;
#133086=ADVANCED_FACE ( 'NONE', ( #36886 ), #26034, .T. ) ;
#133127=CARTESIAN_POINT ( 'NONE',  ( -12.20000000000000462, -21.76999999999999247, 0.000000000000000000 ) ) ;
#133159=DIRECTION ( 'NONE',  ( 0.000000000000000000, 0.000000000000000000, 1.000000000000000000 ) ) ;
#133163=FILL_AREA_STYLE ('',( #36663 ) ) ;
#133185=EDGE_LOOP ( 'NONE', ( #38420, #6106, #13672, #43505 ) ) ;
#133214=CARTESIAN_POINT ( 'NONE',  ( 16.63171309283781696, 0.4494914063655743863, -33.70035307763171062 ) ) ;
#133219=ORIENTED_EDGE ( 'NONE', *, *, #87004, .F. ) ;
#133223=CARTESIAN_POINT ( 'NONE',  ( -8.648657329869978142E-14, -34.64999999999997726, -40.00000000000000000 ) ) ;
#133252=DIRECTION ( 'NONE',  ( -1.000000000000000000, -3.115803279706882722E-16, 0.000000000000000000 ) ) ;
#133260=SURFACE_STYLE_USAGE ( .BOTH. , #88321 ) ;
#133297=ORIENTED_EDGE ( 'NONE', *, *, #137656, .F. ) ;
#133325=CARTESIAN_POINT ( 'NONE',  ( -12.70000000000000817, -1.739288537755694446E-15, -40.00000000000000000 ) ) ;
#133372=EDGE_CURVE ( 'NONE', #125503, #19482, #21578, .T. ) ;
#133388=UNCERTAINTY_MEASURE_WITH_UNIT (LENGTH_MEASURE( 1.000000000000000082E-05 ), #5955, 'distance_accuracy_value', 'NONE');
#133415=DIRECTION ( 'NONE',  ( 1.400468248933914810E-15, 0.9647414015272155474, -0.2631995976047525887 ) ) ;
#133441=ADVANCED_FACE ( 'NONE', ( #46949 ), #41970, .F. ) ;
#133453=CARTESIAN_POINT ( 'NONE',  ( -9.524999999999991473, -4.870000000000014317, -10.00000000000000178 ) ) ;
#133469=LINE ( 'NONE', #21121, #85974 ) ;
#133510=DIRECTION ( 'NONE',  ( -0.000000000000000000, -0.000000000000000000, 1.000000000000000000 ) ) ;
#133539=VERTEX_POINT ( 'NONE', #28731 ) ;
#133542=ADVANCED_FACE ( 'NONE', ( #72973 ), #95388, .T. ) ;
#133563=EDGE_CURVE ( 'NONE', #56577, #63324, #38394, .T. ) ;
#133631=DIRECTION ( 'NONE',  ( 0.000000000000000000, -1.000000000000000000, 0.000000000000000000 ) ) ;
#133658=ORIENTED_EDGE ( 'NONE', *, *, #88831, .F. ) ;
#133687=STYLED_ITEM ( 'NONE', ( #15870 ), #110241 ) ;
#133689=CARTESIAN_POINT ( 'NONE',  ( 17.49525436401519229, 4.684374302865251138, -29.47233687491770482 ) ) ;
#133701=ADVANCED_FACE ( 'NONE', ( #21413 ), #126435, .F. ) ;
#133747=DIRECTION ( 'NONE',  ( 0.000000000000000000, 0.000000000000000000, 1.000000000000000000 ) ) ;
#133753=PLANE ( 'NONE',  #120910 ) ;
#133778=CIRCLE ( 'NONE', #119866, 0.5000000000000004441 ) ;
#133780=CARTESIAN_POINT ( 'NONE',  ( -12.70000000000000107, -60.06289321881342858, 24.72882142070204736 ) ) ;
#133817=ADVANCED_FACE ( 'NONE', ( #84205 ), #89405, .T. ) ;
#133825=( LENGTH_UNIT ( ) NAMED_UNIT ( * ) SI_UNIT ( .MILLI., .METRE. ) );
#133834=DIRECTION ( 'NONE',  ( 2.496005001405472275E-15, 1.000000000000000000, 0.000000000000000000 ) ) ;
#133838=EDGE_CURVE ( 'NONE', #103756, #43110, #71898, .T. ) ;
#133872=MECHANICAL_DESIGN_GEOMETRIC_PRESENTATION_REPRESENTATION('',(#45931),#138534);
#133880=AXIS2_PLACEMENT_3D ( 'NONE', #17225, #116540, #28827 ) ;
#133904=CARTESIAN_POINT ( 'NONE',  ( 19.86756573869621434, -2.692863782213888335, -33.80212331857929797 ) ) ;
#133908=CARTESIAN_POINT ( 'NONE',  ( -19.93618820137057668, -3.270000000000008455, -36.99999999997771738 ) ) ;
#133960=DIRECTION ( 'NONE',  ( -0.000000000000000000, -1.000000000000000000, -0.000000000000000000 ) ) ;
#134000=EDGE_CURVE ( 'NONE', #58156, #57981, #43741, .T. ) ;
#134002=CIRCLE ( 'NONE', #96905, 0.5000000000000004441 ) ;
#134010=AXIS2_PLACEMENT_3D ( 'NONE', #30550, #29807, #42868 ) ;
#134015=DIRECTION ( 'NONE',  ( 0.000000000000000000, -1.000000000000000000, 0.000000000000000000 ) ) ;
#134072=CARTESIAN_POINT ( 'NONE',  ( 6.639999999999984581, -40.42999999999999972, -40.00000000000000000 ) ) ;
#134096=STYLED_ITEM ( 'NONE', ( #140663 ), #139343 ) ;
#134108=CARTESIAN_POINT ( 'NONE',  ( 7.939999999999994174, -32.12917598568331101, -10.00000000000000178 ) ) ;
#134121=ORIENTED_EDGE ( 'NONE', *, *, #54703, .F. ) ;
#134127=DIRECTION ( 'NONE',  ( -0.000000000000000000, 0.000000000000000000, 1.000000000000000000 ) ) ;
#134128=CARTESIAN_POINT ( 'NONE',  ( 7.139999999999991687, -35.69931899287964683, -11.97485302731577939 ) ) ;
#134132=EDGE_CURVE ( 'NONE', #91102, #140981, #119484, .T. ) ;
#134151=DIRECTION ( 'NONE',  ( 0.000000000000000000, -0.000000000000000000, -1.000000000000000000 ) ) ;
#134240=DIRECTION ( 'NONE',  ( 0.000000000000000000, -1.000000000000000000, 0.000000000000000000 ) ) ;
#134249=ORIENTED_EDGE ( 'NONE', *, *, #73941, .T. ) ;
#134277=EDGE_LOOP ( 'NONE', ( #134527, #48657, #49922, #102358 ) ) ;
#134280=AXIS2_PLACEMENT_3D ( 'NONE', #70096, #112135, #1187 ) ;
#134284=ORIENTED_EDGE ( 'NONE', *, *, #130561, .T. ) ;
#134288=AXIS2_PLACEMENT_3D ( 'NONE', #49383, #103016, #3652 ) ;
#134295=STYLED_ITEM ( 'NONE', ( #139408 ), #114719 ) ;
#134318=VERTEX_POINT ( 'NONE', #128924 ) ;
#134379=ORIENTED_EDGE ( 'NONE', *, *, #7843, .T. ) ;
#134388=CARTESIAN_POINT ( 'NONE',  ( 7.122370700763592133, -39.92999999999999972, 19.06900128115122328 ) ) ;
#134413=CARTESIAN_POINT ( 'NONE',  ( -19.93618820137057668, -0.2700000000508183118, -36.99999999997771738 ) ) ;
#134475=UNCERTAINTY_MEASURE_WITH_UNIT (LENGTH_MEASURE( 1.000000000000000082E-05 ), #45802, 'distance_accuracy_value', 'NONE');
#134476=AXIS2_PLACEMENT_3D ( 'NONE', #127706, #116086, #3723 ) ;
#134527=ORIENTED_EDGE ( 'NONE', *, *, #22113, .F. ) ;
#134530=CARTESIAN_POINT ( 'NONE',  ( -17.29187175597492399, -1.888566033147011769, -32.52167028562607243 ) ) ;
#134535=FILL_AREA_STYLE ('',( #25744 ) ) ;
#134536=AXIS2_PLACEMENT_3D ( 'NONE', #130301, #118682, #83212 ) ;
#134620=CARTESIAN_POINT ( 'NONE',  ( -32.75085989791905661, 22.27000000000000313, -14.49214836789566263 ) ) ;
#134627=UNCERTAINTY_MEASURE_WITH_UNIT (LENGTH_MEASURE( 1.000000000000000082E-05 ), #53307, 'distance_accuracy_value', 'NONE');
#134735=DIRECTION ( 'NONE',  ( -1.000000000000000000, -0.000000000000000000, -0.000000000000000000 ) ) ;
#134740=ORIENTED_EDGE ( 'NONE', *, *, #94940, .F. ) ;
#134778=SURFACE_STYLE_FILL_AREA ( #131896 ) ;
#134798=ORIENTED_EDGE ( 'NONE', *, *, #23055, .T. ) ;
#134814=DIRECTION ( 'NONE',  ( -1.000000000000000000, 1.451651444332056451E-15, 0.000000000000000000 ) ) ;
#134819=STYLED_ITEM ( 'NONE', ( #96315 ), #11968 ) ;
#134830=ORIENTED_EDGE ( 'NONE', *, *, #56951, .F. ) ;
#134831=UNCERTAINTY_MEASURE_WITH_UNIT (LENGTH_MEASURE( 1.000000000000000082E-05 ), #21217, 'distance_accuracy_value', 'NONE');
#134835=DIRECTION ( 'NONE',  ( 1.000000000000000000, 0.000000000000000000, 0.000000000000000000 ) ) ;
#134883=ADVANCED_FACE ( 'NONE', ( #111098 ), #98808, .T. ) ;
#135023=ORIENTED_EDGE ( 'NONE', *, *, #105365, .F. ) ;
#135049=AXIS2_PLACEMENT_3D ( 'NONE', #122658, #21215, #865 ) ;
#135058=CARTESIAN_POINT ( 'NONE',  ( -19.93618820135885272, -3.270000000000008455, -36.39086428169088094 ) ) ;
#135067=CARTESIAN_POINT ( 'NONE',  ( 12.19999999999999574, -27.55040120718573604, 16.07347811296899209 ) ) ;
#135087=EDGE_CURVE ( 'NONE', #2401, #106633, #87334, .T. ) ;
#135088=DIRECTION ( 'NONE',  ( 1.000000000000000000, 0.000000000000000000, 0.000000000000000000 ) ) ;
#135098=CARTESIAN_POINT ( 'NONE',  ( -31.92499999999997584, -6.270000000000012896, -40.00000000000000000 ) ) ;
#135106=VECTOR ( 'NONE', #36595, 1000.000000000000000 ) ;
#135111=CARTESIAN_POINT ( 'NONE',  ( -6.771599798802371950, -34.64999999999999147, 17.99210858042621908 ) ) ;
#135127=ORIENTED_EDGE ( 'NONE', *, *, #37672, .T. ) ;
#135143=CARTESIAN_POINT ( 'NONE',  ( 16.42522110613515451, 1.155309361455200357, -30.62612907365273429 ) ) ;
#135243=AXIS2_PLACEMENT_3D ( 'NONE', #10679, #31061, #120146 ) ;
#135253=CARTESIAN_POINT ( 'NONE',  ( -17.00227007675744417, -0.8971235601602828291, -35.72539454602287634 ) ) ;
#135254=EDGE_LOOP ( 'NONE', ( #98120, #96346, #72493, #86598 ) ) ;
#135259=ORIENTED_EDGE ( 'NONE', *, *, #13442, .F. ) ;
#135315=LINE ( 'NONE', #101219, #58367 ) ;
#135353=VECTOR ( 'NONE', #37142, 1000.000000000000114 ) ;
#135357=FILL_AREA_STYLE_COLOUR ( '', #87027 ) ;
#135390=ORIENTED_EDGE ( 'NONE', *, *, #43017, .T. ) ;
#135410=CYLINDRICAL_SURFACE ( 'NONE', #53929, 2.247899999999996901 ) ;
#135430=VERTEX_POINT ( 'NONE', #93311 ) ;
#135581=MECHANICAL_DESIGN_GEOMETRIC_PRESENTATION_REPRESENTATION('',(#128632),#29076);
#135652=VERTEX_POINT ( 'NONE', #88158 ) ;
#135656=STYLED_ITEM ( 'NONE', ( #71951 ), #108794 ) ;
#135806=SURFACE_STYLE_FILL_AREA ( #57553 ) ;
#135866=EDGE_CURVE ( 'NONE', #103352, #104775, #101068, .T. ) ;
#135952=COLOUR_RGB ( '', 0.31764706, 0.68627451, 0.89019608) ;
#135967=SURFACE_SIDE_STYLE ('',( #58472 ) ) ;
#136023=DIRECTION ( 'NONE',  ( -0.000000000000000000, -1.000000000000000000, -0.000000000000000000 ) ) ;
#136036=CARTESIAN_POINT ( 'NONE',  ( 16.84501342860041717, -0.1639118413482353043, -31.04646532293632788 ) ) ;
#136082=( NAMED_UNIT ( * ) SI_UNIT ( $, .STERADIAN. ) SOLID_ANGLE_UNIT ( ) );
#136099=ORIENTED_EDGE ( 'NONE', *, *, #6127, .T. ) ;
#136121=( GEOMETRIC_REPRESENTATION_CONTEXT ( 3 ) GLOBAL_UNCERTAINTY_ASSIGNED_CONTEXT ( ( #76536 ) ) GLOBAL_UNIT_ASSIGNED_CONTEXT ( ( #56860, #113313, #111921 ) ) REPRESENTATION_CONTEXT ( 'NONE', 'WORKASPACE' ) );
#136161=DIRECTION ( 'NONE',  ( 1.000000000000000000, 0.000000000000000000, 0.000000000000000000 ) ) ;
#136241=CONICAL_SURFACE ( 'NONE', #15730, 2.552699999999994418, 1.029744258676651869 ) ;
#136243=CARTESIAN_POINT ( 'NONE',  ( 6.639999999999992575, -35.15000000000000568, 18.14679158439240325 ) ) ;
#136244=AXIS2_PLACEMENT_3D ( 'NONE', #71259, #60391, #104579 ) ;
#136267=EDGE_LOOP ( 'NONE', ( #101154, #67962 ) ) ;
#136285=FILL_AREA_STYLE ('',( #3602 ) ) ;
#136290=EDGE_CURVE ( 'NONE', #109867, #67375, #40864, .T. ) ;
#136308=EDGE_LOOP ( 'NONE', ( #48727, #82124, #49372, #64511 ) ) ;
#136326=ADVANCED_FACE ( 'NONE', ( #6617 ), #116860, .T. ) ;
#136327=FACE_OUTER_BOUND ( 'NONE', #43416, .T. ) ;
#136328=FACE_OUTER_BOUND ( 'NONE', #17507, .T. ) ;
#136336=ORIENTED_EDGE ( 'NONE', *, *, #133563, .F. ) ;
#136349=( GEOMETRIC_REPRESENTATION_CONTEXT ( 3 ) GLOBAL_UNCERTAINTY_ASSIGNED_CONTEXT ( ( #89664 ) ) GLOBAL_UNIT_ASSIGNED_CONTEXT ( ( #57436, #35703, #859 ) ) REPRESENTATION_CONTEXT ( 'NONE', 'WORKASPACE' ) );
#136361=ORIENTED_EDGE ( 'NONE', *, *, #43324, .F. ) ;
#136363=( NAMED_UNIT ( * ) PLANE_ANGLE_UNIT ( ) SI_UNIT ( $, .RADIAN. ) );
#136365=ADVANCED_FACE ( 'NONE', ( #128466 ), #74077, .F. ) ;
#136383=CARTESIAN_POINT ( 'NONE',  ( -19.28515664589289003, 1.196650378695325090, -30.59010235425025215 ) ) ;
#136448=DIRECTION ( 'NONE',  ( 1.000000000000000000, 0.000000000000000000, 0.000000000000000000 ) ) ;
#136553=CARTESIAN_POINT ( 'NONE',  ( -7.140000000000001457, -35.14999999999999147, 17.49210858042621908 ) ) ;
#136611=DIRECTION ( 'NONE',  ( 0.000000000000000000, 2.242629915582283412E-16, -1.000000000000000000 ) ) ;
#136639=DIRECTION ( 'NONE',  ( -1.000000000000000000, 0.000000000000000000, 0.000000000000000000 ) ) ;
#136686=ORIENTED_EDGE ( 'NONE', *, *, #3276, .T. ) ;
#136691=CARTESIAN_POINT ( 'NONE',  ( -12.82211510476379956, 6.989083614815657874, -30.85058313491061099 ) ) ;
#136731=AXIS2_PLACEMENT_3D ( 'NONE', #125502, #101582, #67575 ) ;
#136765=ORIENTED_EDGE ( 'NONE', *, *, #92476, .T. ) ;
#136768=LINE ( 'NONE', #103411, #123386 ) ;
#136812=AXIS2_PLACEMENT_3D ( 'NONE', #128769, #49818, #16412 ) ;
#136814=CYLINDRICAL_SURFACE ( 'NONE', #43143, 0.5000000000000005551 ) ;
#136849=AXIS2_PLACEMENT_3D ( 'NONE', #77076, #129999, #19795 ) ;
#136853=ORIENTED_EDGE ( 'NONE', *, *, #57587, .T. ) ;
#136877=( NAMED_UNIT ( * ) PLANE_ANGLE_UNIT ( ) SI_UNIT ( $, .RADIAN. ) );
#136931=LINE ( 'NONE', #83270, #23736 ) ;
#136947=FACE_OUTER_BOUND ( 'NONE', #92975, .T. ) ;
#136983=EDGE_CURVE ( 'NONE', #59778, #32290, #53374, .T. ) ;
#136992=ORIENTED_EDGE ( 'NONE', *, *, #85715, .T. ) ;
#137008=VERTEX_POINT ( 'NONE', #98501 ) ;
#137012=SURFACE_SIDE_STYLE ('',( #125430 ) ) ;
#137045=DIRECTION ( 'NONE',  ( 0.000000000000000000, 0.000000000000000000, -1.000000000000000000 ) ) ;
#137054=PLANE ( 'NONE',  #93203 ) ;
#137062=EDGE_LOOP ( 'NONE', ( #37869, #127821, #123189, #113252, #41283, #66527, #67532, #60541, #103354, #9177, #108827, #16616 ) ) ;
#137065=MECHANICAL_DESIGN_GEOMETRIC_PRESENTATION_REPRESENTATION('',(#97620),#7478);
#137087=ORIENTED_EDGE ( 'NONE', *, *, #96700, .F. ) ;
#137152=CARTESIAN_POINT ( 'NONE',  ( -12.83997584945354831, 6.969621038081828424, -30.86176790400288539 ) ) ;
#137176=CARTESIAN_POINT ( 'NONE',  ( 7.940000000000001279, -35.14999999999999858, -10.00000000000000178 ) ) ;
#137240=( NAMED_UNIT ( * ) SI_UNIT ( $, .STERADIAN. ) SOLID_ANGLE_UNIT ( ) );
#137270=CARTESIAN_POINT ( 'NONE',  ( -7.140000000000000568, -39.92999999999999261, 19.06900128115122328 ) ) ;
#137293=DIRECTION ( 'NONE',  ( -0.000000000000000000, 6.938893903907221278E-15, -1.000000000000000000 ) ) ;
#137294=CARTESIAN_POINT ( 'NONE',  ( 12.69999999999999574, -59.76999999999998892, -39.50000000000000000 ) ) ;
#137328=UNCERTAINTY_MEASURE_WITH_UNIT (LENGTH_MEASURE( 1.000000000000000082E-05 ), #94250, 'distance_accuracy_value', 'NONE');
#137371=CARTESIAN_POINT ( 'NONE',  ( -19.05499999999999261, 3.130000000000007887, -2.396719511207313368E-16 ) ) ;
#137429=VECTOR ( 'NONE', #82517, 1000.000000000000000 ) ;
#137431=CARTESIAN_POINT ( 'NONE',  ( -11.58681024782437596, 8.220342448176232608, -30.10827610979940516 ) ) ;
#137436=CARTESIAN_POINT ( 'NONE',  ( 31.92500000000002203, -22.26999999999999247, -39.50000000000000000 ) ) ;
#137444=CYLINDRICAL_SURFACE ( 'NONE', #55134, 1.898649999999994842 ) ;
#137470=UNCERTAINTY_MEASURE_WITH_UNIT (LENGTH_MEASURE( 1.000000000000000082E-05 ), #57085, 'distance_accuracy_value', 'NONE');
#137489=ORIENTED_EDGE ( 'NONE', *, *, #79689, .T. ) ;
#137504=DIRECTION ( 'NONE',  ( -0.000000000000000000, -1.000000000000000000, -0.000000000000000000 ) ) ;
#137505=CARTESIAN_POINT ( 'NONE',  ( 12.49289321881344961, -34.94289321881345955, -40.00000000000000000 ) ) ;
#137514=VECTOR ( 'NONE', #74891, 1000.000000000000000 ) ;
#137524=VECTOR ( 'NONE', #88604, 1000.000000000000000 ) ;
#137588=ORIENTED_EDGE ( 'NONE', *, *, #79071, .T. ) ;
#137606=CYLINDRICAL_SURFACE ( 'NONE', #80658, 1.898649999999994842 ) ;
#137642=ORIENTED_EDGE ( 'NONE', *, *, #35240, .T. ) ;
#137656=EDGE_CURVE ( 'NONE', #57981, #134318, #66090, .T. ) ;
#137791=ORIENTED_EDGE ( 'NONE', *, *, #24427, .F. ) ;
#137800=CARTESIAN_POINT ( 'NONE',  ( -34.92499999999997584, 0.4299755680429860338, -27.68972139052992532 ) ) ;
#137827=CARTESIAN_POINT ( 'NONE',  ( 12.19999999999999574, -60.26999999999998892, 25.00000000000000000 ) ) ;
#137837=DIRECTION ( 'NONE',  ( -0.000000000000000000, -0.000000000000000000, -1.000000000000000000 ) ) ;
#137840=UNCERTAINTY_MEASURE_WITH_UNIT (LENGTH_MEASURE( 1.000000000000000082E-05 ), #139915, 'distance_accuracy_value', 'NONE');
#137843=VECTOR ( 'NONE', #38126, 1000.000000000000000 ) ;
#137847=CIRCLE ( 'NONE', #15078, 2.552699999999994418 ) ;
#137905=ORIENTED_EDGE ( 'NONE', *, *, #94769, .T. ) ;
#137918=CARTESIAN_POINT ( 'NONE',  ( -19.93618820135885272, -0.2700000000000093991, -36.39086428169088094 ) ) ;
#137931=SURFACE_STYLE_FILL_AREA ( #104575 ) ;
#137960=CARTESIAN_POINT ( 'NONE',  ( 0.000000000000000000, -4.870000000000014317, -10.00000000000000178 ) ) ;
#138026=VECTOR ( 'NONE', #82612, 1000.000000000000000 ) ;
#138054=ORIENTED_EDGE ( 'NONE', *, *, #49320, .F. ) ;
#138094=FILL_AREA_STYLE_COLOUR ( '', #98756 ) ;
#138139=CARTESIAN_POINT ( 'NONE',  ( -14.67277584711400351, 8.043494102545141189, -27.98791813066781131 ) ) ;
#138181=CARTESIAN_POINT ( 'NONE',  ( -7.940000000000007496, -39.92999999999999261, -12.24789999999999957 ) ) ;
#138228=VECTOR ( 'NONE', #95634, 1000.000000000000000 ) ;
#138239=AXIS2_PLACEMENT_3D ( 'NONE', #29141, #119677, #94384 ) ;
#138277=ORIENTED_EDGE ( 'NONE', *, *, #92476, .F. ) ;
#138283=PRESENTATION_STYLE_ASSIGNMENT (( #117910 ) ) ;
#138295=LINE ( 'NONE', #102819, #55853 ) ;
#138335=ADVANCED_FACE ( 'NONE', ( #83948 ), #105632, .T. ) ;
#138385=DIRECTION ( 'NONE',  ( 0.000000000000000000, -1.000000000000000000, 0.000000000000000000 ) ) ;
#138433=( GEOMETRIC_REPRESENTATION_CONTEXT ( 3 ) GLOBAL_UNCERTAINTY_ASSIGNED_CONTEXT ( ( #60659 ) ) GLOBAL_UNIT_ASSIGNED_CONTEXT ( ( #123568, #24227, #124243 ) ) REPRESENTATION_CONTEXT ( 'NONE', 'WORKASPACE' ) );
#138444=VECTOR ( 'NONE', #22528, 1000.000000000000000 ) ;
#138520=( NAMED_UNIT ( * ) SI_UNIT ( $, .STERADIAN. ) SOLID_ANGLE_UNIT ( ) );
#138529=SURFACE_STYLE_USAGE ( .BOTH. , #58884 ) ;
#138534=( GEOMETRIC_REPRESENTATION_CONTEXT ( 3 ) GLOBAL_UNCERTAINTY_ASSIGNED_CONTEXT ( ( #9955 ) ) GLOBAL_UNIT_ASSIGNED_CONTEXT ( ( #59728, #19574, #114080 ) ) REPRESENTATION_CONTEXT ( 'NONE', 'WORKASPACE' ) );
#138542=CARTESIAN_POINT ( 'NONE',  ( 1.015767586731733507, 13.72868181898487450, -24.38142353947347374 ) ) ;
#138621=LINE ( 'NONE', #59646, #40134 ) ;
#138674=FACE_OUTER_BOUND ( 'NONE', #115955, .T. ) ;
#138738=ORIENTED_EDGE ( 'NONE', *, *, #46623, .F. ) ;
#138765=DIRECTION ( 'NONE',  ( 1.000000000000000000, 3.115803279706882722E-16, -0.000000000000000000 ) ) ;
#138768=EDGE_CURVE ( 'NONE', #113921, #53394, #49599, .T. ) ;
#138769=STYLED_ITEM ( 'NONE', ( #107147 ), #47523 ) ;
#138774=VECTOR ( 'NONE', #83505, 1000.000000000000000 ) ;
#138861=CARTESIAN_POINT ( 'NONE',  ( -6.325809920431304967, 11.42897679595730231, -27.74950860237164818 ) ) ;
#138869=ORIENTED_EDGE ( 'NONE', *, *, #141052, .T. ) ;
#138873=ORIENTED_EDGE ( 'NONE', *, *, #105393, .F. ) ;
#138905=CARTESIAN_POINT ( 'NONE',  ( 7.940000000000001279, -60.26999999999998892, -10.00000000000000178 ) ) ;
#138912=DIRECTION ( 'NONE',  ( -1.000000000000000000, -1.369518533665900312E-16, 0.000000000000000000 ) ) ;
#139019=ORIENTED_EDGE ( 'NONE', *, *, #35215, .F. ) ;
#139027=ADVANCED_FACE ( 'NONE', ( #56746 ), #81330, .F. ) ;
#139074=SURFACE_SIDE_STYLE ('',( #130343 ) ) ;
#139306=AXIS2_PLACEMENT_3D ( 'NONE', #55971, #13826, #43628 ) ;
#139320=CARTESIAN_POINT ( 'NONE',  ( -4.657369210609531684, 11.96381612452156418, -27.29251722484990239 ) ) ;
#139343=ADVANCED_FACE ( 'NONE', ( #97129 ), #130538, .T. ) ;
#139398=CARTESIAN_POINT ( 'NONE',  ( -7.140000000000001457, -35.14999999999999147, -39.50000000000000000 ) ) ;
#139408=PRESENTATION_STYLE_ASSIGNMENT (( #82171 ) ) ;
#139536=PRESENTATION_STYLE_ASSIGNMENT (( #6790 ) ) ;
#139605=ORIENTED_EDGE ( 'NONE', *, *, #105266, .T. ) ;
#139647=CARTESIAN_POINT ( 'NONE',  ( -7.060677813783901691, -39.92999999999999972, 19.30339710675713150 ) ) ;
#139653=CARTESIAN_POINT ( 'NONE',  ( -12.20000000000000817, -1.670812611072399357E-15, -39.50000000000000000 ) ) ;
#139676=ORIENTED_EDGE ( 'NONE', *, *, #18717, .F. ) ;
#139691=DIRECTION ( 'NONE',  ( 0.000000000000000000, 0.000000000000000000, -1.000000000000000000 ) ) ;
#139703=EDGE_LOOP ( 'NONE', ( #73433, #126167, #138738, #98584 ) ) ;
#139742=DIRECTION ( 'NONE',  ( 0.000000000000000000, 1.000000000000000000, 0.000000000000000000 ) ) ;
#139757=ADVANCED_FACE ( 'NONE', ( #122300 ), #89008, .T. ) ;
#139775=ORIENTED_EDGE ( 'NONE', *, *, #95027, .F. ) ;
#139825=AXIS2_PLACEMENT_3D ( 'NONE', #27259, #138912, #128044 ) ;
#139828=CARTESIAN_POINT ( 'NONE',  ( -12.20000000000000462, -21.76999999999999247, -40.00000000000000000 ) ) ;
#139915=( LENGTH_UNIT ( ) NAMED_UNIT ( * ) SI_UNIT ( .MILLI., .METRE. ) );
#140007=EDGE_LOOP ( 'NONE', ( #11421, #77630, #51647, #55323 ) ) ;
#140041=SURFACE_STYLE_USAGE ( .BOTH. , #7336 ) ;
#140072=CARTESIAN_POINT ( 'NONE',  ( 34.42500000000002558, -22.26999999999999247, -0.5000000000000000000 ) ) ;
#140102=FILL_AREA_STYLE_COLOUR ( '', #38958 ) ;
#140214=ORIENTED_EDGE ( 'NONE', *, *, #107279, .T. ) ;
#140233=ORIENTED_EDGE ( 'NONE', *, *, #110454, .T. ) ;
#140240=DIRECTION ( 'NONE',  ( 1.000000000000000000, 0.000000000000000000, 0.000000000000000000 ) ) ;
#140276=CARTESIAN_POINT ( 'NONE',  ( 3.894756034733422911, 12.18018086707143866, -25.55842831757935940 ) ) ;
#140280=CARTESIAN_POINT ( 'NONE',  ( 7.139999999999985469, -39.92999999999999972, 18.93259187797431764 ) ) ;
#140338=ORIENTED_EDGE ( 'NONE', *, *, #98465, .F. ) ;
#140385=SURFACE_STYLE_FILL_AREA ( #96146 ) ;
#140396=EDGE_CURVE ( 'NONE', #2401, #25054, #67237, .T. ) ;
#140421=EDGE_LOOP ( 'NONE', ( #34030, #27488, #101028 ) ) ;
#140454=DIRECTION ( 'NONE',  ( 1.369518533665900312E-16, -1.000000000000000000, 0.000000000000000000 ) ) ;
#140511=EDGE_LOOP ( 'NONE', ( #175, #134798, #53975 ) ) ;
#140512=( NAMED_UNIT ( * ) PLANE_ANGLE_UNIT ( ) SI_UNIT ( $, .RADIAN. ) );
#140517=ORIENTED_EDGE ( 'NONE', *, *, #80806, .T. ) ;
#140551=AXIS2_PLACEMENT_3D ( 'NONE', #71016, #72465, #61576 ) ;
#140577=CARTESIAN_POINT ( 'NONE',  ( -12.20000000000000284, -25.33999999999998565, -1.334633813784589971E-30 ) ) ;
#140597=FILL_AREA_STYLE ('',( #96353 ) ) ;
#140621=ORIENTED_EDGE ( 'NONE', *, *, #73593, .F. ) ;
#140660=DIRECTION ( 'NONE',  ( -0.000000000000000000, -1.000000000000000000, -0.000000000000000000 ) ) ;
#140661=CARTESIAN_POINT ( 'NONE',  ( 12.69999999999999574, -59.76999999999998892, 24.34531699603382293 ) ) ;
#140663=PRESENTATION_STYLE_ASSIGNMENT (( #44246 ) ) ;
#140744=CARTESIAN_POINT ( 'NONE',  ( -12.70000000000000462, -28.33999999999998565, 13.17925390838734323 ) ) ;
#140794=DIRECTION ( 'NONE',  ( -1.000000000000000000, -0.000000000000000000, -0.000000000000000000 ) ) ;
#140827=( NAMED_UNIT ( * ) PLANE_ANGLE_UNIT ( ) SI_UNIT ( $, .RADIAN. ) );
#140882=VECTOR ( 'NONE', #11343, 1000.000000000000000 ) ;
#140929=CYLINDRICAL_SURFACE ( 'NONE', #126592, 0.5000000000000004441 ) ;
#140964=DIRECTION ( 'NONE',  ( -1.000000000000000000, 0.000000000000000000, 0.000000000000000000 ) ) ;
#140966=CARTESIAN_POINT ( 'NONE',  ( 6.275962415994857047, 11.42931026327849686, -27.74749330399082226 ) ) ;
#140981=VERTEX_POINT ( 'NONE', #68026 ) ;
#141027=DIRECTION ( 'NONE',  ( -0.000000000000000000, 1.000000000000000000, -0.000000000000000000 ) ) ;
#141052=EDGE_CURVE ( 'NONE', #12164, #81524, #67351, .T. ) ;
#141099=( GEOMETRIC_REPRESENTATION_CONTEXT ( 3 ) GLOBAL_UNCERTAINTY_ASSIGNED_CONTEXT ( ( #79564 ) ) GLOBAL_UNIT_ASSIGNED_CONTEXT ( ( #33390, #18891, #65292 ) ) REPRESENTATION_CONTEXT ( 'NONE', 'WORKASPACE' ) );
#141128=ORIENTED_EDGE ( 'NONE', *, *, #80069, .T. ) ;
#141160=DIRECTION ( 'NONE',  ( 0.000000000000000000, 0.000000000000000000, 1.000000000000000000 ) ) ;
#141169=FACE_OUTER_BOUND ( 'NONE', #123916, .T. ) ;
#141257=CARTESIAN_POINT ( 'NONE',  ( 12.19999999999999574, -22.33999999999998565, 0.000000000000000000 ) ) ;
#141264=CARTESIAN_POINT ( 'NONE',  ( 7.940000000000001279, -33.26999999999999602, -10.00000000000000178 ) ) ;
#141277=CARTESIAN_POINT ( 'NONE',  ( 6.932893218813447334, -34.94289321881344534, -40.00000000000000000 ) ) ;
#141288=FILL_AREA_STYLE_COLOUR ( '', #9561 ) ;
#141300=MECHANICAL_DESIGN_GEOMETRIC_PRESENTATION_REPRESENTATION('',(#4984),#55975);
#141357=CARTESIAN_POINT ( 'NONE',  ( 31.92500000000001492, 0.4299755680430057958, -27.68972139052992532 ) ) ;
#141414=CARTESIAN_POINT ( 'NONE',  ( -9.524999999999991473, -4.870000000000014317, -10.00000000000000178 ) ) ;
#141419=ORIENTED_EDGE ( 'NONE', *, *, #73941, .F. ) ;
#141427=CARTESIAN_POINT ( 'NONE',  ( 16.45742106731621135, 0.9613713492673626737, -33.49048331797055766 ) ) ;
#141458=AXIS2_PLACEMENT_3D ( 'NONE', #48691, #92895, #62436 ) ;
#141459=DIRECTION ( 'NONE',  ( -0.000000000000000000, -0.000000000000000000, 1.000000000000000000 ) ) ;
#141479=DIRECTION ( 'NONE',  ( -1.000000000000000000, -1.369518533665900312E-16, 0.000000000000000000 ) ) ;
#141518=STYLED_ITEM ( 'NONE', ( #32633 ), #72264 ) ;
#141521=VECTOR ( 'NONE', #47826, 1000.000000000000000 ) ;
#141541=AXIS2_PLACEMENT_3D ( 'NONE', #18789, #12021, #56309 ) ;
#141559=CARTESIAN_POINT ( 'NONE',  ( -19.92399413215983728, -3.162306507096367625, -35.07835588745236066 ) ) ;
#141569=AXIS2_PLACEMENT_3D ( 'NONE', #39979, #4385, #28366 ) ;
#141576=( NAMED_UNIT ( * ) SI_UNIT ( $, .STERADIAN. ) SOLID_ANGLE_UNIT ( ) );
#141646=COLOUR_RGB ( '', 0.09019608, 0.27058824, 0.51372549) ;
#141650=FILL_AREA_STYLE_COLOUR ( '', #22178 ) ;
#141658=DIRECTION ( 'NONE',  ( 0.000000000000000000, 0.000000000000000000, 1.000000000000000000 ) ) ;
#141674=CARTESIAN_POINT ( 'NONE',  ( -12.20000000000000284, -34.64999999999999147, 17.49210858042621908 ) ) ;
#141713=CARTESIAN_POINT ( 'NONE',  ( 6.851678761571759146, 12.66444798601647470, -25.17854338220229593 ) ) ;
#141758=FACE_OUTER_BOUND ( 'NONE', #52165, .T. ) ;
#141789=CARTESIAN_POINT ( 'NONE',  ( -19.93618820137057668, -3.270000000000008011, -40.00000000002046363 ) ) ;
#141839=( NAMED_UNIT ( * ) PLANE_ANGLE_UNIT ( ) SI_UNIT ( $, .RADIAN. ) );
#141893=ADVANCED_FACE ( 'NONE', ( #132926 ), #45206, .T. ) ;
#141914=EDGE_CURVE ( 'NONE', #91102, #64204, #60316, .T. ) ;
#141940=ADVANCED_FACE ( 'NONE', ( #81400 ), #92218, .F. ) ;
#141946=DIRECTION ( 'NONE',  ( 0.000000000000000000, 0.000000000000000000, -1.000000000000000000 ) ) ;
#141952=ORIENTED_EDGE ( 'NONE', *, *, #119890, .T. ) ;
#141961=FILL_AREA_STYLE_COLOUR ( '', #46166 ) ;
#141970=FACE_OUTER_BOUND ( 'NONE', #140421, .T. ) ;
#142019=ORIENTED_EDGE ( 'NONE', *, *, #72922, .F. ) ;
#142034=ORIENTED_EDGE ( 'NONE', *, *, #98719, .T. ) ;
#142035=ORIENTED_EDGE ( 'NONE', *, *, #22113, .T. ) ;
#142122=LINE ( 'NONE', #110858, #108783 ) ;
#142133=DIRECTION ( 'NONE',  ( 1.000000000000000000, 3.115803279706880257E-16, 0.000000000000000000 ) ) ;
#142135=CARTESIAN_POINT ( 'NONE',  ( 7.139999999999985469, -39.92999999999999972, -39.50000000000000000 ) ) ;
#142196=ORIENTED_EDGE ( 'NONE', *, *, #127006, .F. ) ;
#142213=DIRECTION ( 'NONE',  ( 0.000000000000000000, -1.000000000000000000, 0.000000000000000000 ) ) ;
#142234=VERTEX_POINT ( 'NONE', #98242 ) ;
#142246=FACE_OUTER_BOUND ( 'NONE', #71097, .T. ) ;
#142285=CARTESIAN_POINT ( 'NONE',  ( -19.83455468016618184, -2.420908269918533140, -33.24323018688586018 ) ) ;
#142304=COLOUR_RGB ( '', 0.09019608, 0.27058824, 0.51372549) ;
#142310=CARTESIAN_POINT ( 'NONE',  ( -7.140000000000000568, -39.92999999999998550, -39.79289321881344677 ) ) ;
#142362=CARTESIAN_POINT ( 'NONE',  ( 12.69999999999999574, -35.28159979880237529, 17.66442088362879659 ) ) ;
#142405=CIRCLE ( 'NONE', #82283, 2.247899999999996901 ) ;
#142432=CARTESIAN_POINT ( 'NONE',  ( 2.289041571428004573, 12.44546514678316029, -26.86570989468548021 ) ) ;
#142435=( LENGTH_UNIT ( ) NAMED_UNIT ( * ) SI_UNIT ( .MILLI., .METRE. ) );
#142436=DIRECTION ( 'NONE',  ( 1.000000000000000000, -0.000000000000000000, 0.000000000000000000 ) ) ;
#142440=CARTESIAN_POINT ( 'NONE',  ( 7.940000000000001279, -33.26999999999999602, -8.101350000000008933 ) ) ;
#142458=LINE ( 'NONE', #3003, #21119 ) ;
#142469=MANIFOLD_SOLID_BREP ( 'Fillet6', #78794 ) ;
#142559=ADVANCED_FACE ( 'NONE', ( #31971 ), #97946, .T. ) ;
#142621=SURFACE_SIDE_STYLE ('',( #120108 ) ) ;
#142686=( NAMED_UNIT ( * ) SI_UNIT ( $, .STERADIAN. ) SOLID_ANGLE_UNIT ( ) );
#142765=VECTOR ( 'NONE', #44727, 1000.000000000000114 ) ;
#142780=CIRCLE ( 'NONE', #50190, 0.5000000000000004441 ) ;
#142782=FILL_AREA_STYLE_COLOUR ( '', #90712 ) ;
#142802=( NAMED_UNIT ( * ) SI_UNIT ( $, .STERADIAN. ) SOLID_ANGLE_UNIT ( ) );
#142824=CARTESIAN_POINT ( 'NONE',  ( 31.92500000000001492, 9.947201970464227326E-15, -37.00000000000000000 ) ) ;
#142854=CARTESIAN_POINT ( 'NONE',  ( 6.342232970832937688, 11.40363289190650065, -27.76885313926799626 ) ) ;
#142872=PRESENTATION_STYLE_ASSIGNMENT (( #131285 ) ) ;
#142981=CARTESIAN_POINT ( 'NONE',  ( 12.19999999999999574, 0.000000000000000000, -40.00000000000000000 ) ) ;
#142985=DIRECTION ( 'NONE',  ( 1.369518533665900312E-16, -1.000000000000000000, 0.000000000000000000 ) ) ;
#142998=CARTESIAN_POINT ( 'NONE',  ( -7.940000000000007496, -60.26999999999998892, -10.00000000000000178 ) ) ;
#143055=DIRECTION ( 'NONE',  ( -1.000000000000000000, 0.000000000000000000, 0.000000000000000000 ) ) ;
#143124=CARTESIAN_POINT ( 'NONE',  ( -2.205225646411241414, 13.66209448022662443, -24.43382165111117033 ) ) ;
#143128=FILL_AREA_STYLE ('',( #130857 ) ) ;
#143240=VERTEX_POINT ( 'NONE', #94712 ) ;
#143284=ORIENTED_EDGE ( 'NONE', *, *, #9786, .T. ) ;
#143319=AXIS2_PLACEMENT_3D ( 'NONE', #133325, #22367, #90524 ) ;
#143337=DIRECTION ( 'NONE',  ( 1.000000000000000000, 0.000000000000000000, 0.000000000000000000 ) ) ;
#143366=ADVANCED_FACE ( 'NONE', ( #10563 ), #53373, .T. ) ;
#143376=ADVANCED_FACE ( 'NONE', ( #36613 ), #89374, .F. ) ;
#143393=DIRECTION ( 'NONE',  ( 0.000000000000000000, -2.242629915582283412E-16, 1.000000000000000000 ) ) ;
#143415=AXIS2_PLACEMENT_3D ( 'NONE', #20491, #9615, #150 ) ;
#143465=LINE ( 'NONE', #77539, #107343 ) ;
#143487=CARTESIAN_POINT ( 'NONE',  ( -34.92499999999999005, 2.729999999999986215, -36.39086428169088094 ) ) ;
#143489=VECTOR ( 'NONE', #91625, 999.9999999999998863 ) ;
#143506=ADVANCED_FACE ( 'NONE', ( #48214 ), #67672, .T. ) ;
#143510=SURFACE_STYLE_USAGE ( .BOTH. , #46391 ) ;
#143526=CIRCLE ( 'NONE', #81049, 0.5000000000000004441 ) ;
ENDSEC;
END-ISO-10303-21;
